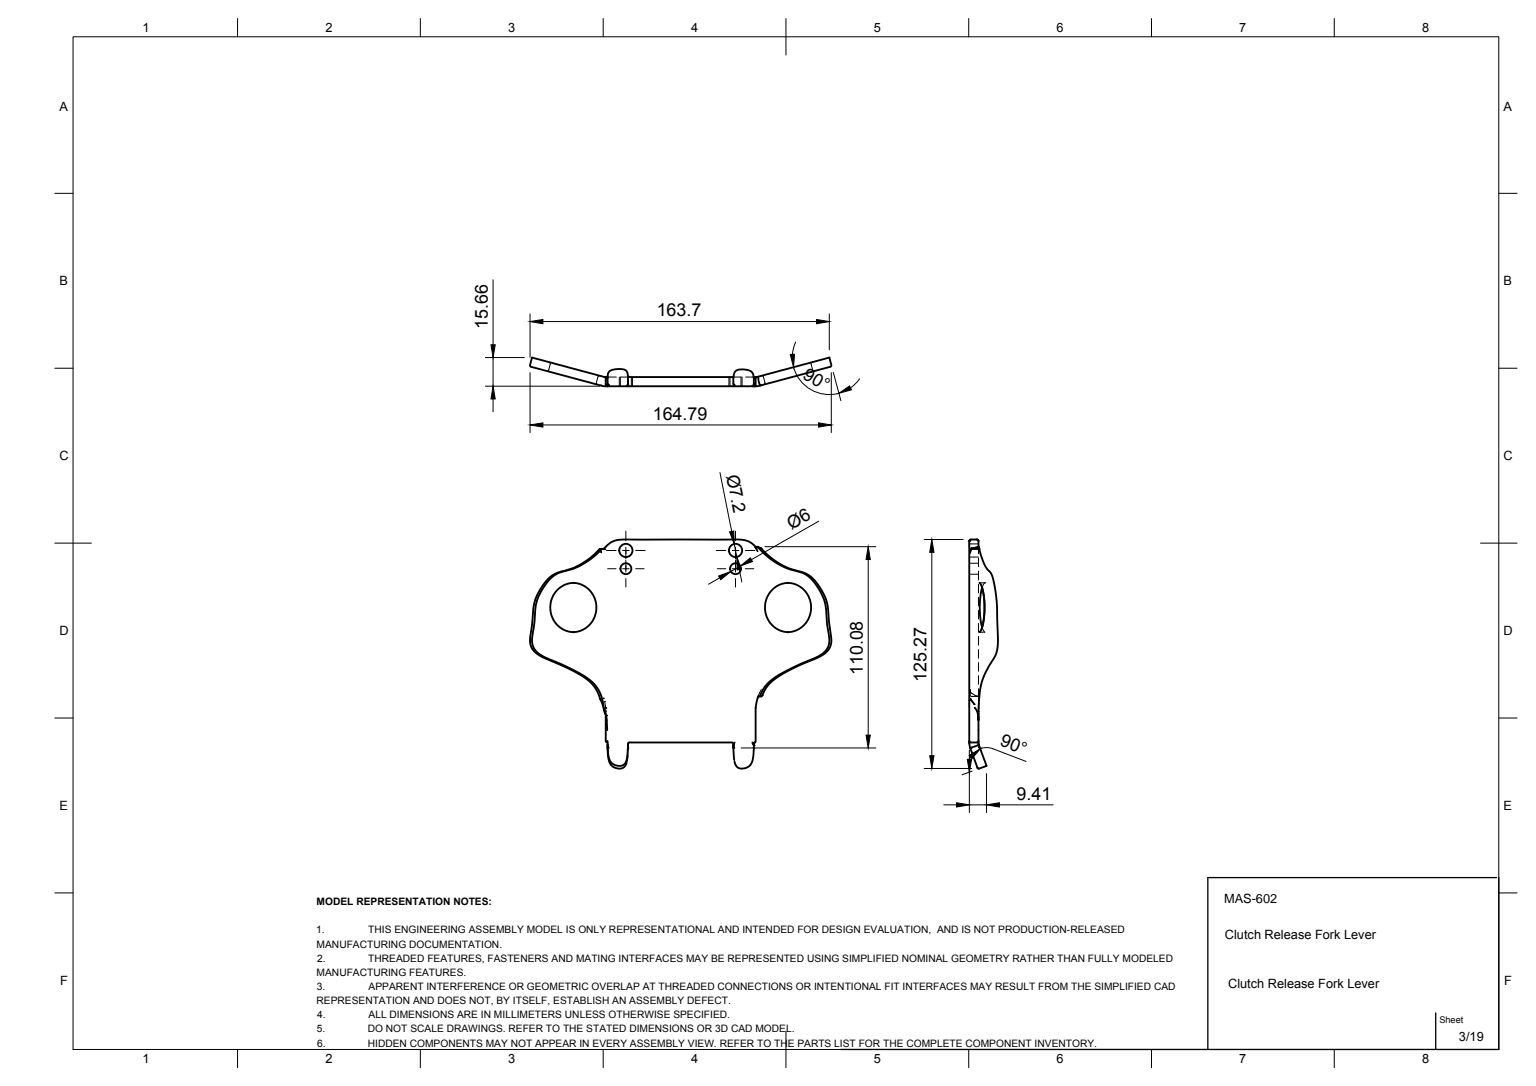
ISO-10303-21;
HEADER;
/* Generated by software containing ST-Developer
 * from STEP Tools, Inc. (www.steptools.com) 
 */

FILE_DESCRIPTION(
/* description */ (''),
/* implementation_level */ '2;1');

FILE_NAME(
/* name */ 'Clutch Release Fork Lever.step',
/* time_stamp */ '2026-10-15T14:42:47-07:00',
/* author */ (''),
/* organization */ (''),
/* preprocessor_version */ 'ST-DEVELOPER v20.2',
/* originating_system */ 'Autodesk Translation Framework v15.15.0.0',
/* authorisation */ '');

FILE_SCHEMA (('AUTOMOTIVE_DESIGN { 1 0 10303 214 3 1 1 }'));
ENDSEC;

DATA;
#10=MECHANICAL_DESIGN_GEOMETRIC_PRESENTATION_REPRESENTATION('',(#234),#85789);
#198=SHAPE_REPRESENTATION_RELATIONSHIP('SRR','None',#85863,#216);
#216=ADVANCED_BREP_SHAPE_REPRESENTATION('',(#252),#85771);
#234=STYLED_ITEM('',(#85962),#252);
#252=MANIFOLD_SOLID_BREP('Body1',#9881);
#270=SPHERICAL_SURFACE('',#10130,0.08);
#271=SPHERICAL_SURFACE('',#10138,0.08);
#272=SPHERICAL_SURFACE('',#10178,0.08);
#273=SPHERICAL_SURFACE('',#10200,0.08);
#274=SPHERICAL_SURFACE('',#10239,0.08);
#275=SPHERICAL_SURFACE('',#10241,0.08);
#276=SPHERICAL_SURFACE('',#10260,0.08);
#277=SPHERICAL_SURFACE('',#10282,0.08);
#278=SPHERICAL_SURFACE('',#10292,0.08);
#280=B_SPLINE_SURFACE_WITH_KNOTS('',3,1,((#13627,#13628),(#13629,#13630),
(#13631,#13632),(#13633,#13634),(#13635,#13636),(#13637,#13638),(#13639,
#13640)),.UNSPECIFIED.,.F.,.F.,.F.,(4,1,1,1,4),(2,2),(0.,0.285714285714286,
0.571428571428571,0.785714285714286,1.),(0.,0.504000000000458),
 .UNSPECIFIED.);
#281=B_SPLINE_SURFACE_WITH_KNOTS('',5,1,((#13700,#13701),(#13702,#13703),
(#13704,#13705),(#13706,#13707),(#13708,#13709),(#13710,#13711),(#13712,
#13713),(#13714,#13715),(#13716,#13717),(#13718,#13719),(#13720,#13721),
(#13722,#13723),(#13724,#13725),(#13726,#13727),(#13728,#13729),(#13730,
#13731),(#13732,#13733),(#13734,#13735),(#13736,#13737),(#13738,#13739),
(#13740,#13741),(#13742,#13743),(#13744,#13745),(#13746,#13747),(#13748,
#13749),(#13750,#13751),(#13752,#13753),(#13754,#13755),(#13756,#13757),
(#13758,#13759),(#13760,#13761),(#13762,#13763),(#13764,#13765),(#13766,
#13767),(#13768,#13769),(#13770,#13771),(#13772,#13773),(#13774,#13775),
(#13776,#13777),(#13778,#13779),(#13780,#13781),(#13782,#13783),(#13784,
#13785),(#13786,#13787),(#13788,#13789),(#13790,#13791),(#13792,#13793),
(#13794,#13795),(#13796,#13797),(#13798,#13799),(#13800,#13801),(#13802,
#13803),(#13804,#13805),(#13806,#13807),(#13808,#13809),(#13810,#13811),
(#13812,#13813),(#13814,#13815),(#13816,#13817),(#13818,#13819),(#13820,
#13821),(#13822,#13823),(#13824,#13825),(#13826,#13827),(#13828,#13829),
(#13830,#13831),(#13832,#13833),(#13834,#13835),(#13836,#13837),(#13838,
#13839),(#13840,#13841),(#13842,#13843),(#13844,#13845),(#13846,#13847),
(#13848,#13849),(#13850,#13851),(#13852,#13853),(#13854,#13855),(#13856,
#13857),(#13858,#13859),(#13860,#13861),(#13862,#13863),(#13864,#13865),
(#13866,#13867),(#13868,#13869),(#13870,#13871),(#13872,#13873),(#13874,
#13875),(#13876,#13877),(#13878,#13879),(#13880,#13881),(#13882,#13883),
(#13884,#13885),(#13886,#13887),(#13888,#13889),(#13890,#13891),(#13892,
#13893),(#13894,#13895),(#13896,#13897),(#13898,#13899),(#13900,#13901),
(#13902,#13903),(#13904,#13905),(#13906,#13907),(#13908,#13909),(#13910,
#13911),(#13912,#13913),(#13914,#13915),(#13916,#13917),(#13918,#13919),
(#13920,#13921),(#13922,#13923),(#13924,#13925),(#13926,#13927),(#13928,
#13929),(#13930,#13931),(#13932,#13933),(#13934,#13935),(#13936,#13937),
(#13938,#13939),(#13940,#13941),(#13942,#13943),(#13944,#13945),(#13946,
#13947),(#13948,#13949),(#13950,#13951),(#13952,#13953),(#13954,#13955),
(#13956,#13957),(#13958,#13959),(#13960,#13961),(#13962,#13963),(#13964,
#13965),(#13966,#13967),(#13968,#13969),(#13970,#13971),(#13972,#13973),
(#13974,#13975),(#13976,#13977),(#13978,#13979),(#13980,#13981),(#13982,
#13983),(#13984,#13985),(#13986,#13987),(#13988,#13989),(#13990,#13991),
(#13992,#13993),(#13994,#13995),(#13996,#13997),(#13998,#13999),(#14000,
#14001),(#14002,#14003),(#14004,#14005),(#14006,#14007),(#14008,#14009),
(#14010,#14011),(#14012,#14013),(#14014,#14015),(#14016,#14017),(#14018,
#14019),(#14020,#14021),(#14022,#14023),(#14024,#14025),(#14026,#14027),
(#14028,#14029),(#14030,#14031),(#14032,#14033),(#14034,#14035),(#14036,
#14037),(#14038,#14039),(#14040,#14041),(#14042,#14043),(#14044,#14045),
(#14046,#14047),(#14048,#14049),(#14050,#14051),(#14052,#14053),(#14054,
#14055),(#14056,#14057),(#14058,#14059),(#14060,#14061),(#14062,#14063),
(#14064,#14065),(#14066,#14067),(#14068,#14069),(#14070,#14071),(#14072,
#14073),(#14074,#14075),(#14076,#14077),(#14078,#14079),(#14080,#14081),
(#14082,#14083),(#14084,#14085),(#14086,#14087),(#14088,#14089),(#14090,
#14091),(#14092,#14093),(#14094,#14095),(#14096,#14097),(#14098,#14099),
(#14100,#14101),(#14102,#14103),(#14104,#14105),(#14106,#14107),(#14108,
#14109),(#14110,#14111),(#14112,#14113),(#14114,#14115),(#14116,#14117),
(#14118,#14119),(#14120,#14121),(#14122,#14123),(#14124,#14125),(#14126,
#14127),(#14128,#14129),(#14130,#14131),(#14132,#14133),(#14134,#14135),
(#14136,#14137),(#14138,#14139),(#14140,#14141),(#14142,#14143),(#14144,
#14145),(#14146,#14147),(#14148,#14149),(#14150,#14151),(#14152,#14153),
(#14154,#14155),(#14156,#14157),(#14158,#14159),(#14160,#14161),(#14162,
#14163),(#14164,#14165),(#14166,#14167),(#14168,#14169),(#14170,#14171),
(#14172,#14173),(#14174,#14175),(#14176,#14177),(#14178,#14179),(#14180,
#14181),(#14182,#14183),(#14184,#14185),(#14186,#14187),(#14188,#14189),
(#14190,#14191),(#14192,#14193),(#14194,#14195),(#14196,#14197),(#14198,
#14199),(#14200,#14201),(#14202,#14203),(#14204,#14205),(#14206,#14207),
(#14208,#14209),(#14210,#14211),(#14212,#14213),(#14214,#14215),(#14216,
#14217),(#14218,#14219)),.UNSPECIFIED.,.T.,.F.,.F.,(6,1,1,1,1,1,1,1,1,1,
1,1,1,1,1,1,1,1,1,1,1,1,1,1,1,1,1,1,1,1,1,1,1,1,1,1,1,1,1,1,1,1,1,1,1,1,
1,1,1,1,1,1,1,1,1,1,1,1,1,1,1,1,1,1,1,1,1,1,1,1,1,1,1,1,1,1,1,1,1,1,5,1,
1,1,1,1,1,1,1,1,1,1,1,1,1,1,1,1,1,1,1,1,1,1,1,1,1,1,1,1,1,1,1,1,1,1,1,1,
1,1,1,1,1,1,1,1,1,1,1,1,1,1,1,1,1,1,1,1,1,1,1,1,1,1,1,1,1,1,1,1,1,1,1,1,
1,1,1,1,1,1,1,1,1,1,1,1,1,1,1,1,1,1,1,1,1,1,1,1,1,1,1,1,1,1,1,1,1,1,1,1,
1,1,1,1,1,1,1,1,1,1,1,1,1,1,1,1,1,1,1,1,1,1,1,1,1,1,1,1,1,1,1,1,1,1,1,1,
1,1,1,1,1,1,1,1,1,1,1,1,1,1,1,1,1,1,1,1,1,1,1,1,1,6),(2,2),(-0.318438690804418,
-0.316,-0.312,-0.308,-0.304,-0.3,-0.296,-0.292,-0.288,-0.284,-0.28,-0.276,
-0.272,-0.268,-0.264,-0.26,-0.256,-0.252,-0.248,-0.244,-0.24,-0.236,-0.232,
-0.228,-0.224,-0.22,-0.216,-0.212,-0.208,-0.204,-0.2,-0.196,-0.192,-0.188,
-0.184,-0.18,-0.176,-0.172,-0.168,-0.164,-0.16,-0.156,-0.152,-0.148,-0.144,
-0.14,-0.136,-0.132,-0.128,-0.124,-0.12,-0.116,-0.112,-0.108,-0.104,-0.1,
-0.0960000000000001,-0.0920000000000001,-0.0880000000000001,-0.084,-0.08,
-0.076,-0.072,-0.068,-0.064,-0.06,-0.056,-0.052,-0.048,-0.044,-0.04,-0.036,
-0.032,-0.028,-0.024,-0.02,-0.016,-0.012,-0.008,-0.004,0.,0.00399999999999923,
0.00799999999999923,0.0119999999999992,0.0159999999999992,0.0199999999999992,
0.0239999999999992,0.0279999999999992,0.0319999999999993,0.0359999999999993,
0.0399999999999993,0.0439999999999993,0.0479999999999993,0.0519999999999993,
0.0559999999999993,0.0599999999999993,0.0639999999999993,0.0679999999999993,
0.0719999999999993,0.0759999999999993,0.0799999999999993,0.0839999999999993,
0.0879999999999993,0.0919999999999993,0.0959999999999993,0.0999999999999993,
0.103999999999999,0.107999999999999,0.111999999999999,0.115999999999999,
0.119999999999999,0.123999999999999,0.127999999999999,0.131999999999999,
0.135999999999999,0.139999999999999,0.143999999999999,0.147999999999999,
0.151999999999999,0.155999999999999,0.159999999999999,0.163999999999999,
0.167999999999999,0.171999999999999,0.175999999999999,0.179999999999999,
0.183999999999999,0.187999999999999,0.191999999999999,0.195999999999999,
0.199999999999999,0.203999999999999,0.207999999999999,0.211999999999999,
0.215999999999999,0.219999999999999,0.223999999999999,0.227999999999999,
0.231999999999999,0.235999999999999,0.239999999999999,0.243999999999999,
0.247999999999999,0.251999999999999,0.255999999999999,0.259999999999999,
0.263999999999999,0.267999999999999,0.271999999999999,0.275999999999999,
0.279999999999999,0.283999999999999,0.287999999999999,0.291999999999999,
0.295999999999999,0.299999999999999,0.303999999999999,0.307999999999999,
0.311999999999999,0.316,0.32,0.324,0.328,0.332,0.336,0.34,0.344,0.348,0.352,
0.356,0.36,0.364,0.368,0.372,0.376,0.38,0.384,0.388,0.392,0.396,0.4,0.404,
0.408,0.412,0.416,0.42,0.424,0.428,0.432,0.436,0.44,0.444,0.448,0.452,0.456,
0.46,0.464,0.468,0.472,0.476,0.48,0.484,0.488,0.492,0.496,0.5,0.504,0.508,
0.512,0.516,0.52,0.524,0.528,0.532,0.536,0.54,0.544,0.548,0.552,0.556,0.56,
0.564,0.568,0.572,0.576,0.58,0.584,0.588,0.592,0.596,0.6,0.604,0.608,0.612,
0.616,0.62,0.624,0.628,0.632,0.636,0.64,0.644,0.648,0.652,0.656,0.66,0.664,
0.668,0.672,0.676,0.68,0.681561309195582),(0.,2.17767906516806),
 .UNSPECIFIED.);
#282=B_SPLINE_SURFACE_WITH_KNOTS('',3,3,((#14275,#14276,#14277,#14278,#14279,
#14280,#14281,#14282,#14283,#14284,#14285,#14286,#14287,#14288,#14289,#14290,
#14291,#14292,#14293,#14294,#14295,#14296,#14297,#14298,#14299,#14300,#14301,
#14302,#14303,#14304,#14305,#14306,#14307,#14308,#14309),(#14310,#14311,
#14312,#14313,#14314,#14315,#14316,#14317,#14318,#14319,#14320,#14321,#14322,
#14323,#14324,#14325,#14326,#14327,#14328,#14329,#14330,#14331,#14332,#14333,
#14334,#14335,#14336,#14337,#14338,#14339,#14340,#14341,#14342,#14343,#14344),
(#14345,#14346,#14347,#14348,#14349,#14350,#14351,#14352,#14353,#14354,
#14355,#14356,#14357,#14358,#14359,#14360,#14361,#14362,#14363,#14364,#14365,
#14366,#14367,#14368,#14369,#14370,#14371,#14372,#14373,#14374,#14375,#14376,
#14377,#14378,#14379),(#14380,#14381,#14382,#14383,#14384,#14385,#14386,
#14387,#14388,#14389,#14390,#14391,#14392,#14393,#14394,#14395,#14396,#14397,
#14398,#14399,#14400,#14401,#14402,#14403,#14404,#14405,#14406,#14407,#14408,
#14409,#14410,#14411,#14412,#14413,#14414),(#14415,#14416,#14417,#14418,
#14419,#14420,#14421,#14422,#14423,#14424,#14425,#14426,#14427,#14428,#14429,
#14430,#14431,#14432,#14433,#14434,#14435,#14436,#14437,#14438,#14439,#14440,
#14441,#14442,#14443,#14444,#14445,#14446,#14447,#14448,#14449)),
 .UNSPECIFIED.,.F.,.F.,.F.,(4,1,4),(4,1,1,1,1,1,1,1,1,1,1,1,1,1,1,1,1,1,
1,1,1,1,1,1,1,1,1,1,1,1,1,1,4),(0.,0.571428571428571,1.),(0.,0.433353360299055,
0.866706720598111,1.30006008089717,1.73341344119622,2.16676680149528,2.49178182171957,
2.60012016179433,3.03347352209339,3.25015020224292,3.46682688239244,4.04463136279118,
4.62243584318992,4.91133808338929,5.20024032358866,5.77804480398741,6.06694704418677,
6.35584928438614,6.64475152458552,6.93365376478489,7.22255600498426,7.36700712508394,
7.51145824518363,7.65590936528331,7.800360485383,8.08926272558237,8.66706720598111,
9.24487168637985,9.82267616677859,10.4004806471773,11.2671873677754,11.7005407280745,
12.1338940883735),.UNSPECIFIED.);
#283=B_SPLINE_SURFACE_WITH_KNOTS('',3,3,((#14451,#14452,#14453,#14454,#14455,
#14456),(#14457,#14458,#14459,#14460,#14461,#14462),(#14463,#14464,#14465,
#14466,#14467,#14468),(#14469,#14470,#14471,#14472,#14473,#14474)),
 .UNSPECIFIED.,.F.,.F.,.F.,(4,4),(4,2,4),(-0.0537574666271907,1.),(-0.15340523472588,
-0.152867184867239,-0.0444303035234761),.UNSPECIFIED.);
#284=B_SPLINE_SURFACE_WITH_KNOTS('',3,3,((#14503,#14504,#14505,#14506),
(#14507,#14508,#14509,#14510),(#14511,#14512,#14513,#14514),(#14515,#14516,
#14517,#14518),(#14519,#14520,#14521,#14522)),.UNSPECIFIED.,.F.,.F.,.F.,
(4,1,4),(4,4),(0.,0.571428571428571,1.),(0.,0.0543233651499556),
 .UNSPECIFIED.);
#285=B_SPLINE_SURFACE_WITH_KNOTS('',3,3,((#14540,#14541,#14542,#14543,#14544,
#14545,#14546,#14547),(#14548,#14549,#14550,#14551,#14552,#14553,#14554,
#14555),(#14556,#14557,#14558,#14559,#14560,#14561,#14562,#14563),(#14564,
#14565,#14566,#14567,#14568,#14569,#14570,#14571),(#14572,#14573,#14574,
#14575,#14576,#14577,#14578,#14579),(#14580,#14581,#14582,#14583,#14584,
#14585,#14586,#14587)),.UNSPECIFIED.,.F.,.F.,.F.,(4,1,1,4),(4,1,1,1,1,4),
(0.,0.285714285714286,0.571428571428571,1.),(0.0937174606900304,0.104785099917186,
0.112163526068624,0.115852739144342,0.117697345682202,0.119541952220061),
 .UNSPECIFIED.);
#286=B_SPLINE_SURFACE_WITH_KNOTS('',3,3,((#14598,#14599,#14600,#14601,#14602,
#14603),(#14604,#14605,#14606,#14607,#14608,#14609),(#14610,#14611,#14612,
#14613,#14614,#14615),(#14616,#14617,#14618,#14619,#14620,#14621),(#14622,
#14623,#14624,#14625,#14626,#14627)),.UNSPECIFIED.,.F.,.F.,.F.,(4,1,4),
(4,1,1,4),(0.362133804475251,0.635505031128715,1.),(1.65498255800438E-15,
0.129082836972258,0.215138061620429,0.3011932862686),.UNSPECIFIED.);
#287=B_SPLINE_SURFACE_WITH_KNOTS('',3,3,((#14636,#14637,#14638,#14639),
(#14640,#14641,#14642,#14643),(#14644,#14645,#14646,#14647),(#14648,#14649,
#14650,#14651),(#14652,#14653,#14654,#14655)),.UNSPECIFIED.,.F.,.F.,.F.,
(4,1,4),(4,4),(-3.21642455285252E-5,0.5,1.),(-3.21642455285252E-5,0.22768259721804),
 .UNSPECIFIED.);
#288=B_SPLINE_SURFACE_WITH_KNOTS('',3,3,((#14667,#14668,#14669,#14670),
(#14671,#14672,#14673,#14674),(#14675,#14676,#14677,#14678),(#14679,#14680,
#14681,#14682),(#14683,#14684,#14685,#14686)),.UNSPECIFIED.,.F.,.F.,.F.,
(4,1,4),(4,4),(0.,0.5,1.),(6.03465648009666E-14,0.0429068684110201),
 .UNSPECIFIED.);
#289=B_SPLINE_SURFACE_WITH_KNOTS('',3,3,((#14693,#14694,#14695,#14696),
(#14697,#14698,#14699,#14700),(#14701,#14702,#14703,#14704),(#14705,#14706,
#14707,#14708),(#14709,#14710,#14711,#14712)),.UNSPECIFIED.,.F.,.F.,.F.,
(4,1,4),(4,4),(0.,0.571428571428571,1.),(0.,0.0979595230969147),
 .UNSPECIFIED.);
#290=B_SPLINE_SURFACE_WITH_KNOTS('',3,3,((#14714,#14715,#14716,#14717),
(#14718,#14719,#14720,#14721),(#14722,#14723,#14724,#14725),(#14726,#14727,
#14728,#14729),(#14730,#14731,#14732,#14733)),.UNSPECIFIED.,.F.,.F.,.F.,
(4,1,4),(4,4),(0.,0.5,1.),(0.101309492239901,0.150948832556605),
 .UNSPECIFIED.);
#291=B_SPLINE_SURFACE_WITH_KNOTS('',3,3,((#14774,#14775,#14776,#14777),
(#14778,#14779,#14780,#14781),(#14782,#14783,#14784,#14785),(#14786,#14787,
#14788,#14789),(#14790,#14791,#14792,#14793)),.UNSPECIFIED.,.F.,.F.,.F.,
(4,1,4),(4,4),(0.362133804475334,0.726628773346571,1.),(0.,0.0965340005117894),
 .UNSPECIFIED.);
#292=B_SPLINE_SURFACE_WITH_KNOTS('',3,3,((#14829,#14830,#14831,#14832),
(#14833,#14834,#14835,#14836),(#14837,#14838,#14839,#14840),(#14841,#14842,
#14843,#14844),(#14845,#14846,#14847,#14848)),.UNSPECIFIED.,.F.,.F.,.F.,
(4,1,4),(4,4),(0.40963181845835,0.704815909229175,1.),(0.,0.224615521635083),
 .UNSPECIFIED.);
#293=B_SPLINE_SURFACE_WITH_KNOTS('',3,3,((#14855,#14856,#14857,#14858),
(#14859,#14860,#14861,#14862),(#14863,#14864,#14865,#14866),(#14867,#14868,
#14869,#14870),(#14871,#14872,#14873,#14874)),.UNSPECIFIED.,.F.,.F.,.F.,
(4,1,4),(4,4),(0.,0.23767239441161,0.47534478882322),(0.0854459382956349,
0.127798241063314),.UNSPECIFIED.);
#294=B_SPLINE_SURFACE_WITH_KNOTS('',3,3,((#14881,#14882,#14883,#14884,#14885,
#14886,#14887),(#14888,#14889,#14890,#14891,#14892,#14893,#14894),(#14895,
#14896,#14897,#14898,#14899,#14900,#14901),(#14902,#14903,#14904,#14905,
#14906,#14907,#14908),(#14909,#14910,#14911,#14912,#14913,#14914,#14915),
(#14916,#14917,#14918,#14919,#14920,#14921,#14922)),.UNSPECIFIED.,.F.,.F.,
 .F.,(4,1,1,4),(4,1,1,1,4),(0.283162399774082,0.590378514156618,0.795189257078309,
1.),(0.,0.0328013253035665,0.065602650607133,0.109337751011888,0.153072851416644),
 .UNSPECIFIED.);
#295=B_SPLINE_SURFACE_WITH_KNOTS('',3,3,((#14931,#14932,#14933,#14934),
(#14935,#14936,#14937,#14938),(#14939,#14940,#14941,#14942),(#14943,#14944,
#14945,#14946),(#14947,#14948,#14949,#14950)),.UNSPECIFIED.,.F.,.F.,.F.,
(4,1,4),(4,4),(0.44925085787876,0.702584769501779,0.955918681124799),(0.,
0.0419417607304844),.UNSPECIFIED.);
#296=B_SPLINE_SURFACE_WITH_KNOTS('',3,3,((#14951,#14952,#14953,#14954),
(#14955,#14956,#14957,#14958),(#14959,#14960,#14961,#14962),(#14963,#14964,
#14965,#14966)),.UNSPECIFIED.,.F.,.F.,.F.,(4,4),(4,4),(0.,0.279727981322212),
(0.,0.17884239607127),.UNSPECIFIED.);
#297=B_SPLINE_SURFACE_WITH_KNOTS('',3,3,((#14973,#14974,#14975,#14976),
(#14977,#14978,#14979,#14980),(#14981,#14982,#14983,#14984),(#14985,#14986,
#14987,#14988)),.UNSPECIFIED.,.F.,.F.,.F.,(4,4),(4,4),(0.547578918945948,
1.),(0.,0.0801298062963358),.UNSPECIFIED.);
#298=B_SPLINE_SURFACE_WITH_KNOTS('',3,3,((#14995,#14996,#14997,#14998,#14999,
#15000,#15001,#15002,#15003,#15004,#15005,#15006,#15007,#15008,#15009,#15010,
#15011,#15012,#15013,#15014,#15015),(#15016,#15017,#15018,#15019,#15020,
#15021,#15022,#15023,#15024,#15025,#15026,#15027,#15028,#15029,#15030,#15031,
#15032,#15033,#15034,#15035,#15036),(#15037,#15038,#15039,#15040,#15041,
#15042,#15043,#15044,#15045,#15046,#15047,#15048,#15049,#15050,#15051,#15052,
#15053,#15054,#15055,#15056,#15057),(#15058,#15059,#15060,#15061,#15062,
#15063,#15064,#15065,#15066,#15067,#15068,#15069,#15070,#15071,#15072,#15073,
#15074,#15075,#15076,#15077,#15078),(#15079,#15080,#15081,#15082,#15083,
#15084,#15085,#15086,#15087,#15088,#15089,#15090,#15091,#15092,#15093,#15094,
#15095,#15096,#15097,#15098,#15099)),.UNSPECIFIED.,.F.,.F.,.F.,(4,1,4),
(4,1,1,1,1,1,1,1,1,1,1,1,1,1,1,1,1,1,4),(0.,0.571428571428571,1.),(0.,0.148302061038192,
0.296604122076384,0.444906183114576,0.593208244152767,0.889812366229151,
1.18641648830553,1.7796247324583,2.37283297661107,4.74566595322214,5.93208244152767,
6.52529068568044,7.11849892983321,7.41510305190959,7.71170717398598,7.86000923502417,
8.00831129606236,8.15661335710055,8.30491541813874),.UNSPECIFIED.);
#299=B_SPLINE_SURFACE_WITH_KNOTS('',5,1,((#15347,#15348),(#15349,#15350),
(#15351,#15352),(#15353,#15354),(#15355,#15356),(#15357,#15358),(#15359,
#15360),(#15361,#15362),(#15363,#15364),(#15365,#15366),(#15367,#15368),
(#15369,#15370),(#15371,#15372),(#15373,#15374),(#15375,#15376),(#15377,
#15378),(#15379,#15380),(#15381,#15382),(#15383,#15384),(#15385,#15386),
(#15387,#15388),(#15389,#15390),(#15391,#15392),(#15393,#15394),(#15395,
#15396),(#15397,#15398),(#15399,#15400),(#15401,#15402),(#15403,#15404),
(#15405,#15406),(#15407,#15408),(#15409,#15410),(#15411,#15412),(#15413,
#15414),(#15415,#15416),(#15417,#15418),(#15419,#15420),(#15421,#15422),
(#15423,#15424),(#15425,#15426),(#15427,#15428)),.UNSPECIFIED.,.F.,.F.,
 .F.,(6,1,1,1,1,1,1,1,1,1,1,1,1,1,1,1,5,1,1,1,1,1,1,1,1,1,1,1,1,1,1,1,6),
(2,2),(-1.06140995878253,-1.06,-1.056,-1.052,-1.048,-1.044,-1.04,-1.036,
-1.032,-1.028,-1.024,-1.02,-1.016,-1.012,-1.008,-1.004,-1.,-0.996000000000001,
-0.992000000000001,-0.988000000000001,-0.984000000000001,-0.980000000000001,
-0.976000000000001,-0.972000000000001,-0.968000000000001,-0.964000000000001,
-0.960000000000001,-0.956000000000001,-0.952000000000001,-0.948000000000001,
-0.944000000000001,-0.940000000000001,-0.938590041217474),(0.,0.6),
 .UNSPECIFIED.);
#300=B_SPLINE_SURFACE_WITH_KNOTS('',5,1,((#15656,#15657),(#15658,#15659),
(#15660,#15661),(#15662,#15663),(#15664,#15665),(#15666,#15667),(#15668,
#15669),(#15670,#15671),(#15672,#15673),(#15674,#15675),(#15676,#15677),
(#15678,#15679),(#15680,#15681),(#15682,#15683),(#15684,#15685),(#15686,
#15687),(#15688,#15689),(#15690,#15691),(#15692,#15693),(#15694,#15695),
(#15696,#15697),(#15698,#15699),(#15700,#15701),(#15702,#15703),(#15704,
#15705),(#15706,#15707),(#15708,#15709),(#15710,#15711),(#15712,#15713),
(#15714,#15715),(#15716,#15717),(#15718,#15719),(#15720,#15721),(#15722,
#15723),(#15724,#15725),(#15726,#15727),(#15728,#15729),(#15730,#15731),
(#15732,#15733),(#15734,#15735),(#15736,#15737),(#15738,#15739),(#15740,
#15741),(#15742,#15743),(#15744,#15745),(#15746,#15747),(#15748,#15749),
(#15750,#15751),(#15752,#15753),(#15754,#15755),(#15756,#15757),(#15758,
#15759),(#15760,#15761),(#15762,#15763),(#15764,#15765),(#15766,#15767),
(#15768,#15769),(#15770,#15771),(#15772,#15773),(#15774,#15775),(#15776,
#15777),(#15778,#15779),(#15780,#15781),(#15782,#15783),(#15784,#15785),
(#15786,#15787),(#15788,#15789),(#15790,#15791),(#15792,#15793),(#15794,
#15795)),.UNSPECIFIED.,.F.,.F.,.F.,(6,1,1,1,1,1,1,1,1,1,1,1,1,1,1,1,1,1,
1,1,1,1,1,1,1,1,1,1,1,1,1,1,1,1,1,1,1,1,1,1,1,1,1,1,1,1,1,1,1,1,1,1,1,1,
1,1,1,1,1,1,1,1,1,1,1,6),(2,2),(-0.318438690804418,-0.316,-0.312,-0.308,
-0.304,-0.3,-0.296,-0.292,-0.288,-0.284,-0.28,-0.276,-0.272,-0.268,-0.264,
-0.26,-0.256,-0.252,-0.248,-0.244,-0.24,-0.236,-0.232,-0.228,-0.224,-0.22,
-0.216,-0.212,-0.208,-0.204,-0.2,-0.196,-0.192,-0.188,-0.184,-0.18,-0.176,
-0.172,-0.168,-0.164,-0.16,-0.156,-0.152,-0.148,-0.144,-0.14,-0.136,-0.132,
-0.128,-0.124,-0.12,-0.116,-0.112,-0.108,-0.104,-0.1,-0.0960000000000001,
-0.0920000000000001,-0.0880000000000001,-0.084,-0.08,-0.076,-0.072,-0.068,
-0.064,-0.0614099587825327),(0.,7.2),.UNSPECIFIED.);
#301=B_SPLINE_SURFACE_WITH_KNOTS('',3,3,((#15802,#15803,#15804,#15805,#15806,
#15807),(#15808,#15809,#15810,#15811,#15812,#15813),(#15814,#15815,#15816,
#15817,#15818,#15819),(#15820,#15821,#15822,#15823,#15824,#15825)),
 .UNSPECIFIED.,.F.,.F.,.F.,(4,4),(4,1,1,4),(-4.4838175058205E-5,1.),(-0.140841580089521,
-0.0804552810939789,-0.0402276405469894,4.34253766641143E-5),
 .UNSPECIFIED.);
#302=B_SPLINE_SURFACE_WITH_KNOTS('',3,3,((#15860,#15861,#15862,#15863),
(#15864,#15865,#15866,#15867),(#15868,#15869,#15870,#15871),(#15872,#15873,
#15874,#15875)),.UNSPECIFIED.,.F.,.F.,.F.,(4,4),(4,4),(0.,1.),(-0.0800719510115295,
0.),.UNSPECIFIED.);
#303=B_SPLINE_SURFACE_WITH_KNOTS('',3,3,((#15884,#15885,#15886,#15887,#15888,
#15889),(#15890,#15891,#15892,#15893,#15894,#15895),(#15896,#15897,#15898,
#15899,#15900,#15901),(#15902,#15903,#15904,#15905,#15906,#15907)),
 .UNSPECIFIED.,.F.,.F.,.F.,(4,4),(4,2,4),(0.,1.),(0.148045073228805,0.168188087897107,
0.168704904027193),.UNSPECIFIED.);
#304=B_SPLINE_SURFACE_WITH_KNOTS('',3,3,((#15911,#15912,#15913,#15914),
(#15915,#15916,#15917,#15918),(#15919,#15920,#15921,#15922),(#15923,#15924,
#15925,#15926)),.UNSPECIFIED.,.F.,.F.,.F.,(4,4),(4,4),(0.,1.),(-0.0911290973321825,
-0.0858168351305703),.UNSPECIFIED.);
#305=B_SPLINE_SURFACE_WITH_KNOTS('',3,3,((#15932,#15933,#15934,#15935),
(#15936,#15937,#15938,#15939),(#15940,#15941,#15942,#15943),(#15944,#15945,
#15946,#15947)),.UNSPECIFIED.,.F.,.F.,.F.,(4,4),(4,4),(0.,1.),(0.00872869968615488,
0.428984955288124),.UNSPECIFIED.);
#306=B_SPLINE_SURFACE_WITH_KNOTS('',3,3,((#15962,#15963,#15964,#15965,#15966,
#15967,#15968,#15969),(#15970,#15971,#15972,#15973,#15974,#15975,#15976,
#15977),(#15978,#15979,#15980,#15981,#15982,#15983,#15984,#15985),(#15986,
#15987,#15988,#15989,#15990,#15991,#15992,#15993),(#15994,#15995,#15996,
#15997,#15998,#15999,#16000,#16001)),.UNSPECIFIED.,.F.,.F.,.F.,(4,1,4),
(4,1,1,1,1,4),(0.,0.5,1.),(-0.288406861392734,-0.268681894462045,-0.248956927531355,
-0.209506993669976,-0.170057059808597,-0.01225732436308),.UNSPECIFIED.);
#307=B_SPLINE_SURFACE_WITH_KNOTS('',5,1,((#16074,#16075),(#16076,#16077),
(#16078,#16079),(#16080,#16081),(#16082,#16083),(#16084,#16085),(#16086,
#16087),(#16088,#16089),(#16090,#16091),(#16092,#16093),(#16094,#16095),
(#16096,#16097),(#16098,#16099),(#16100,#16101),(#16102,#16103),(#16104,
#16105),(#16106,#16107),(#16108,#16109),(#16110,#16111),(#16112,#16113),
(#16114,#16115),(#16116,#16117),(#16118,#16119),(#16120,#16121),(#16122,
#16123),(#16124,#16125),(#16126,#16127),(#16128,#16129),(#16130,#16131),
(#16132,#16133),(#16134,#16135),(#16136,#16137),(#16138,#16139),(#16140,
#16141),(#16142,#16143),(#16144,#16145),(#16146,#16147),(#16148,#16149),
(#16150,#16151),(#16152,#16153),(#16154,#16155),(#16156,#16157),(#16158,
#16159),(#16160,#16161),(#16162,#16163),(#16164,#16165),(#16166,#16167),
(#16168,#16169),(#16170,#16171),(#16172,#16173),(#16174,#16175),(#16176,
#16177),(#16178,#16179),(#16180,#16181),(#16182,#16183),(#16184,#16185),
(#16186,#16187),(#16188,#16189),(#16190,#16191),(#16192,#16193),(#16194,
#16195),(#16196,#16197),(#16198,#16199),(#16200,#16201),(#16202,#16203),
(#16204,#16205),(#16206,#16207),(#16208,#16209),(#16210,#16211),(#16212,
#16213),(#16214,#16215),(#16216,#16217),(#16218,#16219),(#16220,#16221),
(#16222,#16223),(#16224,#16225),(#16226,#16227),(#16228,#16229),(#16230,
#16231),(#16232,#16233),(#16234,#16235),(#16236,#16237),(#16238,#16239),
(#16240,#16241),(#16242,#16243),(#16244,#16245),(#16246,#16247),(#16248,
#16249),(#16250,#16251),(#16252,#16253),(#16254,#16255),(#16256,#16257),
(#16258,#16259),(#16260,#16261),(#16262,#16263),(#16264,#16265),(#16266,
#16267),(#16268,#16269),(#16270,#16271),(#16272,#16273),(#16274,#16275),
(#16276,#16277),(#16278,#16279),(#16280,#16281),(#16282,#16283),(#16284,
#16285),(#16286,#16287),(#16288,#16289),(#16290,#16291),(#16292,#16293),
(#16294,#16295),(#16296,#16297),(#16298,#16299),(#16300,#16301),(#16302,
#16303),(#16304,#16305),(#16306,#16307),(#16308,#16309),(#16310,#16311),
(#16312,#16313),(#16314,#16315),(#16316,#16317),(#16318,#16319),(#16320,
#16321),(#16322,#16323),(#16324,#16325),(#16326,#16327),(#16328,#16329),
(#16330,#16331),(#16332,#16333),(#16334,#16335),(#16336,#16337),(#16338,
#16339),(#16340,#16341),(#16342,#16343),(#16344,#16345),(#16346,#16347),
(#16348,#16349),(#16350,#16351),(#16352,#16353),(#16354,#16355),(#16356,
#16357),(#16358,#16359),(#16360,#16361),(#16362,#16363),(#16364,#16365),
(#16366,#16367),(#16368,#16369),(#16370,#16371),(#16372,#16373),(#16374,
#16375),(#16376,#16377),(#16378,#16379),(#16380,#16381),(#16382,#16383),
(#16384,#16385),(#16386,#16387),(#16388,#16389),(#16390,#16391),(#16392,
#16393),(#16394,#16395),(#16396,#16397),(#16398,#16399),(#16400,#16401),
(#16402,#16403),(#16404,#16405),(#16406,#16407),(#16408,#16409),(#16410,
#16411),(#16412,#16413),(#16414,#16415),(#16416,#16417),(#16418,#16419),
(#16420,#16421),(#16422,#16423),(#16424,#16425),(#16426,#16427),(#16428,
#16429),(#16430,#16431),(#16432,#16433),(#16434,#16435),(#16436,#16437),
(#16438,#16439),(#16440,#16441),(#16442,#16443),(#16444,#16445),(#16446,
#16447),(#16448,#16449),(#16450,#16451),(#16452,#16453),(#16454,#16455),
(#16456,#16457),(#16458,#16459),(#16460,#16461),(#16462,#16463),(#16464,
#16465),(#16466,#16467),(#16468,#16469),(#16470,#16471),(#16472,#16473),
(#16474,#16475),(#16476,#16477),(#16478,#16479),(#16480,#16481),(#16482,
#16483),(#16484,#16485),(#16486,#16487),(#16488,#16489),(#16490,#16491),
(#16492,#16493),(#16494,#16495),(#16496,#16497),(#16498,#16499),(#16500,
#16501),(#16502,#16503),(#16504,#16505),(#16506,#16507),(#16508,#16509),
(#16510,#16511),(#16512,#16513),(#16514,#16515),(#16516,#16517),(#16518,
#16519),(#16520,#16521),(#16522,#16523),(#16524,#16525),(#16526,#16527),
(#16528,#16529),(#16530,#16531),(#16532,#16533),(#16534,#16535),(#16536,
#16537),(#16538,#16539),(#16540,#16541),(#16542,#16543),(#16544,#16545),
(#16546,#16547),(#16548,#16549),(#16550,#16551),(#16552,#16553),(#16554,
#16555),(#16556,#16557),(#16558,#16559),(#16560,#16561),(#16562,#16563),
(#16564,#16565),(#16566,#16567),(#16568,#16569),(#16570,#16571),(#16572,
#16573),(#16574,#16575),(#16576,#16577),(#16578,#16579),(#16580,#16581),
(#16582,#16583),(#16584,#16585),(#16586,#16587),(#16588,#16589),(#16590,
#16591),(#16592,#16593)),.UNSPECIFIED.,.T.,.F.,.F.,(6,1,1,1,1,1,1,1,1,1,
1,1,1,1,1,1,1,1,1,1,1,1,1,1,1,1,1,1,1,1,1,1,1,1,1,1,1,1,1,1,1,1,1,1,1,1,
1,1,1,1,1,1,1,1,1,1,1,1,1,1,1,1,1,1,1,1,1,1,1,1,1,1,1,1,1,1,1,1,1,1,1,1,
1,1,1,1,1,1,1,1,1,1,1,1,1,1,1,1,1,1,1,1,1,1,1,1,1,1,1,1,1,1,1,1,1,1,1,1,
1,1,1,1,1,1,1,1,1,1,1,1,1,1,1,1,1,1,1,1,1,1,1,1,1,1,1,1,1,1,1,1,1,1,1,1,
1,1,1,1,1,1,1,1,1,1,5,1,1,1,1,1,1,1,1,1,1,1,1,1,1,1,1,1,1,1,1,1,1,1,1,1,
1,1,1,1,1,1,1,1,1,1,1,1,1,1,1,1,1,1,1,1,1,1,1,1,1,1,1,1,1,1,1,1,1,1,1,1,
1,1,1,1,1,1,1,1,1,1,1,1,1,1,1,1,1,1,1,1,1,1,1,1,1,6),(2,2),(-0.652913544304935,
-0.652,-0.648,-0.644,-0.64,-0.636,-0.632,-0.628,-0.624,-0.62,-0.616,-0.612,
-0.608,-0.604,-0.6,-0.596,-0.592,-0.588,-0.584,-0.58,-0.576,-0.572,-0.568,
-0.564,-0.56,-0.556,-0.552,-0.548,-0.544,-0.54,-0.536,-0.532,-0.528,-0.524,
-0.52,-0.516,-0.512,-0.508,-0.504,-0.5,-0.496,-0.492,-0.488,-0.484,-0.48,
-0.476,-0.472,-0.468,-0.464,-0.46,-0.456,-0.452,-0.448,-0.444,-0.44,-0.436,
-0.432,-0.428,-0.424,-0.42,-0.416,-0.412,-0.408,-0.404,-0.4,-0.396,-0.392,
-0.388,-0.384,-0.38,-0.376,-0.372,-0.368,-0.364,-0.36,-0.356,-0.352,-0.348,
-0.344,-0.34,-0.336,-0.332,-0.328,-0.324,-0.32,-0.316,-0.312,-0.308,-0.304,
-0.3,-0.296,-0.292,-0.288,-0.284,-0.28,-0.276,-0.272,-0.268,-0.264,-0.26,
-0.256,-0.252,-0.248,-0.244,-0.24,-0.236,-0.232,-0.228,-0.224,-0.22,-0.216,
-0.212,-0.208,-0.204,-0.2,-0.196,-0.192,-0.188,-0.184,-0.18,-0.176,-0.172,
-0.168,-0.164,-0.16,-0.156,-0.152,-0.148,-0.144,-0.14,-0.136,-0.132,-0.128,
-0.124,-0.12,-0.116,-0.112,-0.108,-0.104,-0.1,-0.0960000000000001,-0.0920000000000001,
-0.0880000000000001,-0.084,-0.08,-0.076,-0.072,-0.068,-0.064,-0.06,-0.056,
-0.052,-0.048,-0.044,-0.04,-0.036,-0.032,-0.028,-0.024,-0.02,-0.016,-0.012,
-0.008,-0.004,0.,0.00399999999999923,0.00799999999999923,0.0119999999999992,
0.0159999999999992,0.0199999999999992,0.0239999999999992,0.0279999999999992,
0.0319999999999993,0.0359999999999993,0.0399999999999993,0.0439999999999993,
0.0479999999999993,0.0519999999999993,0.0559999999999993,0.0599999999999993,
0.0639999999999993,0.0679999999999993,0.0719999999999993,0.0759999999999993,
0.0799999999999993,0.0839999999999993,0.0879999999999993,0.0919999999999993,
0.0959999999999993,0.0999999999999993,0.103999999999999,0.107999999999999,
0.111999999999999,0.115999999999999,0.119999999999999,0.123999999999999,
0.127999999999999,0.131999999999999,0.135999999999999,0.139999999999999,
0.143999999999999,0.147999999999999,0.151999999999999,0.155999999999999,
0.159999999999999,0.163999999999999,0.167999999999999,0.171999999999999,
0.175999999999999,0.179999999999999,0.183999999999999,0.187999999999999,
0.191999999999999,0.195999999999999,0.199999999999999,0.203999999999999,
0.207999999999999,0.211999999999999,0.215999999999999,0.219999999999999,
0.223999999999999,0.227999999999999,0.231999999999999,0.235999999999999,
0.239999999999999,0.243999999999999,0.247999999999999,0.251999999999999,
0.255999999999999,0.259999999999999,0.263999999999999,0.267999999999999,
0.271999999999999,0.275999999999999,0.279999999999999,0.283999999999999,
0.287999999999999,0.291999999999999,0.295999999999999,0.299999999999999,
0.303999999999999,0.307999999999999,0.311999999999999,0.316,0.32,0.324,
0.328,0.332,0.336,0.34,0.344,0.347086455695065),(0.,1.0992),
 .UNSPECIFIED.);
#308=B_SPLINE_SURFACE_WITH_KNOTS('',3,3,((#16651,#16652,#16653,#16654,#16655,
#16656,#16657,#16658,#16659,#16660,#16661,#16662,#16663,#16664,#16665,#16666,
#16667,#16668,#16669),(#16670,#16671,#16672,#16673,#16674,#16675,#16676,
#16677,#16678,#16679,#16680,#16681,#16682,#16683,#16684,#16685,#16686,#16687,
#16688),(#16689,#16690,#16691,#16692,#16693,#16694,#16695,#16696,#16697,
#16698,#16699,#16700,#16701,#16702,#16703,#16704,#16705,#16706,#16707),
(#16708,#16709,#16710,#16711,#16712,#16713,#16714,#16715,#16716,#16717,
#16718,#16719,#16720,#16721,#16722,#16723,#16724,#16725,#16726),(#16727,
#16728,#16729,#16730,#16731,#16732,#16733,#16734,#16735,#16736,#16737,#16738,
#16739,#16740,#16741,#16742,#16743,#16744,#16745)),.UNSPECIFIED.,.F.,.F.,
 .F.,(4,1,4),(4,1,1,1,1,1,1,1,1,1,1,1,1,1,1,1,4),(0.,0.571428571428571,
1.),(0.,0.393620506063259,0.787241012126518,0.918447847480938,1.01685297399675,
1.04965468283536,1.11525810051257,1.18086151818978,1.3120683535442,1.44327518889862,
1.57448202425304,1.67288715076885,1.77129227728467,1.96810253031629,2.16491278334792,
2.36172303637955,2.75534354244281),.UNSPECIFIED.);
#309=B_SPLINE_SURFACE_WITH_KNOTS('',3,3,((#16940,#16941,#16942,#16943,#16944),
(#16945,#16946,#16947,#16948,#16949),(#16950,#16951,#16952,#16953,#16954),
(#16955,#16956,#16957,#16958,#16959),(#16960,#16961,#16962,#16963,#16964)),
 .UNSPECIFIED.,.F.,.F.,.F.,(4,1,4),(4,1,4),(0.,0.571428571428571,1.),(-0.166725339205234,
-0.0833626696026172,0.),.UNSPECIFIED.);
#310=B_SPLINE_SURFACE_WITH_KNOTS('',3,3,((#16977,#16978,#16979,#16980),
(#16981,#16982,#16983,#16984),(#16985,#16986,#16987,#16988),(#16989,#16990,
#16991,#16992),(#16993,#16994,#16995,#16996)),.UNSPECIFIED.,.F.,.F.,.F.,
(4,1,4),(4,4),(0.,0.571428571428571,1.),(0.,0.164730944371734),
 .UNSPECIFIED.);
#311=B_SPLINE_SURFACE_WITH_KNOTS('',3,3,((#17011,#17012,#17013,#17014),
(#17015,#17016,#17017,#17018),(#17019,#17020,#17021,#17022),(#17023,#17024,
#17025,#17026),(#17027,#17028,#17029,#17030)),.UNSPECIFIED.,.F.,.F.,.F.,
(4,1,4),(4,4),(0.,0.571428571428571,1.),(0.,0.0505769327849995),
 .UNSPECIFIED.);
#312=B_SPLINE_SURFACE_WITH_KNOTS('',3,3,((#17042,#17043,#17044,#17045),
(#17046,#17047,#17048,#17049),(#17050,#17051,#17052,#17053),(#17054,#17055,
#17056,#17057),(#17058,#17059,#17060,#17061)),.UNSPECIFIED.,.F.,.F.,.F.,
(4,1,4),(4,4),(0.,0.571428571428571,1.),(0.,0.075415368178403),
 .UNSPECIFIED.);
#313=B_SPLINE_SURFACE_WITH_KNOTS('',3,3,((#17070,#17071,#17072,#17073),
(#17074,#17075,#17076,#17077),(#17078,#17079,#17080,#17081),(#17082,#17083,
#17084,#17085),(#17086,#17087,#17088,#17089)),.UNSPECIFIED.,.F.,.F.,.F.,
(4,1,4),(4,4),(0.,0.571428571428571,1.),(0.,0.0172305871960441),
 .UNSPECIFIED.);
#314=B_SPLINE_SURFACE_WITH_KNOTS('',5,1,((#17098,#17099),(#17100,#17101),
(#17102,#17103),(#17104,#17105),(#17106,#17107),(#17108,#17109),(#17110,
#17111),(#17112,#17113),(#17114,#17115),(#17116,#17117),(#17118,#17119),
(#17120,#17121),(#17122,#17123),(#17124,#17125),(#17126,#17127),(#17128,
#17129),(#17130,#17131),(#17132,#17133),(#17134,#17135),(#17136,#17137),
(#17138,#17139),(#17140,#17141),(#17142,#17143),(#17144,#17145)),
 .UNSPECIFIED.,.F.,.F.,.F.,(6,1,1,1,1,1,1,1,1,1,1,1,1,1,1,1,1,1,1,6),(2,
2),(-0.648016352593037,-0.648,-0.644,-0.64,-0.636,-0.632,-0.628,-0.624,
-0.62,-0.616,-0.612,-0.608,-0.604,-0.6,-0.596,-0.592,-0.588,-0.584,-0.58,
-0.578213301303361),(0.,0.600000000000007),.UNSPECIFIED.);
#315=B_SPLINE_SURFACE_WITH_KNOTS('',3,3,((#17175,#17176,#17177,#17178),
(#17179,#17180,#17181,#17182),(#17183,#17184,#17185,#17186),(#17187,#17188,
#17189,#17190)),.UNSPECIFIED.,.F.,.F.,.F.,(4,4),(4,4),(0.,1.),(0.0795665830105256,
0.50017173665434),.UNSPECIFIED.);
#316=B_SPLINE_SURFACE_WITH_KNOTS('',3,3,((#17204,#17205,#17206,#17207),
(#17208,#17209,#17210,#17211),(#17212,#17213,#17214,#17215),(#17216,#17217,
#17218,#17219)),.UNSPECIFIED.,.F.,.F.,.F.,(4,4),(4,4),(0.301693544058951,
1.00002749346625),(0.119480684281991,0.541502145499565),.UNSPECIFIED.);
#317=B_SPLINE_SURFACE_WITH_KNOTS('',5,1,((#17232,#17233),(#17234,#17235),
(#17236,#17237),(#17238,#17239),(#17240,#17241),(#17242,#17243),(#17244,
#17245),(#17246,#17247),(#17248,#17249),(#17250,#17251),(#17252,#17253),
(#17254,#17255),(#17256,#17257),(#17258,#17259),(#17260,#17261),(#17262,
#17263),(#17264,#17265),(#17266,#17267),(#17268,#17269),(#17270,#17271),
(#17272,#17273),(#17274,#17275),(#17276,#17277),(#17278,#17279),(#17280,
#17281),(#17282,#17283),(#17284,#17285),(#17286,#17287),(#17288,#17289),
(#17290,#17291),(#17292,#17293),(#17294,#17295),(#17296,#17297),(#17298,
#17299),(#17300,#17301),(#17302,#17303),(#17304,#17305),(#17306,#17307),
(#17308,#17309),(#17310,#17311),(#17312,#17313),(#17314,#17315),(#17316,
#17317),(#17318,#17319),(#17320,#17321),(#17322,#17323),(#17324,#17325),
(#17326,#17327),(#17328,#17329),(#17330,#17331),(#17332,#17333),(#17334,
#17335),(#17336,#17337),(#17338,#17339),(#17340,#17341),(#17342,#17343),
(#17344,#17345),(#17346,#17347),(#17348,#17349),(#17350,#17351),(#17352,
#17353),(#17354,#17355),(#17356,#17357),(#17358,#17359),(#17360,#17361),
(#17362,#17363),(#17364,#17365),(#17366,#17367),(#17368,#17369),(#17370,
#17371),(#17372,#17373),(#17374,#17375),(#17376,#17377),(#17378,#17379),
(#17380,#17381),(#17382,#17383),(#17384,#17385),(#17386,#17387),(#17388,
#17389),(#17390,#17391),(#17392,#17393),(#17394,#17395),(#17396,#17397),
(#17398,#17399),(#17400,#17401),(#17402,#17403),(#17404,#17405),(#17406,
#17407),(#17408,#17409),(#17410,#17411),(#17412,#17413),(#17414,#17415),
(#17416,#17417),(#17418,#17419),(#17420,#17421),(#17422,#17423),(#17424,
#17425),(#17426,#17427),(#17428,#17429),(#17430,#17431),(#17432,#17433),
(#17434,#17435),(#17436,#17437),(#17438,#17439),(#17440,#17441),(#17442,
#17443),(#17444,#17445),(#17446,#17447),(#17448,#17449),(#17450,#17451),
(#17452,#17453),(#17454,#17455),(#17456,#17457),(#17458,#17459),(#17460,
#17461),(#17462,#17463),(#17464,#17465),(#17466,#17467),(#17468,#17469),
(#17470,#17471),(#17472,#17473),(#17474,#17475),(#17476,#17477),(#17478,
#17479),(#17480,#17481),(#17482,#17483),(#17484,#17485),(#17486,#17487),
(#17488,#17489),(#17490,#17491),(#17492,#17493),(#17494,#17495),(#17496,
#17497),(#17498,#17499),(#17500,#17501),(#17502,#17503),(#17504,#17505),
(#17506,#17507),(#17508,#17509),(#17510,#17511),(#17512,#17513),(#17514,
#17515),(#17516,#17517),(#17518,#17519),(#17520,#17521),(#17522,#17523),
(#17524,#17525),(#17526,#17527),(#17528,#17529),(#17530,#17531),(#17532,
#17533),(#17534,#17535),(#17536,#17537),(#17538,#17539),(#17540,#17541),
(#17542,#17543),(#17544,#17545),(#17546,#17547),(#17548,#17549),(#17550,
#17551),(#17552,#17553),(#17554,#17555),(#17556,#17557),(#17558,#17559),
(#17560,#17561),(#17562,#17563),(#17564,#17565),(#17566,#17567),(#17568,
#17569),(#17570,#17571),(#17572,#17573),(#17574,#17575),(#17576,#17577),
(#17578,#17579),(#17580,#17581),(#17582,#17583),(#17584,#17585),(#17586,
#17587),(#17588,#17589),(#17590,#17591),(#17592,#17593),(#17594,#17595),
(#17596,#17597),(#17598,#17599),(#17600,#17601),(#17602,#17603),(#17604,
#17605),(#17606,#17607),(#17608,#17609),(#17610,#17611),(#17612,#17613),
(#17614,#17615),(#17616,#17617),(#17618,#17619),(#17620,#17621),(#17622,
#17623),(#17624,#17625),(#17626,#17627),(#17628,#17629),(#17630,#17631),
(#17632,#17633),(#17634,#17635),(#17636,#17637),(#17638,#17639),(#17640,
#17641),(#17642,#17643),(#17644,#17645),(#17646,#17647),(#17648,#17649),
(#17650,#17651),(#17652,#17653),(#17654,#17655),(#17656,#17657),(#17658,
#17659),(#17660,#17661),(#17662,#17663),(#17664,#17665),(#17666,#17667),
(#17668,#17669),(#17670,#17671),(#17672,#17673),(#17674,#17675),(#17676,
#17677),(#17678,#17679),(#17680,#17681),(#17682,#17683),(#17684,#17685),
(#17686,#17687),(#17688,#17689),(#17690,#17691),(#17692,#17693),(#17694,
#17695),(#17696,#17697),(#17698,#17699),(#17700,#17701),(#17702,#17703),
(#17704,#17705),(#17706,#17707),(#17708,#17709),(#17710,#17711),(#17712,
#17713),(#17714,#17715),(#17716,#17717),(#17718,#17719),(#17720,#17721),
(#17722,#17723),(#17724,#17725),(#17726,#17727),(#17728,#17729),(#17730,
#17731),(#17732,#17733),(#17734,#17735),(#17736,#17737),(#17738,#17739),
(#17740,#17741),(#17742,#17743),(#17744,#17745),(#17746,#17747),(#17748,
#17749),(#17750,#17751)),.UNSPECIFIED.,.T.,.F.,.F.,(6,1,1,1,1,1,1,1,1,1,
1,1,1,1,1,1,1,1,1,1,1,1,1,1,1,1,1,1,1,1,1,1,1,1,1,1,1,1,1,1,1,1,1,1,1,1,
1,1,1,1,1,1,1,1,1,1,1,1,1,1,1,1,1,1,1,1,1,1,1,1,1,1,1,1,1,1,1,1,1,1,1,1,
1,1,1,1,1,1,1,1,1,1,1,1,1,1,1,1,1,1,1,1,1,1,1,1,1,1,1,1,1,1,1,1,1,1,1,1,
1,1,1,1,1,1,1,1,1,1,1,1,1,1,1,1,1,1,1,1,1,1,1,1,1,1,1,1,1,1,1,1,1,1,1,1,
1,1,1,1,1,1,1,1,1,5,1,1,1,1,1,1,1,1,1,1,1,1,1,1,1,1,1,1,1,1,1,1,1,1,1,1,
1,1,1,1,1,1,1,1,1,1,1,1,1,1,1,1,1,1,1,1,1,1,1,1,1,1,1,1,1,1,1,1,1,1,1,1,
1,1,1,1,1,1,1,1,1,1,1,1,1,1,1,1,1,1,1,1,1,1,1,1,1,6),(2,2),(-0.648016352593037,
-0.648,-0.644,-0.64,-0.636,-0.632,-0.628,-0.624,-0.62,-0.616,-0.612,-0.608,
-0.604,-0.6,-0.596,-0.592,-0.588,-0.584,-0.58,-0.576,-0.572,-0.568,-0.564,
-0.56,-0.556,-0.552,-0.548,-0.544,-0.54,-0.536,-0.532,-0.528,-0.524,-0.52,
-0.516,-0.512,-0.508,-0.504,-0.5,-0.496,-0.492,-0.488,-0.484,-0.48,-0.476,
-0.472,-0.468,-0.464,-0.46,-0.456,-0.452,-0.448,-0.444,-0.44,-0.436,-0.432,
-0.428,-0.424,-0.42,-0.416,-0.412,-0.408,-0.404,-0.4,-0.396,-0.392,-0.388,
-0.384,-0.38,-0.376,-0.372,-0.368,-0.364,-0.36,-0.356,-0.352,-0.348,-0.344,
-0.34,-0.336,-0.332,-0.328,-0.324,-0.32,-0.316,-0.312,-0.308,-0.304,-0.3,
-0.296,-0.292,-0.288,-0.284,-0.28,-0.276,-0.272,-0.268,-0.264,-0.26,-0.256,
-0.252,-0.248,-0.244,-0.24,-0.236,-0.232,-0.228,-0.224,-0.22,-0.216,-0.212,
-0.208,-0.204,-0.2,-0.196,-0.192,-0.188,-0.184,-0.18,-0.176,-0.172,-0.168,
-0.164,-0.16,-0.156,-0.152,-0.148,-0.144,-0.14,-0.136,-0.132,-0.128,-0.124,
-0.12,-0.116,-0.112,-0.108,-0.104,-0.1,-0.0960000000000001,-0.0920000000000001,
-0.0880000000000001,-0.084,-0.08,-0.076,-0.072,-0.068,-0.064,-0.06,-0.056,
-0.052,-0.048,-0.044,-0.04,-0.036,-0.032,-0.028,-0.024,-0.02,-0.016,-0.012,
-0.008,-0.004,0.,0.00399999999999923,0.00799999999999923,0.0119999999999992,
0.0159999999999992,0.0199999999999992,0.0239999999999992,0.0279999999999992,
0.0319999999999993,0.0359999999999993,0.0399999999999993,0.0439999999999993,
0.0479999999999993,0.0519999999999993,0.0559999999999993,0.0599999999999993,
0.0639999999999993,0.0679999999999993,0.0719999999999993,0.0759999999999993,
0.0799999999999993,0.0839999999999993,0.0879999999999993,0.0919999999999993,
0.0959999999999993,0.0999999999999993,0.103999999999999,0.107999999999999,
0.111999999999999,0.115999999999999,0.119999999999999,0.123999999999999,
0.127999999999999,0.131999999999999,0.135999999999999,0.139999999999999,
0.143999999999999,0.147999999999999,0.151999999999999,0.155999999999999,
0.159999999999999,0.163999999999999,0.167999999999999,0.171999999999999,
0.175999999999999,0.179999999999999,0.183999999999999,0.187999999999999,
0.191999999999999,0.195999999999999,0.199999999999999,0.203999999999999,
0.207999999999999,0.211999999999999,0.215999999999999,0.219999999999999,
0.223999999999999,0.227999999999999,0.231999999999999,0.235999999999999,
0.239999999999999,0.243999999999999,0.247999999999999,0.251999999999999,
0.255999999999999,0.259999999999999,0.263999999999999,0.267999999999999,
0.271999999999999,0.275999999999999,0.279999999999999,0.283999999999999,
0.287999999999999,0.291999999999999,0.295999999999999,0.299999999999999,
0.303999999999999,0.307999999999999,0.311999999999999,0.316,0.32,0.324,
0.328,0.332,0.336,0.34,0.344,0.348,0.351983647406963),(0.,0.878547542022766),
 .UNSPECIFIED.);
#318=B_SPLINE_SURFACE_WITH_KNOTS('',3,1,((#17757,#17758),(#17759,#17760),
(#17761,#17762),(#17763,#17764),(#17765,#17766)),.UNSPECIFIED.,.F.,.F.,
 .F.,(4,1,4),(2,2),(0.,0.571428571428571,1.),(0.,0.51269230976995),
 .UNSPECIFIED.);
#319=B_SPLINE_SURFACE_WITH_KNOTS('',5,1,((#17785,#17786),(#17787,#17788),
(#17789,#17790),(#17791,#17792),(#17793,#17794),(#17795,#17796),(#17797,
#17798),(#17799,#17800),(#17801,#17802),(#17803,#17804),(#17805,#17806),
(#17807,#17808),(#17809,#17810),(#17811,#17812),(#17813,#17814),(#17815,
#17816),(#17817,#17818),(#17819,#17820),(#17821,#17822),(#17823,#17824),
(#17825,#17826),(#17827,#17828),(#17829,#17830),(#17831,#17832),(#17833,
#17834),(#17835,#17836),(#17837,#17838),(#17839,#17840),(#17841,#17842),
(#17843,#17844),(#17845,#17846),(#17847,#17848),(#17849,#17850),(#17851,
#17852),(#17853,#17854),(#17855,#17856),(#17857,#17858),(#17859,#17860),
(#17861,#17862),(#17863,#17864),(#17865,#17866),(#17867,#17868),(#17869,
#17870),(#17871,#17872),(#17873,#17874),(#17875,#17876),(#17877,#17878),
(#17879,#17880),(#17881,#17882),(#17883,#17884),(#17885,#17886),(#17887,
#17888),(#17889,#17890),(#17891,#17892),(#17893,#17894),(#17895,#17896),
(#17897,#17898),(#17899,#17900),(#17901,#17902),(#17903,#17904),(#17905,
#17906),(#17907,#17908),(#17909,#17910),(#17911,#17912),(#17913,#17914),
(#17915,#17916),(#17917,#17918),(#17919,#17920),(#17921,#17922),(#17923,
#17924),(#17925,#17926),(#17927,#17928),(#17929,#17930),(#17931,#17932),
(#17933,#17934),(#17935,#17936),(#17937,#17938),(#17939,#17940),(#17941,
#17942),(#17943,#17944),(#17945,#17946),(#17947,#17948),(#17949,#17950),
(#17951,#17952),(#17953,#17954),(#17955,#17956),(#17957,#17958),(#17959,
#17960),(#17961,#17962),(#17963,#17964),(#17965,#17966),(#17967,#17968),
(#17969,#17970),(#17971,#17972),(#17973,#17974),(#17975,#17976),(#17977,
#17978),(#17979,#17980),(#17981,#17982),(#17983,#17984),(#17985,#17986),
(#17987,#17988),(#17989,#17990),(#17991,#17992),(#17993,#17994),(#17995,
#17996),(#17997,#17998),(#17999,#18000),(#18001,#18002),(#18003,#18004),
(#18005,#18006),(#18007,#18008),(#18009,#18010),(#18011,#18012),(#18013,
#18014),(#18015,#18016),(#18017,#18018),(#18019,#18020),(#18021,#18022),
(#18023,#18024),(#18025,#18026),(#18027,#18028),(#18029,#18030),(#18031,
#18032),(#18033,#18034),(#18035,#18036),(#18037,#18038),(#18039,#18040),
(#18041,#18042),(#18043,#18044),(#18045,#18046),(#18047,#18048),(#18049,
#18050),(#18051,#18052),(#18053,#18054),(#18055,#18056),(#18057,#18058),
(#18059,#18060),(#18061,#18062),(#18063,#18064),(#18065,#18066),(#18067,
#18068),(#18069,#18070),(#18071,#18072),(#18073,#18074),(#18075,#18076),
(#18077,#18078),(#18079,#18080),(#18081,#18082),(#18083,#18084),(#18085,
#18086),(#18087,#18088),(#18089,#18090),(#18091,#18092),(#18093,#18094),
(#18095,#18096),(#18097,#18098),(#18099,#18100),(#18101,#18102),(#18103,
#18104),(#18105,#18106),(#18107,#18108),(#18109,#18110),(#18111,#18112),
(#18113,#18114),(#18115,#18116),(#18117,#18118),(#18119,#18120),(#18121,
#18122),(#18123,#18124),(#18125,#18126),(#18127,#18128),(#18129,#18130),
(#18131,#18132),(#18133,#18134),(#18135,#18136),(#18137,#18138),(#18139,
#18140),(#18141,#18142),(#18143,#18144),(#18145,#18146),(#18147,#18148),
(#18149,#18150),(#18151,#18152),(#18153,#18154),(#18155,#18156),(#18157,
#18158),(#18159,#18160),(#18161,#18162),(#18163,#18164),(#18165,#18166),
(#18167,#18168),(#18169,#18170),(#18171,#18172),(#18173,#18174),(#18175,
#18176),(#18177,#18178),(#18179,#18180),(#18181,#18182),(#18183,#18184),
(#18185,#18186),(#18187,#18188),(#18189,#18190),(#18191,#18192),(#18193,
#18194),(#18195,#18196),(#18197,#18198),(#18199,#18200),(#18201,#18202),
(#18203,#18204),(#18205,#18206),(#18207,#18208),(#18209,#18210),(#18211,
#18212),(#18213,#18214),(#18215,#18216),(#18217,#18218),(#18219,#18220),
(#18221,#18222),(#18223,#18224),(#18225,#18226),(#18227,#18228),(#18229,
#18230),(#18231,#18232),(#18233,#18234),(#18235,#18236),(#18237,#18238),
(#18239,#18240),(#18241,#18242),(#18243,#18244),(#18245,#18246),(#18247,
#18248),(#18249,#18250),(#18251,#18252),(#18253,#18254),(#18255,#18256),
(#18257,#18258),(#18259,#18260),(#18261,#18262),(#18263,#18264),(#18265,
#18266),(#18267,#18268),(#18269,#18270),(#18271,#18272),(#18273,#18274),
(#18275,#18276),(#18277,#18278),(#18279,#18280),(#18281,#18282),(#18283,
#18284),(#18285,#18286),(#18287,#18288),(#18289,#18290),(#18291,#18292),
(#18293,#18294),(#18295,#18296),(#18297,#18298),(#18299,#18300),(#18301,
#18302),(#18303,#18304)),.UNSPECIFIED.,.T.,.F.,.F.,(6,1,1,1,1,1,1,1,1,1,
1,1,1,1,1,1,1,1,1,1,1,1,1,1,1,1,1,1,1,1,1,1,1,1,1,1,1,1,1,1,1,1,1,1,1,1,
1,1,1,1,1,1,1,1,1,1,1,1,1,1,1,1,1,1,1,1,1,1,1,1,1,1,1,1,1,1,1,1,1,1,1,5,
1,1,1,1,1,1,1,1,1,1,1,1,1,1,1,1,1,1,1,1,1,1,1,1,1,1,1,1,1,1,1,1,1,1,1,1,
1,1,1,1,1,1,1,1,1,1,1,1,1,1,1,1,1,1,1,1,1,1,1,1,1,1,1,1,1,1,1,1,1,1,1,1,
1,1,1,1,1,1,1,1,1,1,1,1,1,1,1,1,1,1,1,1,1,1,1,1,1,1,1,1,1,1,1,1,1,1,1,1,
1,1,1,1,1,1,1,1,1,1,1,1,1,1,1,1,1,1,1,1,1,1,1,1,1,1,1,1,1,1,1,1,1,1,1,1,
1,1,1,1,1,1,1,1,1,1,1,1,1,1,1,1,1,1,1,1,1,1,1,1,1,6),(2,2),(-0.322416215027029,
-0.32,-0.316,-0.312,-0.308,-0.304,-0.3,-0.296,-0.292,-0.288,-0.284,-0.28,
-0.276,-0.272,-0.268,-0.264,-0.26,-0.256,-0.252,-0.248,-0.244,-0.24,-0.236,
-0.232,-0.228,-0.224,-0.22,-0.216,-0.212,-0.208,-0.204,-0.2,-0.196,-0.192,
-0.188,-0.184,-0.18,-0.176,-0.172,-0.168,-0.164,-0.16,-0.156,-0.152,-0.148,
-0.144,-0.14,-0.136,-0.132,-0.128,-0.124,-0.12,-0.116,-0.112,-0.108,-0.104,
-0.1,-0.0960000000000001,-0.0920000000000001,-0.0880000000000001,-0.084,
-0.08,-0.076,-0.072,-0.068,-0.064,-0.06,-0.056,-0.052,-0.048,-0.044,-0.04,
-0.036,-0.032,-0.028,-0.024,-0.02,-0.016,-0.012,-0.008,-0.004,0.,0.00399999999999923,
0.00799999999999923,0.0119999999999992,0.0159999999999992,0.0199999999999992,
0.0239999999999992,0.0279999999999992,0.0319999999999993,0.0359999999999993,
0.0399999999999993,0.0439999999999993,0.0479999999999993,0.0519999999999993,
0.0559999999999993,0.0599999999999993,0.0639999999999993,0.0679999999999993,
0.0719999999999993,0.0759999999999993,0.0799999999999993,0.0839999999999993,
0.0879999999999993,0.0919999999999993,0.0959999999999993,0.0999999999999993,
0.103999999999999,0.107999999999999,0.111999999999999,0.115999999999999,
0.119999999999999,0.123999999999999,0.127999999999999,0.131999999999999,
0.135999999999999,0.139999999999999,0.143999999999999,0.147999999999999,
0.151999999999999,0.155999999999999,0.159999999999999,0.163999999999999,
0.167999999999999,0.171999999999999,0.175999999999999,0.179999999999999,
0.183999999999999,0.187999999999999,0.191999999999999,0.195999999999999,
0.199999999999999,0.203999999999999,0.207999999999999,0.211999999999999,
0.215999999999999,0.219999999999999,0.223999999999999,0.227999999999999,
0.231999999999999,0.235999999999999,0.239999999999999,0.243999999999999,
0.247999999999999,0.251999999999999,0.255999999999999,0.259999999999999,
0.263999999999999,0.267999999999999,0.271999999999999,0.275999999999999,
0.279999999999999,0.283999999999999,0.287999999999999,0.291999999999999,
0.295999999999999,0.299999999999999,0.303999999999999,0.307999999999999,
0.311999999999999,0.316,0.32,0.324,0.328,0.332,0.336,0.34,0.344,0.348,0.352,
0.356,0.36,0.364,0.368,0.372,0.376,0.38,0.384,0.388,0.392,0.396,0.4,0.404,
0.408,0.412,0.416,0.42,0.424,0.428,0.432,0.436,0.44,0.444,0.448,0.452,0.456,
0.46,0.464,0.468,0.472,0.476,0.48,0.484,0.488,0.492,0.496,0.5,0.504,0.508,
0.512,0.516,0.52,0.524,0.528,0.532,0.536,0.54,0.544,0.548,0.552,0.556,0.56,
0.564,0.568,0.572,0.576,0.58,0.584,0.588,0.592,0.596,0.6,0.604,0.608,0.612,
0.616,0.62,0.624,0.628,0.632,0.636,0.64,0.644,0.648,0.652,0.656,0.66,0.664,
0.668,0.672,0.676,0.677583784972971),(0.,7.2),.UNSPECIFIED.);
#320=B_SPLINE_SURFACE_WITH_KNOTS('',3,3,((#18315,#18316,#18317,#18318),
(#18319,#18320,#18321,#18322),(#18323,#18324,#18325,#18326),(#18327,#18328,
#18329,#18330)),.UNSPECIFIED.,.F.,.F.,.F.,(4,4),(4,4),(0.,1.),(0.214918350132049,
0.48911828449592),.UNSPECIFIED.);
#321=B_SPLINE_SURFACE_WITH_KNOTS('',3,3,((#18350,#18351,#18352,#18353),
(#18354,#18355,#18356,#18357),(#18358,#18359,#18360,#18361),(#18362,#18363,
#18364,#18365)),.UNSPECIFIED.,.F.,.F.,.F.,(4,4),(4,4),(0.,1.),(0.,0.197269104818139),
 .UNSPECIFIED.);
#322=B_SPLINE_SURFACE_WITH_KNOTS('',3,3,((#18377,#18378,#18379,#18380),
(#18381,#18382,#18383,#18384),(#18385,#18386,#18387,#18388),(#18389,#18390,
#18391,#18392)),.UNSPECIFIED.,.F.,.F.,.F.,(4,4),(4,4),(-0.0471135960368116,
1.),(-0.237658380445436,7.56806292790953E-5),.UNSPECIFIED.);
#323=B_SPLINE_SURFACE_WITH_KNOTS('',3,3,((#18408,#18409,#18410,#18411,#18412,
#18413),(#18414,#18415,#18416,#18417,#18418,#18419),(#18420,#18421,#18422,
#18423,#18424,#18425),(#18426,#18427,#18428,#18429,#18430,#18431)),
 .UNSPECIFIED.,.F.,.F.,.F.,(4,4),(4,2,4),(0.,1.),(0.,0.471468502883735,
0.473994966708672),.UNSPECIFIED.);
#324=B_SPLINE_SURFACE_WITH_KNOTS('',3,3,((#18452,#18453,#18454,#18455),
(#18456,#18457,#18458,#18459),(#18460,#18461,#18462,#18463),(#18464,#18465,
#18466,#18467)),.UNSPECIFIED.,.F.,.F.,.F.,(4,4),(4,4),(0.,1.),(1.89854339553983E-15,
0.0666641979607186),.UNSPECIFIED.);
#325=B_SPLINE_SURFACE_WITH_KNOTS('',3,3,((#18476,#18477,#18478,#18479),
(#18480,#18481,#18482,#18483),(#18484,#18485,#18486,#18487),(#18488,#18489,
#18490,#18491)),.UNSPECIFIED.,.F.,.F.,.F.,(4,4),(4,4),(0.186511816400127,
1.),(-1.01772858153936,-0.745004297261558),.UNSPECIFIED.);
#326=B_SPLINE_SURFACE_WITH_KNOTS('',3,3,((#18506,#18507,#18508,#18509),
(#18510,#18511,#18512,#18513),(#18514,#18515,#18516,#18517),(#18518,#18519,
#18520,#18521)),.UNSPECIFIED.,.F.,.F.,.F.,(4,4),(4,4),(0.165314557349038,
1.),(-0.195956842698031,-5.68173586430139E-15),.UNSPECIFIED.);
#327=B_SPLINE_SURFACE_WITH_KNOTS('',3,3,((#18523,#18524,#18525,#18526,#18527,
#18528),(#18529,#18530,#18531,#18532,#18533,#18534),(#18535,#18536,#18537,
#18538,#18539,#18540),(#18541,#18542,#18543,#18544,#18545,#18546)),
 .UNSPECIFIED.,.F.,.F.,.F.,(4,4),(4,2,4),(0.144606210418872,1.),(-0.531787427886525,
-0.530925715886322,0.),.UNSPECIFIED.);
#328=B_SPLINE_SURFACE_WITH_KNOTS('',3,3,((#18547,#18548,#18549,#18550,#18551,
#18552),(#18553,#18554,#18555,#18556,#18557,#18558),(#18559,#18560,#18561,
#18562,#18563,#18564),(#18565,#18566,#18567,#18568,#18569,#18570)),
 .UNSPECIFIED.,.F.,.F.,.F.,(4,4),(4,2,4),(0.,1.02106399261821),(-0.880320663133757,
0.,0.00551932282830541),.UNSPECIFIED.);
#329=B_SPLINE_SURFACE_WITH_KNOTS('',3,3,((#18652,#18653,#18654,#18655),
(#18656,#18657,#18658,#18659),(#18660,#18661,#18662,#18663),(#18664,#18665,
#18666,#18667),(#18668,#18669,#18670,#18671)),.UNSPECIFIED.,.F.,.F.,.F.,
(4,1,4),(4,4),(0.,0.571428571428571,1.00011302068706),(-0.000113020687060352,
0.32384869792086),.UNSPECIFIED.);
#330=B_SPLINE_SURFACE_WITH_KNOTS('',3,3,((#18692,#18693,#18694,#18695),
(#18696,#18697,#18698,#18699),(#18700,#18701,#18702,#18703),(#18704,#18705,
#18706,#18707),(#18708,#18709,#18710,#18711)),.UNSPECIFIED.,.F.,.F.,.F.,
(4,1,4),(4,4),(0.,0.5,1.),(0.,0.105411804182902),.UNSPECIFIED.);
#331=B_SPLINE_SURFACE_WITH_KNOTS('',3,3,((#18722,#18723,#18724,#18725),
(#18726,#18727,#18728,#18729),(#18730,#18731,#18732,#18733),(#18734,#18735,
#18736,#18737),(#18738,#18739,#18740,#18741)),.UNSPECIFIED.,.F.,.F.,.F.,
(4,1,4),(4,4),(0.,0.571428571428571,1.),(0.0597111975742865,0.0778887211231013),
 .UNSPECIFIED.);
#332=B_SPLINE_SURFACE_WITH_KNOTS('',3,3,((#18747,#18748,#18749,#18750,#18751,
#18752,#18753),(#18754,#18755,#18756,#18757,#18758,#18759,#18760),(#18761,
#18762,#18763,#18764,#18765,#18766,#18767),(#18768,#18769,#18770,#18771,
#18772,#18773,#18774),(#18775,#18776,#18777,#18778,#18779,#18780,#18781),
(#18782,#18783,#18784,#18785,#18786,#18787,#18788)),.UNSPECIFIED.,.F.,.F.,
 .F.,(4,1,1,4),(4,1,1,1,4),(0.,0.285714285714286,0.571428571428571,1.),
(-1.84302877518546E-14,0.0336059064221182,0.0672118128442549,0.11201968807377,
0.156827563303286),.UNSPECIFIED.);
#333=B_SPLINE_SURFACE_WITH_KNOTS('',3,3,((#18807,#18808,#18809,#18810,#18811),
(#18812,#18813,#18814,#18815,#18816),(#18817,#18818,#18819,#18820,#18821),
(#18822,#18823,#18824,#18825,#18826),(#18827,#18828,#18829,#18830,#18831)),
 .UNSPECIFIED.,.F.,.F.,.F.,(4,1,4),(4,1,4),(0.,0.571428571428571,1.),(4.07518504807266E-15,
0.0864360398355901,0.172872079671176),.UNSPECIFIED.);
#334=B_SPLINE_SURFACE_WITH_KNOTS('',3,3,((#18845,#18846,#18847,#18848),
(#18849,#18850,#18851,#18852),(#18853,#18854,#18855,#18856),(#18857,#18858,
#18859,#18860),(#18861,#18862,#18863,#18864)),.UNSPECIFIED.,.F.,.F.,.F.,
(4,1,4),(4,4),(0.,0.571428571428571,1.),(0.00704588444375797,0.110567549348147),
 .UNSPECIFIED.);
#335=B_SPLINE_SURFACE_WITH_KNOTS('',3,1,((#18892,#18893),(#18894,#18895),
(#18896,#18897),(#18898,#18899),(#18900,#18901)),.UNSPECIFIED.,.F.,.F.,
 .F.,(4,1,4),(2,2),(0.,0.367757184420533,0.643575072735933),(0.,0.504000000000047),
 .UNSPECIFIED.);
#336=B_SPLINE_SURFACE_WITH_KNOTS('',5,1,((#18910,#18911),(#18912,#18913),
(#18914,#18915),(#18916,#18917),(#18918,#18919),(#18920,#18921),(#18922,
#18923),(#18924,#18925),(#18926,#18927),(#18928,#18929),(#18930,#18931),
(#18932,#18933),(#18934,#18935),(#18936,#18937),(#18938,#18939),(#18940,
#18941),(#18942,#18943),(#18944,#18945),(#18946,#18947),(#18948,#18949),
(#18950,#18951),(#18952,#18953),(#18954,#18955),(#18956,#18957),(#18958,
#18959),(#18960,#18961),(#18962,#18963),(#18964,#18965),(#18966,#18967),
(#18968,#18969),(#18970,#18971),(#18972,#18973),(#18974,#18975),(#18976,
#18977),(#18978,#18979),(#18980,#18981),(#18982,#18983),(#18984,#18985),
(#18986,#18987),(#18988,#18989),(#18990,#18991),(#18992,#18993),(#18994,
#18995),(#18996,#18997),(#18998,#18999),(#19000,#19001),(#19002,#19003),
(#19004,#19005),(#19006,#19007),(#19008,#19009),(#19010,#19011),(#19012,
#19013),(#19014,#19015),(#19016,#19017),(#19018,#19019),(#19020,#19021),
(#19022,#19023),(#19024,#19025),(#19026,#19027),(#19028,#19029),(#19030,
#19031),(#19032,#19033),(#19034,#19035),(#19036,#19037),(#19038,#19039),
(#19040,#19041),(#19042,#19043),(#19044,#19045),(#19046,#19047),(#19048,
#19049),(#19050,#19051),(#19052,#19053),(#19054,#19055),(#19056,#19057),
(#19058,#19059),(#19060,#19061),(#19062,#19063),(#19064,#19065),(#19066,
#19067),(#19068,#19069),(#19070,#19071),(#19072,#19073),(#19074,#19075),
(#19076,#19077),(#19078,#19079),(#19080,#19081),(#19082,#19083),(#19084,
#19085),(#19086,#19087),(#19088,#19089),(#19090,#19091),(#19092,#19093),
(#19094,#19095),(#19096,#19097),(#19098,#19099),(#19100,#19101),(#19102,
#19103),(#19104,#19105),(#19106,#19107),(#19108,#19109),(#19110,#19111),
(#19112,#19113),(#19114,#19115),(#19116,#19117),(#19118,#19119),(#19120,
#19121),(#19122,#19123),(#19124,#19125),(#19126,#19127),(#19128,#19129),
(#19130,#19131),(#19132,#19133),(#19134,#19135),(#19136,#19137),(#19138,
#19139),(#19140,#19141),(#19142,#19143),(#19144,#19145),(#19146,#19147),
(#19148,#19149),(#19150,#19151),(#19152,#19153),(#19154,#19155),(#19156,
#19157),(#19158,#19159),(#19160,#19161),(#19162,#19163),(#19164,#19165),
(#19166,#19167),(#19168,#19169),(#19170,#19171),(#19172,#19173),(#19174,
#19175),(#19176,#19177),(#19178,#19179),(#19180,#19181),(#19182,#19183),
(#19184,#19185),(#19186,#19187),(#19188,#19189),(#19190,#19191),(#19192,
#19193),(#19194,#19195),(#19196,#19197),(#19198,#19199),(#19200,#19201),
(#19202,#19203),(#19204,#19205),(#19206,#19207),(#19208,#19209),(#19210,
#19211),(#19212,#19213),(#19214,#19215),(#19216,#19217),(#19218,#19219),
(#19220,#19221),(#19222,#19223),(#19224,#19225),(#19226,#19227),(#19228,
#19229),(#19230,#19231),(#19232,#19233),(#19234,#19235),(#19236,#19237),
(#19238,#19239),(#19240,#19241),(#19242,#19243),(#19244,#19245),(#19246,
#19247),(#19248,#19249),(#19250,#19251),(#19252,#19253),(#19254,#19255),
(#19256,#19257),(#19258,#19259),(#19260,#19261),(#19262,#19263),(#19264,
#19265),(#19266,#19267),(#19268,#19269),(#19270,#19271),(#19272,#19273),
(#19274,#19275),(#19276,#19277),(#19278,#19279),(#19280,#19281),(#19282,
#19283),(#19284,#19285),(#19286,#19287),(#19288,#19289),(#19290,#19291),
(#19292,#19293),(#19294,#19295),(#19296,#19297),(#19298,#19299),(#19300,
#19301),(#19302,#19303),(#19304,#19305),(#19306,#19307),(#19308,#19309),
(#19310,#19311),(#19312,#19313),(#19314,#19315),(#19316,#19317),(#19318,
#19319),(#19320,#19321),(#19322,#19323),(#19324,#19325),(#19326,#19327),
(#19328,#19329),(#19330,#19331),(#19332,#19333),(#19334,#19335),(#19336,
#19337),(#19338,#19339),(#19340,#19341),(#19342,#19343),(#19344,#19345),
(#19346,#19347),(#19348,#19349),(#19350,#19351),(#19352,#19353),(#19354,
#19355),(#19356,#19357),(#19358,#19359),(#19360,#19361),(#19362,#19363),
(#19364,#19365),(#19366,#19367),(#19368,#19369),(#19370,#19371),(#19372,
#19373),(#19374,#19375),(#19376,#19377),(#19378,#19379),(#19380,#19381),
(#19382,#19383),(#19384,#19385),(#19386,#19387),(#19388,#19389),(#19390,
#19391),(#19392,#19393),(#19394,#19395),(#19396,#19397),(#19398,#19399),
(#19400,#19401),(#19402,#19403),(#19404,#19405),(#19406,#19407),(#19408,
#19409),(#19410,#19411),(#19412,#19413),(#19414,#19415),(#19416,#19417),
(#19418,#19419),(#19420,#19421),(#19422,#19423),(#19424,#19425),(#19426,
#19427),(#19428,#19429)),.UNSPECIFIED.,.T.,.F.,.F.,(6,1,1,1,1,1,1,1,1,1,
1,1,1,1,1,1,1,1,1,1,1,1,1,1,1,1,1,1,1,1,1,1,1,1,1,1,1,1,1,1,1,1,1,1,1,1,
1,1,1,1,1,1,1,1,1,1,1,1,1,1,1,1,1,1,1,1,1,1,1,1,1,1,1,1,1,1,1,1,1,1,1,1,
1,1,1,1,1,1,1,1,1,1,1,1,1,1,1,1,1,1,1,1,1,1,1,1,1,1,1,1,1,1,1,1,1,1,1,1,
1,1,1,1,1,1,1,1,1,1,1,1,1,1,1,1,1,1,1,1,1,1,1,1,1,1,1,1,1,1,1,1,1,1,1,1,
1,1,1,1,1,1,1,1,1,1,1,1,1,1,1,1,1,1,1,1,1,1,1,1,1,1,1,1,1,1,1,1,1,1,1,1,
1,1,1,1,1,1,1,1,1,1,1,1,1,1,1,1,1,1,1,1,1,1,1,1,1,1,1,1,1,1,1,1,1,1,1,1,
1,1,1,1,1,1,1,1,1,5,1,1,1,1,1,1,1,1,1,1,1,1,1,1,1,6),(2,2),(-0.939015270874982,
-0.936000000000001,-0.932000000000001,-0.928000000000001,-0.924000000000001,
-0.920000000000001,-0.916000000000001,-0.912000000000001,-0.908000000000001,
-0.904000000000001,-0.900000000000001,-0.896000000000001,-0.892000000000001,
-0.888000000000001,-0.884000000000001,-0.880000000000001,-0.876000000000001,
-0.872000000000001,-0.868000000000001,-0.864000000000001,-0.860000000000001,
-0.856000000000001,-0.852000000000001,-0.848000000000001,-0.844000000000001,
-0.840000000000001,-0.836000000000001,-0.832000000000001,-0.828000000000001,
-0.824000000000001,-0.820000000000001,-0.816000000000001,-0.812000000000001,
-0.808000000000001,-0.804000000000001,-0.800000000000001,-0.796000000000001,
-0.792000000000001,-0.788000000000001,-0.784000000000001,-0.780000000000001,
-0.776000000000001,-0.772000000000001,-0.768000000000001,-0.764000000000001,
-0.760000000000001,-0.756000000000001,-0.752000000000001,-0.748000000000001,
-0.744000000000001,-0.740000000000001,-0.736000000000001,-0.732000000000001,
-0.728000000000001,-0.724000000000001,-0.720000000000001,-0.716000000000001,
-0.712000000000001,-0.708000000000001,-0.704000000000001,-0.700000000000001,
-0.696000000000001,-0.692000000000001,-0.688000000000001,-0.684,-0.68,-0.676,
-0.672,-0.668,-0.664,-0.66,-0.656,-0.652,-0.648,-0.644,-0.64,-0.636,-0.632,
-0.628,-0.624,-0.62,-0.616,-0.612,-0.608,-0.604,-0.6,-0.596,-0.592,-0.588,
-0.584,-0.58,-0.576,-0.572,-0.568,-0.564,-0.56,-0.556,-0.552,-0.548,-0.544,
-0.54,-0.536,-0.532,-0.528,-0.524,-0.52,-0.516,-0.512,-0.508,-0.504,-0.5,
-0.496,-0.492,-0.488,-0.484,-0.48,-0.476,-0.472,-0.468,-0.464,-0.46,-0.456,
-0.452,-0.448,-0.444,-0.44,-0.436,-0.432,-0.428,-0.424,-0.42,-0.416,-0.412,
-0.408,-0.404,-0.4,-0.396,-0.392,-0.388,-0.384,-0.38,-0.376,-0.372,-0.368,
-0.364,-0.36,-0.356,-0.352,-0.348,-0.344,-0.34,-0.336,-0.332,-0.328,-0.324,
-0.32,-0.316,-0.312,-0.308,-0.304,-0.3,-0.296,-0.292,-0.288,-0.284,-0.28,
-0.276,-0.272,-0.268,-0.264,-0.26,-0.256,-0.252,-0.248,-0.244,-0.24,-0.236,
-0.232,-0.228,-0.224,-0.22,-0.216,-0.212,-0.208,-0.204,-0.2,-0.196,-0.192,
-0.188,-0.184,-0.18,-0.176,-0.172,-0.168,-0.164,-0.16,-0.156,-0.152,-0.148,
-0.144,-0.14,-0.136,-0.132,-0.128,-0.124,-0.12,-0.116,-0.112,-0.108,-0.104,
-0.1,-0.0960000000000001,-0.0920000000000001,-0.0880000000000001,-0.084,
-0.08,-0.076,-0.072,-0.068,-0.064,-0.06,-0.056,-0.052,-0.048,-0.044,-0.04,
-0.036,-0.032,-0.028,-0.024,-0.02,-0.016,-0.012,-0.008,-0.004,0.,0.00399999999999923,
0.00799999999999923,0.0119999999999992,0.0159999999999992,0.0199999999999992,
0.0239999999999992,0.0279999999999992,0.0319999999999993,0.0359999999999993,
0.0399999999999993,0.0439999999999993,0.0479999999999993,0.0519999999999993,
0.0559999999999993,0.0599999999999993,0.0609847291250184),(0.,2.16728151094469),
 .UNSPECIFIED.);
#337=B_SPLINE_SURFACE_WITH_KNOTS('',5,1,((#19434,#19435),(#19436,#19437),
(#19438,#19439),(#19440,#19441),(#19442,#19443),(#19444,#19445),(#19446,
#19447),(#19448,#19449),(#19450,#19451),(#19452,#19453),(#19454,#19455),
(#19456,#19457),(#19458,#19459),(#19460,#19461),(#19462,#19463),(#19464,
#19465),(#19466,#19467),(#19468,#19469),(#19470,#19471),(#19472,#19473),
(#19474,#19475),(#19476,#19477),(#19478,#19479),(#19480,#19481),(#19482,
#19483),(#19484,#19485),(#19486,#19487),(#19488,#19489),(#19490,#19491),
(#19492,#19493),(#19494,#19495),(#19496,#19497),(#19498,#19499),(#19500,
#19501),(#19502,#19503),(#19504,#19505),(#19506,#19507),(#19508,#19509),
(#19510,#19511),(#19512,#19513),(#19514,#19515),(#19516,#19517),(#19518,
#19519),(#19520,#19521),(#19522,#19523),(#19524,#19525),(#19526,#19527),
(#19528,#19529),(#19530,#19531),(#19532,#19533),(#19534,#19535),(#19536,
#19537),(#19538,#19539),(#19540,#19541),(#19542,#19543),(#19544,#19545),
(#19546,#19547),(#19548,#19549),(#19550,#19551),(#19552,#19553),(#19554,
#19555),(#19556,#19557),(#19558,#19559),(#19560,#19561),(#19562,#19563),
(#19564,#19565),(#19566,#19567),(#19568,#19569),(#19570,#19571),(#19572,
#19573),(#19574,#19575),(#19576,#19577),(#19578,#19579),(#19580,#19581),
(#19582,#19583),(#19584,#19585),(#19586,#19587),(#19588,#19589),(#19590,
#19591),(#19592,#19593),(#19594,#19595),(#19596,#19597),(#19598,#19599),
(#19600,#19601),(#19602,#19603),(#19604,#19605),(#19606,#19607),(#19608,
#19609),(#19610,#19611),(#19612,#19613),(#19614,#19615),(#19616,#19617),
(#19618,#19619),(#19620,#19621),(#19622,#19623),(#19624,#19625),(#19626,
#19627),(#19628,#19629),(#19630,#19631),(#19632,#19633),(#19634,#19635),
(#19636,#19637),(#19638,#19639),(#19640,#19641),(#19642,#19643),(#19644,
#19645),(#19646,#19647),(#19648,#19649),(#19650,#19651),(#19652,#19653),
(#19654,#19655),(#19656,#19657),(#19658,#19659),(#19660,#19661),(#19662,
#19663),(#19664,#19665),(#19666,#19667),(#19668,#19669),(#19670,#19671),
(#19672,#19673),(#19674,#19675),(#19676,#19677),(#19678,#19679),(#19680,
#19681),(#19682,#19683),(#19684,#19685),(#19686,#19687),(#19688,#19689),
(#19690,#19691),(#19692,#19693),(#19694,#19695),(#19696,#19697),(#19698,
#19699),(#19700,#19701),(#19702,#19703),(#19704,#19705),(#19706,#19707),
(#19708,#19709),(#19710,#19711),(#19712,#19713),(#19714,#19715),(#19716,
#19717),(#19718,#19719),(#19720,#19721),(#19722,#19723),(#19724,#19725),
(#19726,#19727),(#19728,#19729),(#19730,#19731),(#19732,#19733),(#19734,
#19735),(#19736,#19737),(#19738,#19739),(#19740,#19741),(#19742,#19743),
(#19744,#19745),(#19746,#19747),(#19748,#19749),(#19750,#19751),(#19752,
#19753),(#19754,#19755),(#19756,#19757),(#19758,#19759),(#19760,#19761),
(#19762,#19763),(#19764,#19765),(#19766,#19767),(#19768,#19769),(#19770,
#19771),(#19772,#19773),(#19774,#19775),(#19776,#19777),(#19778,#19779),
(#19780,#19781),(#19782,#19783),(#19784,#19785),(#19786,#19787),(#19788,
#19789),(#19790,#19791),(#19792,#19793),(#19794,#19795),(#19796,#19797),
(#19798,#19799),(#19800,#19801),(#19802,#19803),(#19804,#19805),(#19806,
#19807),(#19808,#19809),(#19810,#19811),(#19812,#19813),(#19814,#19815),
(#19816,#19817),(#19818,#19819),(#19820,#19821),(#19822,#19823),(#19824,
#19825),(#19826,#19827),(#19828,#19829),(#19830,#19831),(#19832,#19833),
(#19834,#19835),(#19836,#19837),(#19838,#19839),(#19840,#19841),(#19842,
#19843),(#19844,#19845),(#19846,#19847),(#19848,#19849),(#19850,#19851),
(#19852,#19853),(#19854,#19855),(#19856,#19857),(#19858,#19859),(#19860,
#19861),(#19862,#19863),(#19864,#19865),(#19866,#19867),(#19868,#19869),
(#19870,#19871),(#19872,#19873),(#19874,#19875),(#19876,#19877),(#19878,
#19879),(#19880,#19881),(#19882,#19883),(#19884,#19885),(#19886,#19887),
(#19888,#19889),(#19890,#19891),(#19892,#19893),(#19894,#19895),(#19896,
#19897),(#19898,#19899),(#19900,#19901),(#19902,#19903),(#19904,#19905),
(#19906,#19907),(#19908,#19909),(#19910,#19911),(#19912,#19913),(#19914,
#19915),(#19916,#19917),(#19918,#19919),(#19920,#19921),(#19922,#19923),
(#19924,#19925),(#19926,#19927),(#19928,#19929),(#19930,#19931),(#19932,
#19933),(#19934,#19935),(#19936,#19937),(#19938,#19939),(#19940,#19941),
(#19942,#19943),(#19944,#19945),(#19946,#19947),(#19948,#19949),(#19950,
#19951),(#19952,#19953)),.UNSPECIFIED.,.T.,.F.,.F.,(6,1,1,1,1,1,1,1,1,1,
1,1,1,1,1,1,1,1,1,1,1,1,1,1,1,1,1,1,1,1,1,1,1,1,1,1,1,1,1,1,1,1,1,1,1,1,
1,1,1,1,1,1,1,1,1,1,1,1,1,1,1,1,1,1,1,1,1,1,1,1,1,1,1,1,1,1,1,1,1,1,1,1,
1,1,1,1,1,1,1,1,1,1,1,1,1,1,1,1,1,1,1,1,1,1,1,1,1,1,1,1,1,1,1,1,1,1,1,1,
1,1,1,1,1,1,1,1,1,1,1,1,1,1,1,1,1,1,1,1,1,1,1,1,1,1,1,1,1,1,1,1,1,1,1,1,
1,1,1,1,1,1,1,1,1,1,1,1,1,1,1,1,1,1,1,1,1,1,1,1,1,1,1,1,1,1,1,1,1,1,1,1,
1,1,1,1,1,1,1,1,1,1,1,1,1,1,1,1,1,1,1,1,1,1,1,1,1,1,1,1,1,1,1,1,1,1,1,1,
1,1,1,1,1,1,1,1,1,5,1,1,1,1,1,1,1,1,1,1,1,1,1,1,1,6),(2,2),(-0.938590041217468,
-0.936000000000001,-0.932000000000001,-0.928000000000001,-0.924000000000001,
-0.920000000000001,-0.916000000000001,-0.912000000000001,-0.908000000000001,
-0.904000000000001,-0.900000000000001,-0.896000000000001,-0.892000000000001,
-0.888000000000001,-0.884000000000001,-0.880000000000001,-0.876000000000001,
-0.872000000000001,-0.868000000000001,-0.864000000000001,-0.860000000000001,
-0.856000000000001,-0.852000000000001,-0.848000000000001,-0.844000000000001,
-0.840000000000001,-0.836000000000001,-0.832000000000001,-0.828000000000001,
-0.824000000000001,-0.820000000000001,-0.816000000000001,-0.812000000000001,
-0.808000000000001,-0.804000000000001,-0.800000000000001,-0.796000000000001,
-0.792000000000001,-0.788000000000001,-0.784000000000001,-0.780000000000001,
-0.776000000000001,-0.772000000000001,-0.768000000000001,-0.764000000000001,
-0.760000000000001,-0.756000000000001,-0.752000000000001,-0.748000000000001,
-0.744000000000001,-0.740000000000001,-0.736000000000001,-0.732000000000001,
-0.728000000000001,-0.724000000000001,-0.720000000000001,-0.716000000000001,
-0.712000000000001,-0.708000000000001,-0.704000000000001,-0.700000000000001,
-0.696000000000001,-0.692000000000001,-0.688000000000001,-0.684,-0.68,-0.676,
-0.672,-0.668,-0.664,-0.66,-0.656,-0.652,-0.648,-0.644,-0.64,-0.636,-0.632,
-0.628,-0.624,-0.62,-0.616,-0.612,-0.608,-0.604,-0.6,-0.596,-0.592,-0.588,
-0.584,-0.58,-0.576,-0.572,-0.568,-0.564,-0.56,-0.556,-0.552,-0.548,-0.544,
-0.54,-0.536,-0.532,-0.528,-0.524,-0.52,-0.516,-0.512,-0.508,-0.504,-0.5,
-0.496,-0.492,-0.488,-0.484,-0.48,-0.476,-0.472,-0.468,-0.464,-0.46,-0.456,
-0.452,-0.448,-0.444,-0.44,-0.436,-0.432,-0.428,-0.424,-0.42,-0.416,-0.412,
-0.408,-0.404,-0.4,-0.396,-0.392,-0.388,-0.384,-0.38,-0.376,-0.372,-0.368,
-0.364,-0.36,-0.356,-0.352,-0.348,-0.344,-0.34,-0.336,-0.332,-0.328,-0.324,
-0.32,-0.316,-0.312,-0.308,-0.304,-0.3,-0.296,-0.292,-0.288,-0.284,-0.28,
-0.276,-0.272,-0.268,-0.264,-0.26,-0.256,-0.252,-0.248,-0.244,-0.24,-0.236,
-0.232,-0.228,-0.224,-0.22,-0.216,-0.212,-0.208,-0.204,-0.2,-0.196,-0.192,
-0.188,-0.184,-0.18,-0.176,-0.172,-0.168,-0.164,-0.16,-0.156,-0.152,-0.148,
-0.144,-0.14,-0.136,-0.132,-0.128,-0.124,-0.12,-0.116,-0.112,-0.108,-0.104,
-0.1,-0.0960000000000001,-0.0920000000000001,-0.0880000000000001,-0.084,
-0.08,-0.076,-0.072,-0.068,-0.064,-0.06,-0.056,-0.052,-0.048,-0.044,-0.04,
-0.036,-0.032,-0.028,-0.024,-0.02,-0.016,-0.012,-0.008,-0.004,0.,0.00399999999999923,
0.00799999999999923,0.0119999999999992,0.0159999999999992,0.0199999999999992,
0.0239999999999992,0.0279999999999992,0.0319999999999993,0.0359999999999993,
0.0399999999999993,0.0439999999999993,0.0479999999999993,0.0519999999999993,
0.0559999999999993,0.0599999999999993,0.0614099587825321),(0.,0.936109769296308),
 .UNSPECIFIED.);
#338=B_SPLINE_SURFACE_WITH_KNOTS('',3,3,((#19994,#19995,#19996,#19997,#19998,
#19999,#20000,#20001,#20002,#20003,#20004,#20005,#20006,#20007,#20008,#20009,
#20010,#20011,#20012,#20013,#20014,#20015,#20016,#20017,#20018,#20019,#20020,
#20021,#20022,#20023,#20024,#20025,#20026,#20027),(#20028,#20029,#20030,
#20031,#20032,#20033,#20034,#20035,#20036,#20037,#20038,#20039,#20040,#20041,
#20042,#20043,#20044,#20045,#20046,#20047,#20048,#20049,#20050,#20051,#20052,
#20053,#20054,#20055,#20056,#20057,#20058,#20059,#20060,#20061),(#20062,
#20063,#20064,#20065,#20066,#20067,#20068,#20069,#20070,#20071,#20072,#20073,
#20074,#20075,#20076,#20077,#20078,#20079,#20080,#20081,#20082,#20083,#20084,
#20085,#20086,#20087,#20088,#20089,#20090,#20091,#20092,#20093,#20094,#20095),
(#20096,#20097,#20098,#20099,#20100,#20101,#20102,#20103,#20104,#20105,
#20106,#20107,#20108,#20109,#20110,#20111,#20112,#20113,#20114,#20115,#20116,
#20117,#20118,#20119,#20120,#20121,#20122,#20123,#20124,#20125,#20126,#20127,
#20128,#20129),(#20130,#20131,#20132,#20133,#20134,#20135,#20136,#20137,
#20138,#20139,#20140,#20141,#20142,#20143,#20144,#20145,#20146,#20147,#20148,
#20149,#20150,#20151,#20152,#20153,#20154,#20155,#20156,#20157,#20158,#20159,
#20160,#20161,#20162,#20163)),.UNSPECIFIED.,.F.,.F.,.F.,(4,1,4),(4,1,1,
1,1,1,1,1,1,1,1,1,1,1,1,1,1,1,1,1,1,1,1,1,1,1,1,1,1,1,1,4),(0.,0.571428571428571,
1.),(0.,0.438300757907035,0.876601515814069,1.3149022737211,1.75320303162814,
2.19150378953517,2.62980454744221,3.50640606325628,4.01775694748115,4.09080707379899,
4.6752080843417,4.96740858961306,5.11350884224874,5.25960909488442,5.55180960015577,
5.84401010542713,6.42841111596984,7.01281212651256,7.30501263178391,7.59721313705527,
8.18161414759798,8.76601515814069,9.05821566341205,9.35041616868341,9.64261667395476,
9.93481717922612,10.5192181897688,10.6287933792456,10.9575189476759,11.3958197055829,
11.8341204634899,12.272421221397),.UNSPECIFIED.);
#339=B_SPLINE_SURFACE_WITH_KNOTS('',3,3,((#20178,#20179,#20180,#20181),
(#20182,#20183,#20184,#20185),(#20186,#20187,#20188,#20189),(#20190,#20191,
#20192,#20193),(#20194,#20195,#20196,#20197)),.UNSPECIFIED.,.F.,.F.,.F.,
(4,1,4),(4,4),(0.,0.571428571428571,1.),(0.,0.164738445253465),
 .UNSPECIFIED.);
#340=B_SPLINE_SURFACE_WITH_KNOTS('',3,3,((#20212,#20213,#20214,#20215),
(#20216,#20217,#20218,#20219),(#20220,#20221,#20222,#20223),(#20224,#20225,
#20226,#20227),(#20228,#20229,#20230,#20231)),.UNSPECIFIED.,.F.,.F.,.F.,
(4,1,4),(4,4),(0.,0.571428571428571,1.),(0.,0.0754181362626584),
 .UNSPECIFIED.);
#341=B_SPLINE_SURFACE_WITH_KNOTS('',3,3,((#20243,#20244,#20245,#20246),
(#20247,#20248,#20249,#20250),(#20251,#20252,#20253,#20254),(#20255,#20256,
#20257,#20258),(#20259,#20260,#20261,#20262)),.UNSPECIFIED.,.F.,.F.,.F.,
(4,1,4),(4,4),(0.,0.571428571428571,1.),(0.,0.0505696713863416),
 .UNSPECIFIED.);
#342=B_SPLINE_SURFACE_WITH_KNOTS('',3,3,((#20274,#20275,#20276,#20277,#20278),
(#20279,#20280,#20281,#20282,#20283),(#20284,#20285,#20286,#20287,#20288),
(#20289,#20290,#20291,#20292,#20293),(#20294,#20295,#20296,#20297,#20298)),
 .UNSPECIFIED.,.F.,.F.,.F.,(4,1,4),(4,1,4),(0.,0.571428571428571,1.),(0.,
0.0837730396707311,0.167546079341462),.UNSPECIFIED.);
#343=B_SPLINE_SURFACE_WITH_KNOTS('',3,3,((#20309,#20310,#20311,#20312,#20313),
(#20314,#20315,#20316,#20317,#20318),(#20319,#20320,#20321,#20322,#20323),
(#20324,#20325,#20326,#20327,#20328),(#20329,#20330,#20331,#20332,#20333)),
 .UNSPECIFIED.,.F.,.F.,.F.,(4,1,4),(4,1,4),(-2.33603068056626E-9,0.571428571428571,
1.00000203313126),(-0.0971295855432269,-0.0737466502954258,-0.0503637127115938),
 .UNSPECIFIED.);
#344=B_SPLINE_SURFACE_WITH_KNOTS('',5,1,((#20382,#20383),(#20384,#20385),
(#20386,#20387),(#20388,#20389),(#20390,#20391),(#20392,#20393),(#20394,
#20395),(#20396,#20397),(#20398,#20399),(#20400,#20401),(#20402,#20403),
(#20404,#20405),(#20406,#20407),(#20408,#20409),(#20410,#20411),(#20412,
#20413),(#20414,#20415),(#20416,#20417),(#20418,#20419),(#20420,#20421),
(#20422,#20423),(#20424,#20425),(#20426,#20427),(#20428,#20429)),
 .UNSPECIFIED.,.F.,.F.,.F.,(6,1,1,1,1,1,1,1,1,1,1,1,1,1,1,1,1,1,1,6),(2,
2),(-0.421786698696643,-0.42,-0.416,-0.412,-0.408,-0.404,-0.4,-0.396,-0.392,
-0.388,-0.384,-0.38,-0.376,-0.372,-0.368,-0.364,-0.36,-0.356,-0.352,-0.351983647406963),
(0.,7.2),.UNSPECIFIED.);
#345=B_SPLINE_SURFACE_WITH_KNOTS('',3,3,((#20446,#20447,#20448,#20449),
(#20450,#20451,#20452,#20453),(#20454,#20455,#20456,#20457),(#20458,#20459,
#20460,#20461)),.UNSPECIFIED.,.F.,.F.,.F.,(4,4),(4,4),(-2.28168025676385E-5,
1.),(-0.0965691449411131,-0.0938109728066715),.UNSPECIFIED.);
#346=B_SPLINE_SURFACE_WITH_KNOTS('',3,3,((#20463,#20464,#20465,#20466,#20467,
#20468,#20469,#20470,#20471,#20472,#20473,#20474,#20475,#20476,#20477,#20478,
#20479,#20480,#20481,#20482),(#20483,#20484,#20485,#20486,#20487,#20488,
#20489,#20490,#20491,#20492,#20493,#20494,#20495,#20496,#20497,#20498,#20499,
#20500,#20501,#20502),(#20503,#20504,#20505,#20506,#20507,#20508,#20509,
#20510,#20511,#20512,#20513,#20514,#20515,#20516,#20517,#20518,#20519,#20520,
#20521,#20522),(#20523,#20524,#20525,#20526,#20527,#20528,#20529,#20530,
#20531,#20532,#20533,#20534,#20535,#20536,#20537,#20538,#20539,#20540,#20541,
#20542),(#20543,#20544,#20545,#20546,#20547,#20548,#20549,#20550,#20551,
#20552,#20553,#20554,#20555,#20556,#20557,#20558,#20559,#20560,#20561,#20562)),
 .UNSPECIFIED.,.F.,.F.,.F.,(4,1,4),(4,1,1,1,1,1,1,1,1,1,1,1,1,1,1,1,1,4),
(0.,0.571428571428571,1.),(0.,0.197097619692083,0.394195239384165,0.689841668922289,
0.78839047876833,0.886939288614372,0.985488098460413,1.08403690830645,1.1825857181525,
1.37968333784458,1.47823214769062,1.57678095753666,1.62605536245968,1.6753297673827,
1.77387857722874,1.97097619692083,2.36517143630499,2.75936667568916),
 .UNSPECIFIED.);
#347=B_SPLINE_SURFACE_WITH_KNOTS('',3,3,((#20785,#20786,#20787,#20788),
(#20789,#20790,#20791,#20792),(#20793,#20794,#20795,#20796),(#20797,#20798,
#20799,#20800),(#20801,#20802,#20803,#20804)),.UNSPECIFIED.,.F.,.F.,.F.,
(4,1,4),(4,4),(0.,0.571428571428571,1.),(0.,0.304037814733278),
 .UNSPECIFIED.);
#348=B_SPLINE_SURFACE_WITH_KNOTS('',3,3,((#20816,#20817,#20818,#20819,#20820,
#20821,#20822,#20823,#20824,#20825,#20826,#20827,#20828,#20829,#20830,#20831,
#20832,#20833,#20834,#20835,#20836),(#20837,#20838,#20839,#20840,#20841,
#20842,#20843,#20844,#20845,#20846,#20847,#20848,#20849,#20850,#20851,#20852,
#20853,#20854,#20855,#20856,#20857),(#20858,#20859,#20860,#20861,#20862,
#20863,#20864,#20865,#20866,#20867,#20868,#20869,#20870,#20871,#20872,#20873,
#20874,#20875,#20876,#20877,#20878),(#20879,#20880,#20881,#20882,#20883,
#20884,#20885,#20886,#20887,#20888,#20889,#20890,#20891,#20892,#20893,#20894,
#20895,#20896,#20897,#20898,#20899),(#20900,#20901,#20902,#20903,#20904,
#20905,#20906,#20907,#20908,#20909,#20910,#20911,#20912,#20913,#20914,#20915,
#20916,#20917,#20918,#20919,#20920)),.UNSPECIFIED.,.F.,.F.,.F.,(4,1,4),
(4,1,1,1,1,1,1,1,1,1,1,1,1,1,1,1,1,1,4),(0.,0.571428571428571,1.),(0.,0.148302061038192,
0.296604122076384,0.444906183114576,0.593208244152768,0.889812366229152,
1.18641648830554,1.7796247324583,2.37283297661107,4.74566595322215,5.93208244152768,
6.52529068568045,7.11849892983322,7.4151030519096,7.71170717398599,7.86000923502418,
8.00831129606237,8.15661335710056,8.30491541813876),.UNSPECIFIED.);
#349=B_SPLINE_SURFACE_WITH_KNOTS('',3,3,((#20946,#20947,#20948,#20949),
(#20950,#20951,#20952,#20953),(#20954,#20955,#20956,#20957),(#20958,#20959,
#20960,#20961),(#20962,#20963,#20964,#20965)),.UNSPECIFIED.,.F.,.F.,.F.,
(4,1,4),(4,4),(0.,0.571428571428571,1.),(0.,0.0801298062965183),
 .UNSPECIFIED.);
#350=B_SPLINE_SURFACE_WITH_KNOTS('',3,3,((#20974,#20975,#20976,#20977),
(#20978,#20979,#20980,#20981),(#20982,#20983,#20984,#20985),(#20986,#20987,
#20988,#20989),(#20990,#20991,#20992,#20993)),.UNSPECIFIED.,.F.,.F.,.F.,
(4,1,4),(4,4),(0.,0.571428571428571,1.),(0.0423193643606908,0.252933252504432),
 .UNSPECIFIED.);
#351=B_SPLINE_SURFACE_WITH_KNOTS('',3,3,((#20995,#20996,#20997,#20998),
(#20999,#21000,#21001,#21002),(#21003,#21004,#21005,#21006),(#21007,#21008,
#21009,#21010),(#21011,#21012,#21013,#21014)),.UNSPECIFIED.,.F.,.F.,.F.,
(4,1,4),(4,4),(0.,0.571428571428571,1.),(2.65444323739948E-13,0.080129806296636),
 .UNSPECIFIED.);
#352=B_SPLINE_SURFACE_WITH_KNOTS('',3,3,((#21199,#21200,#21201,#21202),
(#21203,#21204,#21205,#21206),(#21207,#21208,#21209,#21210),(#21211,#21212,
#21213,#21214),(#21215,#21216,#21217,#21218)),.UNSPECIFIED.,.F.,.F.,.F.,
(4,1,4),(4,4),(0.,0.571428571428571,1.),(0.,0.0200337106211744),
 .UNSPECIFIED.);
#353=B_SPLINE_SURFACE_WITH_KNOTS('',3,3,((#21222,#21223,#21224,#21225),
(#21226,#21227,#21228,#21229),(#21230,#21231,#21232,#21233),(#21234,#21235,
#21236,#21237),(#21238,#21239,#21240,#21241)),.UNSPECIFIED.,.F.,.F.,.F.,
(4,1,4),(4,4),(0.,0.571428571428571,1.),(0.,0.357185215222936),
 .UNSPECIFIED.);
#354=B_SPLINE_SURFACE_WITH_KNOTS('',3,3,((#21248,#21249,#21250,#21251,#21252,
#21253),(#21254,#21255,#21256,#21257,#21258,#21259),(#21260,#21261,#21262,
#21263,#21264,#21265),(#21266,#21267,#21268,#21269,#21270,#21271),(#21272,
#21273,#21274,#21275,#21276,#21277)),.UNSPECIFIED.,.F.,.F.,.F.,(4,1,4),
(4,1,1,4),(0.,0.5,1.),(0.0650388601395548,0.184879728366205,0.264773640517305,
0.344667552668405),.UNSPECIFIED.);
#355=B_SPLINE_SURFACE_WITH_KNOTS('',3,3,((#21288,#21289,#21290,#21291),
(#21292,#21293,#21294,#21295),(#21296,#21297,#21298,#21299),(#21300,#21301,
#21302,#21303),(#21304,#21305,#21306,#21307)),.UNSPECIFIED.,.F.,.F.,.F.,
(4,1,4),(4,4),(0.,0.571428571428571,1.),(0.,0.0647166470509305),
 .UNSPECIFIED.);
#356=B_SPLINE_SURFACE_WITH_KNOTS('',3,3,((#21309,#21310,#21311,#21312),
(#21313,#21314,#21315,#21316),(#21317,#21318,#21319,#21320),(#21321,#21322,
#21323,#21324)),.UNSPECIFIED.,.F.,.F.,.F.,(4,4),(4,4),(0.,1.),(0.,0.0229846076752987),
 .UNSPECIFIED.);
#357=B_SPLINE_SURFACE_WITH_KNOTS('',5,1,((#21330,#21331),(#21332,#21333),
(#21334,#21335),(#21336,#21337),(#21338,#21339),(#21340,#21341),(#21342,
#21343),(#21344,#21345),(#21346,#21347),(#21348,#21349),(#21350,#21351),
(#21352,#21353),(#21354,#21355),(#21356,#21357),(#21358,#21359),(#21360,
#21361),(#21362,#21363),(#21364,#21365),(#21366,#21367),(#21368,#21369),
(#21370,#21371),(#21372,#21373),(#21374,#21375),(#21376,#21377),(#21378,
#21379),(#21380,#21381),(#21382,#21383),(#21384,#21385),(#21386,#21387),
(#21388,#21389),(#21390,#21391),(#21392,#21393),(#21394,#21395),(#21396,
#21397),(#21398,#21399),(#21400,#21401),(#21402,#21403),(#21404,#21405),
(#21406,#21407),(#21408,#21409),(#21410,#21411),(#21412,#21413),(#21414,
#21415),(#21416,#21417),(#21418,#21419),(#21420,#21421),(#21422,#21423),
(#21424,#21425),(#21426,#21427),(#21428,#21429),(#21430,#21431),(#21432,
#21433),(#21434,#21435),(#21436,#21437),(#21438,#21439),(#21440,#21441),
(#21442,#21443),(#21444,#21445),(#21446,#21447),(#21448,#21449),(#21450,
#21451),(#21452,#21453),(#21454,#21455),(#21456,#21457),(#21458,#21459),
(#21460,#21461),(#21462,#21463),(#21464,#21465),(#21466,#21467),(#21468,
#21469),(#21470,#21471),(#21472,#21473),(#21474,#21475),(#21476,#21477),
(#21478,#21479),(#21480,#21481),(#21482,#21483),(#21484,#21485),(#21486,
#21487),(#21488,#21489),(#21490,#21491),(#21492,#21493),(#21494,#21495),
(#21496,#21497),(#21498,#21499),(#21500,#21501),(#21502,#21503),(#21504,
#21505),(#21506,#21507),(#21508,#21509),(#21510,#21511),(#21512,#21513),
(#21514,#21515),(#21516,#21517),(#21518,#21519),(#21520,#21521),(#21522,
#21523),(#21524,#21525),(#21526,#21527),(#21528,#21529),(#21530,#21531),
(#21532,#21533),(#21534,#21535),(#21536,#21537),(#21538,#21539),(#21540,
#21541),(#21542,#21543),(#21544,#21545),(#21546,#21547),(#21548,#21549),
(#21550,#21551),(#21552,#21553),(#21554,#21555),(#21556,#21557),(#21558,
#21559),(#21560,#21561),(#21562,#21563),(#21564,#21565),(#21566,#21567),
(#21568,#21569),(#21570,#21571),(#21572,#21573),(#21574,#21575),(#21576,
#21577),(#21578,#21579),(#21580,#21581),(#21582,#21583),(#21584,#21585),
(#21586,#21587),(#21588,#21589),(#21590,#21591),(#21592,#21593),(#21594,
#21595),(#21596,#21597),(#21598,#21599),(#21600,#21601),(#21602,#21603),
(#21604,#21605),(#21606,#21607),(#21608,#21609),(#21610,#21611),(#21612,
#21613),(#21614,#21615),(#21616,#21617),(#21618,#21619),(#21620,#21621),
(#21622,#21623),(#21624,#21625),(#21626,#21627),(#21628,#21629),(#21630,
#21631),(#21632,#21633),(#21634,#21635),(#21636,#21637),(#21638,#21639),
(#21640,#21641),(#21642,#21643),(#21644,#21645),(#21646,#21647),(#21648,
#21649),(#21650,#21651),(#21652,#21653),(#21654,#21655),(#21656,#21657),
(#21658,#21659),(#21660,#21661),(#21662,#21663),(#21664,#21665),(#21666,
#21667),(#21668,#21669),(#21670,#21671),(#21672,#21673),(#21674,#21675),
(#21676,#21677),(#21678,#21679),(#21680,#21681),(#21682,#21683),(#21684,
#21685),(#21686,#21687),(#21688,#21689),(#21690,#21691),(#21692,#21693),
(#21694,#21695),(#21696,#21697),(#21698,#21699),(#21700,#21701),(#21702,
#21703),(#21704,#21705),(#21706,#21707),(#21708,#21709),(#21710,#21711),
(#21712,#21713),(#21714,#21715),(#21716,#21717),(#21718,#21719),(#21720,
#21721),(#21722,#21723),(#21724,#21725),(#21726,#21727),(#21728,#21729),
(#21730,#21731),(#21732,#21733),(#21734,#21735),(#21736,#21737),(#21738,
#21739),(#21740,#21741),(#21742,#21743),(#21744,#21745),(#21746,#21747),
(#21748,#21749),(#21750,#21751),(#21752,#21753),(#21754,#21755),(#21756,
#21757),(#21758,#21759),(#21760,#21761),(#21762,#21763),(#21764,#21765),
(#21766,#21767),(#21768,#21769),(#21770,#21771),(#21772,#21773),(#21774,
#21775),(#21776,#21777),(#21778,#21779),(#21780,#21781),(#21782,#21783),
(#21784,#21785),(#21786,#21787),(#21788,#21789),(#21790,#21791),(#21792,
#21793),(#21794,#21795),(#21796,#21797),(#21798,#21799),(#21800,#21801),
(#21802,#21803),(#21804,#21805),(#21806,#21807),(#21808,#21809),(#21810,
#21811),(#21812,#21813),(#21814,#21815),(#21816,#21817),(#21818,#21819),
(#21820,#21821),(#21822,#21823),(#21824,#21825),(#21826,#21827),(#21828,
#21829),(#21830,#21831),(#21832,#21833),(#21834,#21835),(#21836,#21837),
(#21838,#21839),(#21840,#21841),(#21842,#21843),(#21844,#21845),(#21846,
#21847),(#21848,#21849)),.UNSPECIFIED.,.T.,.F.,.F.,(6,1,1,1,1,1,1,1,1,1,
1,1,1,1,1,1,1,1,1,1,1,1,1,1,1,1,1,1,1,1,1,1,1,1,1,1,1,1,1,1,1,1,1,1,1,1,
1,1,1,1,1,1,1,1,1,1,1,1,1,1,1,1,1,1,1,1,1,1,1,1,1,1,1,1,1,1,1,1,1,1,1,1,
1,1,1,1,1,1,1,1,1,1,1,1,1,1,1,1,1,1,1,1,1,1,1,1,1,1,1,1,1,1,1,1,1,1,1,1,
1,1,1,1,1,1,1,1,1,1,1,1,1,1,1,1,1,1,1,1,1,1,1,1,1,1,1,1,1,1,1,1,1,1,1,1,
1,1,1,1,1,1,1,1,1,1,1,1,1,1,1,1,1,1,1,1,1,1,1,1,1,1,1,1,1,1,1,1,1,1,1,1,
1,1,1,1,1,1,1,1,1,1,1,1,1,1,1,1,1,1,1,1,1,1,1,1,1,1,1,1,1,1,1,1,1,1,1,1,
1,1,1,1,1,1,1,1,1,5,1,1,1,1,1,1,1,1,1,1,1,1,1,1,1,6),(2,2),(-0.938590041217468,
-0.936000000000001,-0.932000000000001,-0.928000000000001,-0.924000000000001,
-0.920000000000001,-0.916000000000001,-0.912000000000001,-0.908000000000001,
-0.904000000000001,-0.900000000000001,-0.896000000000001,-0.892000000000001,
-0.888000000000001,-0.884000000000001,-0.880000000000001,-0.876000000000001,
-0.872000000000001,-0.868000000000001,-0.864000000000001,-0.860000000000001,
-0.856000000000001,-0.852000000000001,-0.848000000000001,-0.844000000000001,
-0.840000000000001,-0.836000000000001,-0.832000000000001,-0.828000000000001,
-0.824000000000001,-0.820000000000001,-0.816000000000001,-0.812000000000001,
-0.808000000000001,-0.804000000000001,-0.800000000000001,-0.796000000000001,
-0.792000000000001,-0.788000000000001,-0.784000000000001,-0.780000000000001,
-0.776000000000001,-0.772000000000001,-0.768000000000001,-0.764000000000001,
-0.760000000000001,-0.756000000000001,-0.752000000000001,-0.748000000000001,
-0.744000000000001,-0.740000000000001,-0.736000000000001,-0.732000000000001,
-0.728000000000001,-0.724000000000001,-0.720000000000001,-0.716000000000001,
-0.712000000000001,-0.708000000000001,-0.704000000000001,-0.700000000000001,
-0.696000000000001,-0.692000000000001,-0.688000000000001,-0.684,-0.68,-0.676,
-0.672,-0.668,-0.664,-0.66,-0.656,-0.652,-0.648,-0.644,-0.64,-0.636,-0.632,
-0.628,-0.624,-0.62,-0.616,-0.612,-0.608,-0.604,-0.6,-0.596,-0.592,-0.588,
-0.584,-0.58,-0.576,-0.572,-0.568,-0.564,-0.56,-0.556,-0.552,-0.548,-0.544,
-0.54,-0.536,-0.532,-0.528,-0.524,-0.52,-0.516,-0.512,-0.508,-0.504,-0.5,
-0.496,-0.492,-0.488,-0.484,-0.48,-0.476,-0.472,-0.468,-0.464,-0.46,-0.456,
-0.452,-0.448,-0.444,-0.44,-0.436,-0.432,-0.428,-0.424,-0.42,-0.416,-0.412,
-0.408,-0.404,-0.4,-0.396,-0.392,-0.388,-0.384,-0.38,-0.376,-0.372,-0.368,
-0.364,-0.36,-0.356,-0.352,-0.348,-0.344,-0.34,-0.336,-0.332,-0.328,-0.324,
-0.32,-0.316,-0.312,-0.308,-0.304,-0.3,-0.296,-0.292,-0.288,-0.284,-0.28,
-0.276,-0.272,-0.268,-0.264,-0.26,-0.256,-0.252,-0.248,-0.244,-0.24,-0.236,
-0.232,-0.228,-0.224,-0.22,-0.216,-0.212,-0.208,-0.204,-0.2,-0.196,-0.192,
-0.188,-0.184,-0.18,-0.176,-0.172,-0.168,-0.164,-0.16,-0.156,-0.152,-0.148,
-0.144,-0.14,-0.136,-0.132,-0.128,-0.124,-0.12,-0.116,-0.112,-0.108,-0.104,
-0.1,-0.0960000000000001,-0.0920000000000001,-0.0880000000000001,-0.084,
-0.08,-0.076,-0.072,-0.068,-0.064,-0.06,-0.056,-0.052,-0.048,-0.044,-0.04,
-0.036,-0.032,-0.028,-0.024,-0.02,-0.016,-0.012,-0.008,-0.004,0.,0.00399999999999923,
0.00799999999999923,0.0119999999999992,0.0159999999999992,0.0199999999999992,
0.0239999999999992,0.0279999999999992,0.0319999999999993,0.0359999999999993,
0.0399999999999993,0.0439999999999993,0.0479999999999993,0.0519999999999993,
0.0559999999999993,0.0599999999999993,0.0614099587825321),(0.,0.8496),
 .UNSPECIFIED.);
#358=B_SPLINE_SURFACE_WITH_KNOTS('',3,3,((#21860,#21861,#21862,#21863,#21864),
(#21865,#21866,#21867,#21868,#21869),(#21870,#21871,#21872,#21873,#21874),
(#21875,#21876,#21877,#21878,#21879),(#21880,#21881,#21882,#21883,#21884),
(#21885,#21886,#21887,#21888,#21889)),.UNSPECIFIED.,.F.,.F.,.F.,(4,1,1,
4),(4,1,4),(-6.44657208043772E-5,0.285714285714286,0.571428571428571,1.),
(0.0475827460273853,0.473360639981091,1.04097854429163),.UNSPECIFIED.);
#359=B_SPLINE_SURFACE_WITH_KNOTS('',3,3,((#21920,#21921,#21922,#21923,#21924,
#21925),(#21926,#21927,#21928,#21929,#21930,#21931),(#21932,#21933,#21934,
#21935,#21936,#21937),(#21938,#21939,#21940,#21941,#21942,#21943),(#21944,
#21945,#21946,#21947,#21948,#21949),(#21950,#21951,#21952,#21953,#21954,
#21955)),.UNSPECIFIED.,.F.,.F.,.F.,(4,1,1,4),(4,1,1,4),(0.331395853675239,
0.617940487814422,0.808970243907211,1.),(-0.0266531801543891,0.336302079828547,
0.698984668949978,1.24300855263212),.UNSPECIFIED.);
#360=B_SPLINE_SURFACE_WITH_KNOTS('',3,3,((#21956,#21957,#21958,#21959),
(#21960,#21961,#21962,#21963),(#21964,#21965,#21966,#21967),(#21968,#21969,
#21970,#21971),(#21972,#21973,#21974,#21975)),.UNSPECIFIED.,.F.,.F.,.F.,
(4,1,4),(4,4),(0.,0.571428571428571,1.),(0.19533758964745,0.254963272600067),
 .UNSPECIFIED.);
#361=B_SPLINE_SURFACE_WITH_KNOTS('',3,3,((#21983,#21984,#21985,#21986),
(#21987,#21988,#21989,#21990),(#21991,#21992,#21993,#21994),(#21995,#21996,
#21997,#21998),(#21999,#22000,#22001,#22002)),.UNSPECIFIED.,.F.,.F.,.F.,
(4,1,4),(4,4),(0.,0.571428571428571,1.),(2.63411853293822E-13,0.0801298062968181),
 .UNSPECIFIED.);
#362=B_SPLINE_SURFACE_WITH_KNOTS('',3,1,((#22009,#22010),(#22011,#22012),
(#22013,#22014),(#22015,#22016),(#22017,#22018)),.UNSPECIFIED.,.F.,.F.,
 .F.,(4,1,4),(2,2),(0.,0.5,1.),(0.,0.6),.UNSPECIFIED.);
#363=B_SPLINE_SURFACE_WITH_KNOTS('',3,3,((#22052,#22053,#22054,#22055,#22056),
(#22057,#22058,#22059,#22060,#22061),(#22062,#22063,#22064,#22065,#22066),
(#22067,#22068,#22069,#22070,#22071),(#22072,#22073,#22074,#22075,#22076),
(#22077,#22078,#22079,#22080,#22081)),.UNSPECIFIED.,.F.,.F.,.F.,(4,1,1,
4),(4,1,4),(-1.51321272498462E-5,0.285714285714286,0.571428571428571,1.),
(-6.52754885944507E-7,0.0874114081347553,0.17493857403387),
 .UNSPECIFIED.);
#364=B_SPLINE_SURFACE_WITH_KNOTS('',3,1,((#22105,#22106),(#22107,#22108),
(#22109,#22110),(#22111,#22112),(#22113,#22114)),.UNSPECIFIED.,.F.,.F.,
 .F.,(4,1,4),(2,2),(0.239075842950699,0.619537921475349,1.),(0.,0.410906527432635),
 .UNSPECIFIED.);
#365=B_SPLINE_SURFACE_WITH_KNOTS('',3,3,((#22118,#22119,#22120,#22121,#22122,
#22123),(#22124,#22125,#22126,#22127,#22128,#22129),(#22130,#22131,#22132,
#22133,#22134,#22135),(#22136,#22137,#22138,#22139,#22140,#22141),(#22142,
#22143,#22144,#22145,#22146,#22147)),.UNSPECIFIED.,.F.,.F.,.F.,(4,1,4),
(4,1,1,4),(0.,0.571428571428571,1.),(0.,0.107642143366443,0.179403572277406,
0.251165001188368),.UNSPECIFIED.);
#366=B_SPLINE_SURFACE_WITH_KNOTS('',3,3,((#22154,#22155,#22156,#22157),
(#22158,#22159,#22160,#22161),(#22162,#22163,#22164,#22165),(#22166,#22167,
#22168,#22169),(#22170,#22171,#22172,#22173)),.UNSPECIFIED.,.F.,.F.,.F.,
(4,1,4),(4,4),(0.,0.571428571428571,1.),(0.00243784671109485,0.137031673359032),
 .UNSPECIFIED.);
#367=B_SPLINE_SURFACE_WITH_KNOTS('',3,3,((#22182,#22183,#22184,#22185),
(#22186,#22187,#22188,#22189),(#22190,#22191,#22192,#22193),(#22194,#22195,
#22196,#22197),(#22198,#22199,#22200,#22201)),.UNSPECIFIED.,.F.,.F.,.F.,
(4,1,4),(4,4),(0.,0.571428571428571,1.),(0.,0.033167786256901),
 .UNSPECIFIED.);
#368=B_SPLINE_SURFACE_WITH_KNOTS('',3,3,((#22207,#22208,#22209,#22210,#22211,
#22212,#22213,#22214,#22215,#22216,#22217,#22218,#22219,#22220,#22221,#22222,
#22223,#22224,#22225,#22226),(#22227,#22228,#22229,#22230,#22231,#22232,
#22233,#22234,#22235,#22236,#22237,#22238,#22239,#22240,#22241,#22242,#22243,
#22244,#22245,#22246),(#22247,#22248,#22249,#22250,#22251,#22252,#22253,
#22254,#22255,#22256,#22257,#22258,#22259,#22260,#22261,#22262,#22263,#22264,
#22265,#22266),(#22267,#22268,#22269,#22270,#22271,#22272,#22273,#22274,
#22275,#22276,#22277,#22278,#22279,#22280,#22281,#22282,#22283,#22284,#22285,
#22286),(#22287,#22288,#22289,#22290,#22291,#22292,#22293,#22294,#22295,
#22296,#22297,#22298,#22299,#22300,#22301,#22302,#22303,#22304,#22305,#22306)),
 .UNSPECIFIED.,.F.,.F.,.F.,(4,1,4),(4,1,1,1,1,1,1,1,1,1,1,1,1,1,1,1,1,4),
(0.,0.571428571428571,1.),(0.00458897054204579,0.398834822329043,0.79308067411604,
0.990203600009539,1.02305742099179,1.05591124197404,1.12161888393854,1.18732652590304,
1.31874180983204,1.45015709376104,1.58157237769003,1.68013384063678,1.77869530358353,
1.97581822947703,2.07437969242378,2.17294115537053,2.37006408126403,2.76430993305103),
 .UNSPECIFIED.);
#369=B_SPLINE_SURFACE_WITH_KNOTS('',3,3,((#22503,#22504,#22505,#22506),
(#22507,#22508,#22509,#22510),(#22511,#22512,#22513,#22514),(#22515,#22516,
#22517,#22518)),.UNSPECIFIED.,.F.,.F.,.F.,(4,4),(4,4),(0.461946105359466,
1.),(-0.919615460485724,-0.751979757135207),.UNSPECIFIED.);
#370=B_SPLINE_SURFACE_WITH_KNOTS('',3,3,((#22527,#22528,#22529,#22530),
(#22531,#22532,#22533,#22534),(#22535,#22536,#22537,#22538),(#22539,#22540,
#22541,#22542),(#22543,#22544,#22545,#22546)),.UNSPECIFIED.,.F.,.F.,.F.,
(4,1,4),(4,4),(0.,0.571428571428571,1.),(0.0177382428884037,0.0280297096615123),
 .UNSPECIFIED.);
#371=B_SPLINE_SURFACE_WITH_KNOTS('',3,3,((#22549,#22550,#22551,#22552),
(#22553,#22554,#22555,#22556),(#22557,#22558,#22559,#22560),(#22561,#22562,
#22563,#22564)),.UNSPECIFIED.,.F.,.F.,.F.,(4,4),(4,4),(0.,1.),(0.0797065098565302,
0.419743206478425),.UNSPECIFIED.);
#372=B_SPLINE_SURFACE_WITH_KNOTS('',5,1,((#22575,#22576),(#22577,#22578),
(#22579,#22580),(#22581,#22582),(#22583,#22584),(#22585,#22586),(#22587,
#22588),(#22589,#22590),(#22591,#22592),(#22593,#22594),(#22595,#22596),
(#22597,#22598),(#22599,#22600),(#22601,#22602),(#22603,#22604),(#22605,
#22606),(#22607,#22608),(#22609,#22610),(#22611,#22612),(#22613,#22614),
(#22615,#22616),(#22617,#22618),(#22619,#22620),(#22621,#22622)),
 .UNSPECIFIED.,.F.,.F.,.F.,(6,1,1,1,1,1,1,1,1,1,1,1,1,1,1,1,1,1,1,6),(2,
2),(-0.421786698696643,-0.42,-0.416,-0.412,-0.408,-0.404,-0.4,-0.396,-0.392,
-0.388,-0.384,-0.38,-0.376,-0.372,-0.368,-0.364,-0.36,-0.356,-0.352,-0.351983647406963),
(0.,0.600000000000009),.UNSPECIFIED.);
#373=B_SPLINE_SURFACE_WITH_KNOTS('',3,3,((#22624,#22625,#22626,#22627),
(#22628,#22629,#22630,#22631),(#22632,#22633,#22634,#22635),(#22636,#22637,
#22638,#22639)),.UNSPECIFIED.,.F.,.F.,.F.,(4,4),(4,4),(0.,1.),(0.0253342885542915,
0.430969252801444),.UNSPECIFIED.);
#374=B_SPLINE_SURFACE_WITH_KNOTS('',3,1,((#22640,#22641),(#22642,#22643),
(#22644,#22645),(#22646,#22647),(#22648,#22649)),.UNSPECIFIED.,.F.,.F.,
 .F.,(4,1,4),(2,2),(0.,0.571428571428571,1.),(0.,0.504),.UNSPECIFIED.);
#375=B_SPLINE_SURFACE_WITH_KNOTS('',3,3,((#22651,#22652,#22653,#22654),
(#22655,#22656,#22657,#22658),(#22659,#22660,#22661,#22662),(#22663,#22664,
#22665,#22666),(#22667,#22668,#22669,#22670)),.UNSPECIFIED.,.F.,.F.,.F.,
(4,1,4),(4,4),(-0.000167747802972519,0.571428571428571,1.00016650641139),
(0.,0.17490202709838),.UNSPECIFIED.);
#376=B_SPLINE_SURFACE_WITH_KNOTS('',3,3,((#22677,#22678,#22679,#22680),
(#22681,#22682,#22683,#22684),(#22685,#22686,#22687,#22688),(#22689,#22690,
#22691,#22692),(#22693,#22694,#22695,#22696)),.UNSPECIFIED.,.F.,.F.,.F.,
(4,1,4),(4,4),(0.,0.571428571428571,1.),(0.,0.0459140586584383),
 .UNSPECIFIED.);
#377=B_SPLINE_SURFACE_WITH_KNOTS('',3,3,((#22703,#22704,#22705,#22706),
(#22707,#22708,#22709,#22710),(#22711,#22712,#22713,#22714),(#22715,#22716,
#22717,#22718),(#22719,#22720,#22721,#22722)),.UNSPECIFIED.,.F.,.F.,.F.,
(4,1,4),(4,4),(0.,0.571428571428571,1.),(0.0248279171959177,0.040552544467034),
 .UNSPECIFIED.);
#378=B_SPLINE_SURFACE_WITH_KNOTS('',3,3,((#22726,#22727,#22728,#22729),
(#22730,#22731,#22732,#22733),(#22734,#22735,#22736,#22737),(#22738,#22739,
#22740,#22741)),.UNSPECIFIED.,.F.,.F.,.F.,(4,4),(4,4),(0.287554629624749,
1.),(0.120808499840007,0.462316210796172),.UNSPECIFIED.);
#379=B_SPLINE_SURFACE_WITH_KNOTS('',5,1,((#22746,#22747),(#22748,#22749),
(#22750,#22751),(#22752,#22753),(#22754,#22755),(#22756,#22757),(#22758,
#22759),(#22760,#22761),(#22762,#22763),(#22764,#22765),(#22766,#22767),
(#22768,#22769),(#22770,#22771),(#22772,#22773),(#22774,#22775),(#22776,
#22777),(#22778,#22779),(#22780,#22781),(#22782,#22783),(#22784,#22785),
(#22786,#22787),(#22788,#22789),(#22790,#22791),(#22792,#22793)),
 .UNSPECIFIED.,.F.,.F.,.F.,(6,1,1,1,1,1,1,1,1,1,1,1,1,1,1,1,1,1,1,6),(2,
2),(-0.421786698696643,-0.42,-0.416,-0.412,-0.408,-0.404,-0.4,-0.396,-0.392,
-0.388,-0.384,-0.38,-0.376,-0.372,-0.368,-0.364,-0.36,-0.356,-0.352,-0.351983647406963),
(0.,7.2),.UNSPECIFIED.);
#380=B_SPLINE_SURFACE_WITH_KNOTS('',5,1,((#22799,#22800),(#22801,#22802),
(#22803,#22804),(#22805,#22806),(#22807,#22808),(#22809,#22810),(#22811,
#22812),(#22813,#22814),(#22815,#22816),(#22817,#22818),(#22819,#22820),
(#22821,#22822),(#22823,#22824),(#22825,#22826),(#22827,#22828),(#22829,
#22830),(#22831,#22832),(#22833,#22834),(#22835,#22836),(#22837,#22838),
(#22839,#22840),(#22841,#22842),(#22843,#22844),(#22845,#22846),(#22847,
#22848),(#22849,#22850),(#22851,#22852),(#22853,#22854),(#22855,#22856),
(#22857,#22858),(#22859,#22860),(#22861,#22862),(#22863,#22864),(#22865,
#22866),(#22867,#22868),(#22869,#22870),(#22871,#22872),(#22873,#22874),
(#22875,#22876),(#22877,#22878),(#22879,#22880),(#22881,#22882),(#22883,
#22884),(#22885,#22886),(#22887,#22888),(#22889,#22890),(#22891,#22892),
(#22893,#22894),(#22895,#22896),(#22897,#22898),(#22899,#22900),(#22901,
#22902),(#22903,#22904),(#22905,#22906),(#22907,#22908),(#22909,#22910),
(#22911,#22912),(#22913,#22914),(#22915,#22916),(#22917,#22918),(#22919,
#22920),(#22921,#22922),(#22923,#22924),(#22925,#22926),(#22927,#22928),
(#22929,#22930),(#22931,#22932),(#22933,#22934),(#22935,#22936),(#22937,
#22938),(#22939,#22940),(#22941,#22942),(#22943,#22944),(#22945,#22946),
(#22947,#22948),(#22949,#22950),(#22951,#22952),(#22953,#22954),(#22955,
#22956),(#22957,#22958),(#22959,#22960),(#22961,#22962),(#22963,#22964),
(#22965,#22966),(#22967,#22968),(#22969,#22970),(#22971,#22972),(#22973,
#22974),(#22975,#22976),(#22977,#22978),(#22979,#22980),(#22981,#22982),
(#22983,#22984),(#22985,#22986),(#22987,#22988),(#22989,#22990),(#22991,
#22992),(#22993,#22994),(#22995,#22996),(#22997,#22998),(#22999,#23000),
(#23001,#23002),(#23003,#23004),(#23005,#23006),(#23007,#23008),(#23009,
#23010),(#23011,#23012),(#23013,#23014),(#23015,#23016),(#23017,#23018),
(#23019,#23020),(#23021,#23022),(#23023,#23024),(#23025,#23026),(#23027,
#23028),(#23029,#23030),(#23031,#23032),(#23033,#23034),(#23035,#23036),
(#23037,#23038),(#23039,#23040),(#23041,#23042),(#23043,#23044),(#23045,
#23046),(#23047,#23048),(#23049,#23050),(#23051,#23052),(#23053,#23054),
(#23055,#23056),(#23057,#23058),(#23059,#23060),(#23061,#23062),(#23063,
#23064),(#23065,#23066),(#23067,#23068),(#23069,#23070),(#23071,#23072),
(#23073,#23074),(#23075,#23076),(#23077,#23078),(#23079,#23080),(#23081,
#23082),(#23083,#23084),(#23085,#23086),(#23087,#23088),(#23089,#23090),
(#23091,#23092),(#23093,#23094),(#23095,#23096),(#23097,#23098),(#23099,
#23100),(#23101,#23102),(#23103,#23104),(#23105,#23106),(#23107,#23108),
(#23109,#23110),(#23111,#23112),(#23113,#23114),(#23115,#23116),(#23117,
#23118),(#23119,#23120),(#23121,#23122),(#23123,#23124),(#23125,#23126),
(#23127,#23128),(#23129,#23130),(#23131,#23132),(#23133,#23134),(#23135,
#23136),(#23137,#23138),(#23139,#23140),(#23141,#23142),(#23143,#23144),
(#23145,#23146),(#23147,#23148),(#23149,#23150),(#23151,#23152),(#23153,
#23154),(#23155,#23156),(#23157,#23158),(#23159,#23160),(#23161,#23162),
(#23163,#23164),(#23165,#23166),(#23167,#23168),(#23169,#23170),(#23171,
#23172),(#23173,#23174),(#23175,#23176),(#23177,#23178),(#23179,#23180),
(#23181,#23182),(#23183,#23184),(#23185,#23186),(#23187,#23188),(#23189,
#23190),(#23191,#23192),(#23193,#23194),(#23195,#23196),(#23197,#23198),
(#23199,#23200),(#23201,#23202),(#23203,#23204),(#23205,#23206),(#23207,
#23208),(#23209,#23210),(#23211,#23212),(#23213,#23214),(#23215,#23216),
(#23217,#23218),(#23219,#23220),(#23221,#23222),(#23223,#23224),(#23225,
#23226),(#23227,#23228),(#23229,#23230),(#23231,#23232),(#23233,#23234),
(#23235,#23236),(#23237,#23238),(#23239,#23240),(#23241,#23242),(#23243,
#23244),(#23245,#23246),(#23247,#23248),(#23249,#23250),(#23251,#23252),
(#23253,#23254),(#23255,#23256),(#23257,#23258),(#23259,#23260),(#23261,
#23262),(#23263,#23264),(#23265,#23266),(#23267,#23268),(#23269,#23270),
(#23271,#23272),(#23273,#23274),(#23275,#23276),(#23277,#23278),(#23279,
#23280),(#23281,#23282),(#23283,#23284),(#23285,#23286),(#23287,#23288),
(#23289,#23290),(#23291,#23292),(#23293,#23294),(#23295,#23296),(#23297,
#23298),(#23299,#23300),(#23301,#23302),(#23303,#23304),(#23305,#23306),
(#23307,#23308),(#23309,#23310),(#23311,#23312),(#23313,#23314),(#23315,
#23316),(#23317,#23318)),.UNSPECIFIED.,.T.,.F.,.F.,(6,1,1,1,1,1,1,1,1,1,
1,1,1,1,1,1,1,1,1,1,1,1,1,1,1,1,1,1,1,1,1,1,1,1,1,1,1,1,1,1,1,1,1,1,1,1,
1,1,1,1,1,1,1,1,1,1,1,1,1,1,1,1,1,1,1,1,1,1,1,1,1,1,1,1,1,1,1,1,1,1,1,1,
1,1,1,1,1,1,1,1,1,1,1,1,1,1,1,1,1,1,1,1,1,1,1,1,1,1,1,1,1,1,1,1,1,1,1,1,
1,1,1,1,1,1,1,1,1,1,1,1,1,1,1,1,1,1,1,1,1,1,1,1,1,1,1,1,1,1,1,1,1,1,1,1,
1,1,1,1,1,1,1,1,1,1,1,1,1,1,1,1,1,1,1,1,1,1,1,1,1,1,1,1,1,1,1,1,1,1,1,1,
1,1,1,1,1,1,1,1,1,1,1,1,1,1,1,1,1,1,1,1,1,1,1,1,1,1,1,1,1,1,1,1,1,1,1,1,
1,1,1,1,1,1,1,1,1,5,1,1,1,1,1,1,1,1,1,1,1,1,1,1,1,6),(2,2),(-0.939015270874982,
-0.936000000000001,-0.932000000000001,-0.928000000000001,-0.924000000000001,
-0.920000000000001,-0.916000000000001,-0.912000000000001,-0.908000000000001,
-0.904000000000001,-0.900000000000001,-0.896000000000001,-0.892000000000001,
-0.888000000000001,-0.884000000000001,-0.880000000000001,-0.876000000000001,
-0.872000000000001,-0.868000000000001,-0.864000000000001,-0.860000000000001,
-0.856000000000001,-0.852000000000001,-0.848000000000001,-0.844000000000001,
-0.840000000000001,-0.836000000000001,-0.832000000000001,-0.828000000000001,
-0.824000000000001,-0.820000000000001,-0.816000000000001,-0.812000000000001,
-0.808000000000001,-0.804000000000001,-0.800000000000001,-0.796000000000001,
-0.792000000000001,-0.788000000000001,-0.784000000000001,-0.780000000000001,
-0.776000000000001,-0.772000000000001,-0.768000000000001,-0.764000000000001,
-0.760000000000001,-0.756000000000001,-0.752000000000001,-0.748000000000001,
-0.744000000000001,-0.740000000000001,-0.736000000000001,-0.732000000000001,
-0.728000000000001,-0.724000000000001,-0.720000000000001,-0.716000000000001,
-0.712000000000001,-0.708000000000001,-0.704000000000001,-0.700000000000001,
-0.696000000000001,-0.692000000000001,-0.688000000000001,-0.684,-0.68,-0.676,
-0.672,-0.668,-0.664,-0.66,-0.656,-0.652,-0.648,-0.644,-0.64,-0.636,-0.632,
-0.628,-0.624,-0.62,-0.616,-0.612,-0.608,-0.604,-0.6,-0.596,-0.592,-0.588,
-0.584,-0.58,-0.576,-0.572,-0.568,-0.564,-0.56,-0.556,-0.552,-0.548,-0.544,
-0.54,-0.536,-0.532,-0.528,-0.524,-0.52,-0.516,-0.512,-0.508,-0.504,-0.5,
-0.496,-0.492,-0.488,-0.484,-0.48,-0.476,-0.472,-0.468,-0.464,-0.46,-0.456,
-0.452,-0.448,-0.444,-0.44,-0.436,-0.432,-0.428,-0.424,-0.42,-0.416,-0.412,
-0.408,-0.404,-0.4,-0.396,-0.392,-0.388,-0.384,-0.38,-0.376,-0.372,-0.368,
-0.364,-0.36,-0.356,-0.352,-0.348,-0.344,-0.34,-0.336,-0.332,-0.328,-0.324,
-0.32,-0.316,-0.312,-0.308,-0.304,-0.3,-0.296,-0.292,-0.288,-0.284,-0.28,
-0.276,-0.272,-0.268,-0.264,-0.26,-0.256,-0.252,-0.248,-0.244,-0.24,-0.236,
-0.232,-0.228,-0.224,-0.22,-0.216,-0.212,-0.208,-0.204,-0.2,-0.196,-0.192,
-0.188,-0.184,-0.18,-0.176,-0.172,-0.168,-0.164,-0.16,-0.156,-0.152,-0.148,
-0.144,-0.14,-0.136,-0.132,-0.128,-0.124,-0.12,-0.116,-0.112,-0.108,-0.104,
-0.1,-0.0960000000000001,-0.0920000000000001,-0.0880000000000001,-0.084,
-0.08,-0.076,-0.072,-0.068,-0.064,-0.06,-0.056,-0.052,-0.048,-0.044,-0.04,
-0.036,-0.032,-0.028,-0.024,-0.02,-0.016,-0.012,-0.008,-0.004,0.,0.00399999999999923,
0.00799999999999923,0.0119999999999992,0.0159999999999992,0.0199999999999992,
0.0239999999999992,0.0279999999999992,0.0319999999999993,0.0359999999999993,
0.0399999999999993,0.0439999999999993,0.0479999999999993,0.0519999999999993,
0.0559999999999993,0.0599999999999993,0.0609847291250184),(0.,2.16728151094469),
 .UNSPECIFIED.);
#386=FACE_BOUND('',#2906,.T.);
#387=FACE_BOUND('',#2909,.T.);
#388=FACE_BOUND('',#2913,.T.);
#389=FACE_BOUND('',#2916,.T.);
#390=FACE_BOUND('',#3005,.T.);
#391=FACE_BOUND('',#3006,.T.);
#392=FACE_BOUND('',#3007,.T.);
#393=FACE_BOUND('',#3008,.T.);
#394=FACE_BOUND('',#3018,.T.);
#395=FACE_BOUND('',#3019,.T.);
#396=FACE_BOUND('',#3020,.T.);
#397=FACE_BOUND('',#3021,.T.);
#475=ELLIPSE('',#10109,0.179163796285099,0.132134456811432);
#476=ELLIPSE('',#10160,0.0711578408474482,0.0609612663807345);
#477=ELLIPSE('',#10161,0.643183425815913,0.414173412397355);
#478=ELLIPSE('',#10163,0.0804815181446777,0.0720771207638654);
#479=ELLIPSE('',#10165,0.062158381280911,0.0435390307992324);
#480=ELLIPSE('',#10177,0.0691697767700365,0.0595893379399011);
#481=ELLIPSE('',#10204,0.111726638420037,0.0803736621029293);
#482=ELLIPSE('',#10214,0.0704571051122974,0.0497299141222001);
#483=ELLIPSE('',#10227,0.417631904706076,0.321033921213905);
#484=ELLIPSE('',#10257,0.224701868798773,0.0973759172030223);
#485=ELLIPSE('',#10259,0.14551373866235,0.0747733658362826);
#486=ELLIPSE('',#10277,0.11254060849194,0.108742931573845);
#487=ELLIPSE('',#10285,0.0694099985395438,0.0599094462298757);
#488=ELLIPSE('',#10286,0.138556662637378,0.119815564117158);
#489=ELLIPSE('',#10291,0.0693000182697834,0.0597453527106058);
#490=B_SPLINE_CURVE_WITH_KNOTS('',3,(#13238,#13239,#13240,#13241),
 .UNSPECIFIED.,.F.,.F.,(4,4),(0.394864882524291,0.484810313459459),
 .UNSPECIFIED.);
#491=B_SPLINE_CURVE_WITH_KNOTS('',3,(#13248,#13249,#13250,#13251,#13252,
#13253,#13254,#13255,#13256,#13257,#13258,#13259,#13260,#13261,#13262,#13263,
#13264,#13265,#13266,#13267,#13268,#13269,#13270,#13271,#13272,#13273,#13274,
#13275,#13276,#13277,#13278,#13279,#13280,#13281),.UNSPECIFIED.,.F.,.F.,
(4,1,1,1,1,1,1,1,1,1,1,1,1,1,1,1,1,1,1,1,1,1,1,1,1,1,1,1,1,1,1,4),(-12.272421221397,
-11.8341204634899,-11.3958197055829,-10.9575189476759,-10.6287933792456,
-10.5192181897688,-9.93481717922612,-9.64261667395476,-9.35041616868341,
-9.05821566341205,-8.76601515814069,-8.18161414759798,-7.59721313705527,
-7.30501263178391,-7.01281212651256,-6.42841111596984,-5.84401010542713,
-5.55180960015577,-5.25960909488442,-5.11350884224874,-4.96740858961306,
-4.6752080843417,-4.09080707379899,-4.01775694748115,-3.50640606325628,
-2.62980454744221,-2.19150378953517,-1.75320303162814,-1.3149022737211,
-0.876601515814069,-0.438300757907035,0.),.UNSPECIFIED.);
#492=B_SPLINE_CURVE_WITH_KNOTS('',3,(#13289,#13290,#13291,#13292),
 .UNSPECIFIED.,.F.,.F.,(4,4),(-1.01772858153936,-0.900201355715508),
 .UNSPECIFIED.);
#493=B_SPLINE_CURVE_WITH_KNOTS('',3,(#13294,#13295,#13296,#13297),
 .UNSPECIFIED.,.F.,.F.,(4,4),(-0.195956842698031,-5.68173586430139E-15),
 .UNSPECIFIED.);
#494=B_SPLINE_CURVE_WITH_KNOTS('',3,(#13299,#13300,#13301,#13302,#13303,
#13304),.UNSPECIFIED.,.F.,.F.,(4,2,4),(-0.531787427886525,-0.530925715886322,
0.),.UNSPECIFIED.);
#495=B_SPLINE_CURVE_WITH_KNOTS('',3,(#13308,#13309,#13310,#13311,#13312,
#13313),.UNSPECIFIED.,.F.,.F.,(4,2,4),(0.,0.0240503814822642,0.0482649912255638),
 .UNSPECIFIED.);
#496=B_SPLINE_CURVE_WITH_KNOTS('',3,(#13315,#13316,#13317,#13318,#13319),
 .UNSPECIFIED.,.F.,.F.,(4,1,4),(0.,0.0699088059566157,0.0984547839530403),
 .UNSPECIFIED.);
#497=B_SPLINE_CURVE_WITH_KNOTS('',5,(#13321,#13322,#13323,#13324,#13325,
#13326,#13327,#13328,#13329,#13330,#13331,#13332,#13333,#13334,#13335,#13336,
#13337,#13338,#13339,#13340,#13341,#13342,#13343,#13344,#13345,#13346,#13347,
#13348,#13349,#13350,#13351,#13352,#13353,#13354,#13355,#13356,#13357,#13358,
#13359,#13360,#13361,#13362,#13363,#13364,#13365,#13366,#13367,#13368,#13369,
#13370,#13371,#13372,#13373,#13374,#13375,#13376,#13377,#13378,#13379,#13380,
#13381,#13382,#13383,#13384,#13385,#13386,#13387,#13388,#13389),
 .UNSPECIFIED.,.F.,.F.,(6,1,1,1,1,1,1,1,1,1,1,1,1,1,1,1,1,1,1,1,1,1,1,1,
1,1,1,1,1,1,1,1,1,1,1,1,1,1,1,1,1,1,1,1,1,1,1,1,1,1,1,1,1,1,1,1,1,1,1,1,
1,1,1,1,6),(-0.934439937517936,-0.932000000000001,-0.928000000000001,-0.924000000000001,
-0.920000000000001,-0.916000000000001,-0.912000000000001,-0.908000000000001,
-0.904000000000001,-0.900000000000001,-0.896000000000001,-0.892000000000001,
-0.888000000000001,-0.884000000000001,-0.880000000000001,-0.876000000000001,
-0.872000000000001,-0.868000000000001,-0.864000000000001,-0.860000000000001,
-0.856000000000001,-0.852000000000001,-0.848000000000001,-0.844000000000001,
-0.840000000000001,-0.836000000000001,-0.832000000000001,-0.828000000000001,
-0.824000000000001,-0.820000000000001,-0.816000000000001,-0.812000000000001,
-0.808000000000001,-0.804000000000001,-0.800000000000001,-0.796000000000001,
-0.792000000000001,-0.788000000000001,-0.784000000000001,-0.780000000000001,
-0.776000000000001,-0.772000000000001,-0.768000000000001,-0.764000000000001,
-0.760000000000001,-0.756000000000001,-0.752000000000001,-0.748000000000001,
-0.744000000000001,-0.740000000000001,-0.736000000000001,-0.732000000000001,
-0.728000000000001,-0.724000000000001,-0.720000000000001,-0.716000000000001,
-0.712000000000001,-0.708000000000001,-0.704000000000001,-0.700000000000001,
-0.696000000000001,-0.692000000000001,-0.688000000000001,-0.684,-0.681561309195619),
 .UNSPECIFIED.);
#498=B_SPLINE_CURVE_WITH_KNOTS('',5,(#13391,#13392,#13393,#13394,#13395,
#13396,#13397),.UNSPECIFIED.,.F.,.F.,(6,1,6),(-0.681561309195566,-0.68,
-0.679861520205026),.UNSPECIFIED.);
#499=B_SPLINE_CURVE_WITH_KNOTS('',3,(#13398,#13399,#13400,#13401,#13402,
#13403),.UNSPECIFIED.,.F.,.F.,(4,2,4),(-0.260568044992996,-0.115264054870948,
0.),.UNSPECIFIED.);
#500=B_SPLINE_CURVE_WITH_KNOTS('',3,(#13423,#13424,#13425,#13426,#13427,
#13428,#13429),.UNSPECIFIED.,.F.,.F.,(4,3,4),(0.584503639029328,0.623122512964242,
0.74773332064937),.UNSPECIFIED.);
#501=B_SPLINE_CURVE_WITH_KNOTS('',3,(#13433,#13434,#13435,#13436),
 .UNSPECIFIED.,.F.,.F.,(4,4),(-0.0543233651499556,0.),.UNSPECIFIED.);
#502=B_SPLINE_CURVE_WITH_KNOTS('',3,(#13437,#13438,#13439,#13440,#13441,
#13442,#13443,#13444,#13445,#13446,#13447,#13448,#13449,#13450,#13451,#13452,
#13453,#13454,#13455,#13456,#13457,#13458,#13459,#13460,#13461,#13462,#13463,
#13464,#13465,#13466,#13467,#13468,#13469,#13470,#13471),.UNSPECIFIED.,
 .F.,.F.,(4,1,1,1,1,1,1,1,1,1,1,1,1,1,1,1,1,1,1,1,1,1,1,1,1,1,1,1,1,1,1,
1,4),(-12.1338940883735,-11.7005407280745,-11.2671873677754,-10.4004806471773,
-9.82267616677859,-9.24487168637985,-8.66706720598111,-8.08926272558237,
-7.800360485383,-7.65590936528331,-7.51145824518363,-7.36700712508394,-7.22255600498426,
-6.93365376478489,-6.64475152458552,-6.35584928438614,-6.06694704418677,
-5.77804480398741,-5.20024032358866,-4.91133808338929,-4.62243584318992,
-4.04463136279118,-3.46682688239244,-3.25015020224292,-3.03347352209339,
-2.60012016179433,-2.49178182171957,-2.16676680149528,-1.73341344119622,
-1.30006008089717,-0.866706720598111,-0.433353360299055,0.),
 .UNSPECIFIED.);
#503=B_SPLINE_CURVE_WITH_KNOTS('',3,(#13479,#13480,#13481,#13482,#13483,
#13484,#13485),.UNSPECIFIED.,.F.,.F.,(4,3,4),(0.489041562207919,0.588820757539051,
0.610492150702822),.UNSPECIFIED.);
#504=B_SPLINE_CURVE_WITH_KNOTS('',3,(#13487,#13488,#13489,#13490,#13491,
#13492),.UNSPECIFIED.,.F.,.F.,(4,1,1,4),(0.,0.0638374291107252,0.12767485822145,
0.141538528407714),.UNSPECIFIED.);
#505=B_SPLINE_CURVE_WITH_KNOTS('',5,(#13494,#13495,#13496,#13497,#13498,
#13499,#13500,#13501,#13502,#13503,#13504,#13505,#13506,#13507,#13508,#13509,
#13510,#13511,#13512,#13513,#13514,#13515,#13516,#13517,#13518,#13519,#13520,
#13521,#13522,#13523,#13524,#13525,#13526,#13527,#13528,#13529,#13530,#13531,
#13532,#13533,#13534,#13535,#13536,#13537,#13538,#13539,#13540,#13541,#13542,
#13543,#13544,#13545,#13546,#13547,#13548,#13549,#13550,#13551,#13552,#13553,
#13554,#13555,#13556,#13557,#13558,#13559,#13560),.UNSPECIFIED.,.F.,.F.,
(6,1,1,1,1,1,1,1,1,1,1,1,1,1,1,1,1,1,1,1,1,1,1,1,1,1,1,1,1,1,1,1,1,1,1,
1,1,1,1,1,1,1,1,1,1,1,1,1,1,1,1,1,1,1,1,1,1,1,1,1,1,1,6),(-0.304944691462234,
-0.304,-0.3,-0.296,-0.292,-0.288,-0.284,-0.28,-0.276,-0.272,-0.268,-0.264,
-0.26,-0.256,-0.252,-0.248,-0.244,-0.24,-0.236,-0.232,-0.228,-0.224,-0.22,
-0.216,-0.212,-0.208,-0.204,-0.2,-0.196,-0.192,-0.188,-0.184,-0.18,-0.176,
-0.172,-0.168,-0.164,-0.16,-0.156,-0.152,-0.148,-0.144,-0.14,-0.136,-0.132,
-0.128,-0.124,-0.12,-0.116,-0.112,-0.108,-0.104,-0.1,-0.0960000000000001,
-0.0920000000000001,-0.0880000000000001,-0.084,-0.08,-0.076,-0.072,-0.068,
-0.064,-0.0619278530721094),.UNSPECIFIED.);
#506=B_SPLINE_CURVE_WITH_KNOTS('',3,(#13562,#13563,#13564,#13565,#13566,
#13567),.UNSPECIFIED.,.F.,.F.,(4,2,4),(-0.0398334813165403,-0.0199277813067177,
-9.94871254822449E-10),.UNSPECIFIED.);
#507=B_SPLINE_CURVE_WITH_KNOTS('',3,(#13569,#13570,#13571,#13572,#13573,
#13574),.UNSPECIFIED.,.F.,.F.,(4,2,4),(2.70147232916989E-5,0.0170939199782327,
0.035271687213346),.UNSPECIFIED.);
#508=B_SPLINE_CURVE_WITH_KNOTS('',3,(#13576,#13577,#13578,#13579,#13580,
#13581,#13582,#13583,#13584,#13585,#13586,#13587,#13588,#13589,#13590,#13591,
#13592,#13593,#13594,#13595),.UNSPECIFIED.,.F.,.F.,(4,2,2,2,2,2,2,2,2,4),
(1.63651820619147E-6,0.010862670932703,0.0337514199363196,0.0421677436560315,
0.0461502331381883,0.0493656606269703,0.0531827874377784,0.0608034042333055,
0.0815457243745407,0.0967454812796038),.UNSPECIFIED.);
#509=B_SPLINE_CURVE_WITH_KNOTS('',3,(#13597,#13598,#13599,#13600,#13601,
#13602),.UNSPECIFIED.,.F.,.F.,(4,2,4),(8.18815340054483E-6,0.00711074921072509,
0.0142181038164433),.UNSPECIFIED.);
#510=B_SPLINE_CURVE_WITH_KNOTS('',3,(#13604,#13605,#13606,#13607,#13608,
#13609),.UNSPECIFIED.,.F.,.F.,(4,2,4),(1.21976025657623E-6,0.00359236891011489,
0.00724827734012079),.UNSPECIFIED.);
#511=B_SPLINE_CURVE_WITH_KNOTS('',3,(#13611,#13612,#13613,#13614,#13615,
#13616),.UNSPECIFIED.,.F.,.F.,(4,2,4),(1.24265944092431E-5,0.0394422622090392,
0.0830428857918921),.UNSPECIFIED.);
#512=B_SPLINE_CURVE_WITH_KNOTS('',3,(#13618,#13619,#13620,#13621,#13622,
#13623,#13624,#13625),.UNSPECIFIED.,.F.,.F.,(4,2,2,4),(-0.000597804895778801,
0.,0.0849714808180455,0.169669487930669),.UNSPECIFIED.);
#513=B_SPLINE_CURVE_WITH_KNOTS('',3,(#13642,#13643,#13644,#13645,#13646,
#13647,#13648,#13649,#13650,#13651,#13652,#13653,#13654,#13655,#13656,#13657,
#13658,#13659,#13660),.UNSPECIFIED.,.F.,.F.,(4,3,3,3,3,3,4),(0.,0.057820470339356,
0.0749307800866031,0.0860134923791381,0.116509264080236,0.148377898752131,
0.154536834355727),.UNSPECIFIED.);
#514=B_SPLINE_CURVE_WITH_KNOTS('',3,(#13668,#13669,#13670,#13671,#13672,
#13673,#13674,#13675,#13676,#13677,#13678,#13679,#13680,#13681,#13682,#13683,
#13684,#13685,#13686,#13687,#13688,#13689,#13690,#13691,#13692,#13693,#13694,
#13695),.UNSPECIFIED.,.F.,.F.,(4,3,3,3,3,3,3,3,3,4),(-0.221165784147146,
-0.203605965934998,-0.1863734624514,-0.168207576681715,-0.143931298953183,
-0.100603143960458,-0.064904744585576,-0.048733613964838,-0.0209494131580949,
-9.99999236175762E-7),.UNSPECIFIED.);
#515=B_SPLINE_CURVE_WITH_KNOTS('',3,(#14221,#14222,#14223,#14224,#14225,
#14226,#14227,#14228,#14229,#14230,#14231,#14232,#14233,#14234,#14235,#14236,
#14237,#14238,#14239,#14240,#14241,#14242,#14243,#14244,#14245,#14246,#14247,
#14248,#14249,#14250,#14251,#14252,#14253,#14254,#14255),.UNSPECIFIED.,
 .F.,.F.,(4,1,1,1,1,1,1,1,1,1,1,1,1,1,1,1,1,1,1,1,1,1,1,1,1,1,1,1,1,1,1,
1,4),(0.,0.433353360299055,0.866706720598111,1.30006008089717,1.73341344119622,
2.16676680149528,2.49178182171957,2.60012016179433,3.03347352209339,3.25015020224292,
3.46682688239244,4.04463136279118,4.62243584318992,4.91133808338929,5.20024032358866,
5.77804480398741,6.06694704418677,6.35584928438614,6.64475152458552,6.93365376478489,
7.22255600498426,7.36700712508394,7.51145824518363,7.65590936528331,7.800360485383,
8.08926272558237,8.66706720598111,9.24487168637985,9.82267616677859,10.4004806471773,
11.2671873677754,11.7005407280745,12.1338940883735),.UNSPECIFIED.);
#516=B_SPLINE_CURVE_WITH_KNOTS('',3,(#14257,#14258,#14259,#14260,#14261,
#14262,#14263,#14264),.UNSPECIFIED.,.F.,.F.,(4,1,1,1,1,4),(-0.119541952220061,
-0.117697345682202,-0.115852739144342,-0.112163526068624,-0.104785099917186,
-0.0937174606900304),.UNSPECIFIED.);
#517=B_SPLINE_CURVE_WITH_KNOTS('',3,(#14268,#14269,#14270,#14271),
 .UNSPECIFIED.,.F.,.F.,(4,4),(-0.227650451044217,0.),.UNSPECIFIED.);
#518=B_SPLINE_CURVE_WITH_KNOTS('',3,(#14478,#14479,#14480,#14481,#14482,
#14483),.UNSPECIFIED.,.F.,.F.,(4,2,4),(0.0543371154509674,0.152867184867239,
0.15340523472588),.UNSPECIFIED.);
#519=B_SPLINE_CURVE_WITH_KNOTS('',3,(#14484,#14485,#14486,#14487,#14488,
#14489,#14490,#14491,#14492,#14493,#14494,#14495,#14496,#14497,#14498,#14499,
#14500,#14501,#14502),.UNSPECIFIED.,.F.,.F.,(4,3,3,3,3,3,4),(-0.15340523472588,
-0.152867184867239,-0.121542670578485,-0.0960576486891604,-0.0776465306498218,
-0.0660266035836145,-0.05433711858811),.UNSPECIFIED.);
#520=B_SPLINE_CURVE_WITH_KNOTS('',3,(#14525,#14526,#14527,#14528,#14529,
#14530,#14531,#14532,#14533,#14534,#14535,#14536,#14537),.UNSPECIFIED.,
 .F.,.F.,(4,3,3,3,4),(0.,0.0223793464434253,0.0433077332578928,0.0522216264092524,
0.0543233530776371),.UNSPECIFIED.);
#521=B_SPLINE_CURVE_WITH_KNOTS('',3,(#14589,#14590,#14591,#14592,#14593,
#14594,#14595,#14596),.UNSPECIFIED.,.F.,.F.,(4,1,1,1,1,4),(0.0937174606900304,
0.104785099917186,0.112163526068624,0.115852739144342,0.117697345682202,
0.119541952220061),.UNSPECIFIED.);
#522=B_SPLINE_CURVE_WITH_KNOTS('',3,(#14629,#14630,#14631,#14632,#14633,
#14634),.UNSPECIFIED.,.F.,.F.,(4,1,1,4),(1.65498255800438E-15,0.129082836972258,
0.215138061620429,0.301190240731281),.UNSPECIFIED.);
#523=B_SPLINE_CURVE_WITH_KNOTS('',3,(#14660,#14661,#14662,#14663,#14664,
#14665,#14666),.UNSPECIFIED.,.F.,.F.,(4,3,4),(0.,0.150132901020185,0.227650451044083),
 .UNSPECIFIED.);
#524=B_SPLINE_CURVE_WITH_KNOTS('',3,(#14689,#14690,#14691,#14692),
 .UNSPECIFIED.,.F.,.F.,(4,4),(6.03465648009666E-14,0.0429068684110201),
 .UNSPECIFIED.);
#525=B_SPLINE_CURVE_WITH_KNOTS('',3,(#14734,#14735,#14736,#14737,#14738,
#14739,#14740,#14741,#14742,#14743,#14744,#14745,#14746,#14747,#14748,#14749,
#14750,#14751,#14752,#14753,#14754,#14755,#14756,#14757,#14758,#14759,#14760,
#14761,#14762,#14763,#14764,#14765,#14766,#14767,#14768,#14769,#14770,#14771,
#14772,#14773),.UNSPECIFIED.,.F.,.F.,(4,3,3,3,3,3,3,3,3,3,3,3,3,4),(-0.000426969481637764,
-5.70290342727375E-17,0.0136974853077621,0.0169318002365105,0.0215321188993139,
0.030659423657535,0.0358425712401134,0.0361428073033054,0.0487839324257399,
0.0601713945215638,0.0711682787397989,0.071687262555713,0.075441369769445,
0.0785208370583627),.UNSPECIFIED.);
#526=B_SPLINE_CURVE_WITH_KNOTS('',3,(#14799,#14800,#14801,#14802,#14803,
#14804,#14805,#14806,#14807,#14808,#14809,#14810,#14811,#14812,#14813,#14814,
#14815,#14816,#14817,#14818,#14819,#14820),.UNSPECIFIED.,.F.,.F.,(4,3,3,
3,3,3,3,4),(9.99999753309056E-7,0.212329740918838,0.392771135232247,0.447248810346286,
0.622477441204398,0.70601051205627,0.853321790119657,0.891484214299584),
 .UNSPECIFIED.);
#527=B_SPLINE_CURVE_WITH_KNOTS('',3,(#14825,#14826,#14827,#14828),
 .UNSPECIFIED.,.F.,.F.,(4,4),(0.0423193643606908,0.252933252504432),
 .UNSPECIFIED.);
#528=B_SPLINE_CURVE_WITH_KNOTS('',3,(#14850,#14851,#14852,#14853),
 .UNSPECIFIED.,.F.,.F.,(4,4),(0.,0.224615521635083),.UNSPECIFIED.);
#529=B_SPLINE_CURVE_WITH_KNOTS('',3,(#14876,#14877,#14878,#14879),
 .UNSPECIFIED.,.F.,.F.,(4,4),(-0.127798241063314,-0.0854459382956349),
 .UNSPECIFIED.);
#530=B_SPLINE_CURVE_WITH_KNOTS('',3,(#14923,#14924,#14925,#14926,#14927,
#14928,#14929),.UNSPECIFIED.,.F.,.F.,(4,1,1,1,4),(0.,0.0328013253035665,
0.065602650607133,0.109337751011888,0.137794282289288),.UNSPECIFIED.);
#531=B_SPLINE_CURVE_WITH_KNOTS('',3,(#14969,#14970,#14971,#14972),
 .UNSPECIFIED.,.F.,.F.,(4,4),(0.,0.17884239607127),.UNSPECIFIED.);
#532=B_SPLINE_CURVE_WITH_KNOTS('',3,(#14991,#14992,#14993,#14994),
 .UNSPECIFIED.,.F.,.F.,(4,4),(-0.0801298062963358,0.),.UNSPECIFIED.);
#533=B_SPLINE_CURVE_WITH_KNOTS('',3,(#15101,#15102,#15103,#15104,#15105,
#15106,#15107,#15108,#15109,#15110,#15111,#15112,#15113,#15114,#15115,#15116,
#15117,#15118,#15119,#15120,#15121,#15122,#15123,#15124,#15125,#15126,#15127,
#15128,#15129,#15130,#15131,#15132,#15133,#15134,#15135,#15136,#15137,#15138,
#15139,#15140,#15141,#15142,#15143,#15144,#15145,#15146,#15147,#15148,#15149,
#15150,#15151,#15152,#15153,#15154,#15155,#15156,#15157,#15158,#15159,#15160,
#15161,#15162,#15163,#15164,#15165,#15166,#15167,#15168,#15169,#15170,#15171,
#15172,#15173,#15174,#15175,#15176,#15177,#15178,#15179,#15180,#15181,#15182,
#15183,#15184,#15185,#15186,#15187,#15188,#15189,#15190,#15191,#15192,#15193,
#15194,#15195,#15196,#15197,#15198,#15199,#15200,#15201,#15202,#15203,#15204,
#15205,#15206,#15207,#15208,#15209,#15210,#15211,#15212,#15213,#15214,#15215,
#15216,#15217,#15218,#15219,#15220,#15221,#15222,#15223,#15224,#15225,#15226,
#15227,#15228,#15229,#15230,#15231,#15232,#15233,#15234,#15235,#15236,#15237,
#15238,#15239,#15240,#15241,#15242,#15243,#15244,#15245,#15246,#15247,#15248,
#15249,#15250,#15251,#15252,#15253,#15254,#15255,#15256,#15257,#15258,#15259,
#15260,#15261,#15262,#15263,#15264,#15265,#15266,#15267,#15268,#15269,#15270,
#15271,#15272,#15273,#15274,#15275,#15276,#15277,#15278,#15279,#15280,#15281,
#15282,#15283,#15284,#15285,#15286,#15287,#15288,#15289,#15290,#15291,#15292,
#15293,#15294,#15295,#15296,#15297,#15298,#15299,#15300,#15301,#15302,#15303,
#15304,#15305,#15306,#15307,#15308,#15309,#15310,#15311,#15312,#15313,#15314,
#15315,#15316,#15317,#15318,#15319,#15320,#15321,#15322,#15323),
 .UNSPECIFIED.,.F.,.F.,(4,3,3,3,3,3,3,3,3,3,3,3,3,3,3,3,3,3,3,3,3,3,3,3,
3,3,3,3,3,3,3,3,3,3,3,3,3,3,3,3,3,3,3,3,3,3,3,3,3,3,3,3,3,3,3,3,3,3,3,3,
3,3,3,3,3,3,3,3,3,3,3,3,3,3,4),(0.0143556209070032,0.0918173375013859,0.137368681256099,
0.164850487143807,0.236118654939979,0.29915612965247,0.361701124093769,
0.423757485765995,0.463705909920997,0.516706771668045,0.570541124923225,
0.604256389891492,0.685039858234251,0.766114259399882,0.848927080753196,
0.893877183497122,0.978785410078009,1.06778327179008,1.16126984103901,1.21538171189569,
1.333822502657,1.45799045338518,1.58635211001713,1.69368579518043,1.76887432285106,
1.82502584109974,1.99446359366836,2.1682652962319,2.34746509975619,2.40944331829074,
2.63945041210237,2.87599055478919,3.12224465593178,3.38274453001889,3.66483085961975,
4.00177577901762,4.34319730999942,4.59080469175813,4.73545737518022,4.788086707876,
5.04860488829482,5.29050385726843,5.52038017836126,5.74206280076628,5.90224108935206,
6.08765479241645,6.25857458098853,6.42517545732593,6.52288884673658,6.57920791189009,
6.70933184189355,6.83569015966474,6.95707192851147,7.05644314801653,7.12291710476878,
7.21605540565365,7.30472824136214,7.38580967032176,7.44201203358028,7.52405452487865,
7.60444481353644,7.68453791087736,7.71803570888323,7.77141664614894,7.82397351603657,
7.87085605861451,7.92952553290749,7.9764492685614,8.00862146467435,8.0699558254521,
8.12869572362376,8.15667568402911,8.21796501853068,8.28865197779449,8.30491541813874),
 .UNSPECIFIED.);
#534=B_SPLINE_CURVE_WITH_KNOTS('',3,(#15326,#15327,#15328,#15329,#15330,
#15331,#15332,#15333,#15334,#15335,#15336,#15337,#15338,#15339,#15340,#15341,
#15342,#15343,#15344,#15345,#15346),.UNSPECIFIED.,.F.,.F.,(4,1,1,1,1,1,
1,1,1,1,1,1,1,1,1,1,1,1,4),(-8.30491541813874,-8.15661335710055,-8.00831129606236,
-7.86000923502417,-7.71170717398598,-7.41510305190959,-7.11849892983321,
-6.52529068568044,-5.93208244152767,-4.74566595322214,-2.37283297661107,
-1.7796247324583,-1.18641648830553,-0.889812366229151,-0.593208244152767,
-0.444906183114576,-0.296604122076384,-0.148302061038192,0.),
 .UNSPECIFIED.);
#535=B_SPLINE_CURVE_WITH_KNOTS('',3,(#15432,#15433,#15434,#15435,#15436,
#15437,#15438,#15439,#15440,#15441,#15442,#15443,#15444,#15445,#15446,#15447,
#15448,#15449,#15450,#15451,#15452,#15453,#15454,#15455,#15456,#15457,#15458,
#15459,#15460,#15461,#15462,#15463,#15464,#15465,#15466,#15467,#15468,#15469,
#15470,#15471,#15472,#15473,#15474,#15475,#15476,#15477,#15478,#15479,#15480,
#15481,#15482,#15483,#15484,#15485,#15486,#15487,#15488,#15489,#15490,#15491,
#15492,#15493,#15494,#15495,#15496,#15497,#15498,#15499,#15500,#15501,#15502,
#15503,#15504,#15505,#15506,#15507,#15508,#15509,#15510,#15511,#15512,#15513,
#15514,#15515,#15516,#15517,#15518,#15519,#15520,#15521,#15522,#15523,#15524,
#15525,#15526,#15527,#15528,#15529,#15530,#15531,#15532,#15533,#15534,#15535,
#15536,#15537,#15538,#15539,#15540,#15541,#15542,#15543,#15544,#15545,#15546,
#15547,#15548,#15549,#15550,#15551,#15552,#15553,#15554,#15555,#15556,#15557,
#15558,#15559,#15560,#15561,#15562,#15563,#15564,#15565,#15566,#15567,#15568,
#15569,#15570,#15571,#15572,#15573,#15574,#15575,#15576,#15577,#15578,#15579,
#15580,#15581,#15582,#15583,#15584,#15585,#15586,#15587,#15588,#15589,#15590,
#15591,#15592,#15593,#15594,#15595,#15596,#15597,#15598,#15599,#15600,#15601,
#15602,#15603,#15604,#15605,#15606,#15607,#15608,#15609,#15610,#15611,#15612,
#15613,#15614,#15615,#15616,#15617,#15618,#15619,#15620,#15621,#15622,#15623,
#15624,#15625,#15626,#15627,#15628,#15629,#15630,#15631,#15632,#15633,#15634,
#15635,#15636,#15637,#15638,#15639,#15640,#15641,#15642,#15643,#15644,#15645,
#15646,#15647,#15648,#15649,#15650,#15651,#15652,#15653,#15654),
 .UNSPECIFIED.,.F.,.F.,(4,3,3,3,3,3,3,3,3,3,3,3,3,3,3,3,3,3,3,3,3,3,3,3,
3,3,3,3,3,3,3,3,3,3,3,3,3,3,3,3,3,3,3,3,3,3,3,3,3,3,3,3,3,3,3,3,3,3,3,3,
3,3,3,3,3,3,3,3,3,3,3,3,3,3,4),(0.,0.0796002531402428,0.143860527866794,
0.179459274819612,0.242939400939292,0.289836237203638,0.325717441475301,
0.388054925667984,0.442922087934823,0.495706533831402,0.549137052626795,
0.589808904685002,0.633776280374242,0.714472650605738,0.796031244337957,
0.863874470471167,0.933235621193325,1.02001599391656,1.11110468536068,1.19249198525964,
1.30962863517608,1.43279082776966,1.56039482576159,1.69164843617825,1.76643789090045,
1.82645895882964,1.99593365718847,2.16977738887537,2.34903131982582,2.41009920440689,
2.64012149822895,2.87668451600587,3.12297220656693,3.38352156197452,3.66568523716309,
4.00272734179774,4.34406360830132,4.59161684641616,4.73716379055164,4.78741151509335,
5.04798742679384,5.28992117381758,5.51982022830723,5.74151786718094,5.9017302141158,
6.08789567836694,6.25881116250794,6.42540866186584,6.52355479195162,6.57973305697088,
6.70984225463914,6.83618333626226,6.95754104745397,7.05650826390725,7.12298174141615,
7.21611710010299,7.30478715182435,7.38589019760746,7.44197485199613,7.52401831132503,
7.6044090168049,7.68450183493196,7.71800683849413,7.77138849884627,7.82394576594535,
7.87083250800939,7.92950086544489,7.97642768453163,8.00860889412839,8.06994218027327,
8.12868548973964,8.15666640215728,8.21795386255756,8.28863888262294,8.30491541813876),
 .UNSPECIFIED.);
#536=B_SPLINE_CURVE_WITH_KNOTS('',3,(#15798,#15799,#15800,#15801),
 .UNSPECIFIED.,.F.,.F.,(4,4),(2.65444323739948E-13,0.080129806296636),
 .UNSPECIFIED.);
#537=B_SPLINE_CURVE_WITH_KNOTS('',3,(#15830,#15831,#15832,#15833,#15834,
#15835),.UNSPECIFIED.,.F.,.F.,(4,1,1,4),(-0.140796741914463,-0.0804552810939789,
-0.0402276405469894,0.),.UNSPECIFIED.);
#538=B_SPLINE_CURVE_WITH_KNOTS('',3,(#15838,#15839,#15840,#15841,#15842,
#15843,#15844,#15845,#15846,#15847,#15848,#15849,#15850,#15851,#15852,#15853,
#15854,#15855,#15856,#15857,#15858,#15859),.UNSPECIFIED.,.F.,.F.,(4,3,3,
3,3,3,3,4),(-0.116549789703214,-0.104681178539138,-0.0961709462162922,-0.0773146819780265,
-0.0757921027293709,-0.0712796665105129,-0.0536565317120064,-0.0452352637954112),
 .UNSPECIFIED.);
#539=B_SPLINE_CURVE_WITH_KNOTS('',3,(#15879,#15880,#15881,#15882),
 .UNSPECIFIED.,.F.,.F.,(4,4),(-0.0800719510115295,0.),.UNSPECIFIED.);
#540=B_SPLINE_CURVE_WITH_KNOTS('',3,(#15950,#15951,#15952,#15953,#15954,
#15955,#15956),.UNSPECIFIED.,.F.,.F.,(4,3,4),(0.,0.0137497525298979,0.0275089565102414),
 .UNSPECIFIED.);
#541=B_SPLINE_CURVE_WITH_KNOTS('',3,(#15957,#15958,#15959,#15960),
 .UNSPECIFIED.,.F.,.F.,(4,4),(0.00882828078135349,0.428984955288124),
 .UNSPECIFIED.);
#542=B_SPLINE_CURVE_WITH_KNOTS('',3,(#16003,#16004,#16005,#16006,#16007,
#16008,#16009,#16010),.UNSPECIFIED.,.F.,.F.,(4,1,1,1,1,4),(0.0418199835477882,
0.170057059808597,0.209506993669976,0.248956927531355,0.268681894462045,
0.288323933546714),.UNSPECIFIED.);
#543=B_SPLINE_CURVE_WITH_KNOTS('',3,(#16013,#16014,#16015,#16016,#16017,
#16018,#16019,#16020,#16021,#16022,#16023,#16024,#16025,#16026,#16027,#16028,
#16029,#16030,#16031,#16032,#16033,#16034,#16035,#16036,#16037,#16038,#16039,
#16040,#16041,#16042,#16043,#16044,#16045,#16046,#16047,#16048,#16049,#16050,
#16051,#16052,#16053,#16054,#16055,#16056,#16057,#16058,#16059,#16060,#16061,
#16062,#16063,#16064,#16065,#16066,#16067,#16068,#16069,#16070,#16071,#16072,
#16073),.UNSPECIFIED.,.F.,.F.,(4,3,3,3,3,3,3,3,3,3,3,3,3,3,3,3,3,3,3,3,
4),(-0.0442526796497479,-0.0442281707822011,-0.0442036619146543,-0.0441546441795607,
-0.0440566087093734,-0.0438605377689989,-0.0431195460395093,-0.0422129105337495,
-0.0415351353283317,-0.0398096658242585,-0.0373324461243466,-0.0332891307954845,
-0.0254070365801755,-0.0151992737645416,-0.00246712194872464,0.00377091893863574,
0.0240422992970927,0.064119853096241,0.133396539450971,0.205795596167866,
0.226989045266928),.UNSPECIFIED.);
#544=B_SPLINE_CURVE_WITH_KNOTS('',3,(#16595,#16596,#16597,#16598,#16599,
#16600,#16601),.UNSPECIFIED.,.F.,.F.,(4,3,4),(0.0271515251943673,0.0836066639604027,
0.140061802726436),.UNSPECIFIED.);
#545=B_SPLINE_CURVE_WITH_KNOTS('',5,(#16603,#16604,#16605,#16606,#16607,
#16608),.UNSPECIFIED.,.F.,.F.,(6,6),(0.648016352593037,0.649373679600467),
 .UNSPECIFIED.);
#546=B_SPLINE_CURVE_WITH_KNOTS('',3,(#16610,#16611,#16612,#16613,#16614,
#16615,#16616,#16617,#16618,#16619,#16620,#16621,#16622,#16623),
 .UNSPECIFIED.,.F.,.F.,(4,2,2,2,2,2,4),(-0.300128297810014,-0.297956747127101,
-0.285522099406917,-0.254881013502635,-0.225735659999153,-0.194244463145828,
-0.1740900876335),.UNSPECIFIED.);
#547=B_SPLINE_CURVE_WITH_KNOTS('',3,(#16627,#16628,#16629,#16630,#16631,
#16632,#16633,#16634,#16635,#16636,#16637,#16638,#16639,#16640,#16641,#16642),
 .UNSPECIFIED.,.F.,.F.,(4,2,2,2,2,2,2,4),(-0.334017896162169,-0.307673650184263,
-0.27974268303834,-0.254256084112274,-0.232306890768372,-0.212897818769103,
-0.209691850469659,-0.208062418892068),.UNSPECIFIED.);
#548=B_SPLINE_CURVE_WITH_KNOTS('',5,(#16644,#16645,#16646,#16647,#16648,
#16649),.UNSPECIFIED.,.F.,.F.,(6,6),(-0.649373679600467,-0.648016352593037),
 .UNSPECIFIED.);
#549=B_SPLINE_CURVE_WITH_KNOTS('',3,(#16747,#16748,#16749,#16750,#16751,
#16752,#16753,#16754,#16755,#16756,#16757,#16758,#16759,#16760,#16761,#16762,
#16763,#16764,#16765),.UNSPECIFIED.,.F.,.F.,(4,1,1,1,1,1,1,1,1,1,1,1,1,
1,1,1,4),(-2.75290571088706,-2.36172303637955,-2.16491278334792,-1.96810253031629,
-1.77129227728466,-1.67288715076885,-1.57448202425304,-1.44327518889862,
-1.3120683535442,-1.18086151818978,-1.11525810051257,-1.04965468283536,
-1.01685297399675,-0.918447847480937,-0.787241012126518,-0.393620506063259,
0.),.UNSPECIFIED.);
#550=B_SPLINE_CURVE_WITH_KNOTS('',3,(#16768,#16769,#16770,#16771,#16772,
#16773,#16774,#16775,#16776,#16777,#16778,#16779,#16780,#16781,#16782,#16783,
#16784,#16785,#16786,#16787,#16788,#16789,#16790,#16791,#16792,#16793,#16794,
#16795,#16796,#16797,#16798,#16799,#16800,#16801,#16802,#16803,#16804,#16805,
#16806,#16807,#16808,#16809,#16810,#16811,#16812,#16813,#16814,#16815,#16816,
#16817,#16818,#16819,#16820,#16821,#16822,#16823,#16824,#16825,#16826,#16827,
#16828,#16829,#16830,#16831,#16832,#16833,#16834,#16835,#16836,#16837,#16838,
#16839,#16840,#16841,#16842,#16843,#16844,#16845,#16846,#16847,#16848,#16849,
#16850,#16851,#16852,#16853,#16854,#16855,#16856,#16857,#16858,#16859,#16860,
#16861,#16862,#16863,#16864,#16865,#16866,#16867,#16868,#16869,#16870,#16871,
#16872,#16873,#16874,#16875,#16876,#16877,#16878,#16879,#16880,#16881,#16882,
#16883,#16884,#16885,#16886,#16887,#16888,#16889,#16890,#16891,#16892,#16893,
#16894,#16895,#16896,#16897,#16898,#16899,#16900,#16901,#16902,#16903,#16904,
#16905,#16906,#16907,#16908,#16909,#16910,#16911,#16912,#16913,#16914,#16915,
#16916,#16917,#16918,#16919,#16920,#16921,#16922,#16923,#16924,#16925,#16926,
#16927,#16928,#16929,#16930,#16931,#16932,#16933,#16934,#16935,#16936,#16937,
#16938,#16939),.UNSPECIFIED.,.F.,.F.,(4,3,3,3,3,3,3,3,3,3,3,3,3,3,3,3,3,
3,3,3,3,3,3,3,3,3,3,3,3,3,3,3,3,3,3,3,3,3,3,3,3,3,3,3,3,3,3,3,3,3,3,3,3,
3,3,3,3,4),(0.,0.124369445529287,0.240030100192546,0.341233173022898,0.386674939404266,
0.411251254648982,0.491051683172279,0.563259965633032,0.630860010468553,
0.694792605008278,0.755770367876227,0.786749499491396,0.817139299607178,
0.861736210910445,0.904274509743171,0.933198720069145,0.967921430487703,
1.00176688673899,1.03365991619405,1.04965468283536,1.07830325879074,1.1039428236405,
1.123230742087,1.14569030213385,1.16906027640734,1.18086151818978,1.21528836919337,
1.25037899156894,1.28678619044467,1.30975642476343,1.3319781812234,1.37090028685257,
1.41175418522684,1.44539431955843,1.4917123985274,1.53781361798719,1.57586142812643,
1.62639986626241,1.66167935614305,1.68488494942284,1.71866494451513,1.75106115070037,
1.77418615895868,1.83844826443971,1.89630279494469,1.94999284166332,1.99684076151575,
2.05216246141503,2.10981892955224,2.1576446865864,2.20199668451076,2.28010760411423,
2.35258768188503,2.41850715945014,2.51795162746106,2.62227620558227,2.73424605476883,
2.75534354244281),.UNSPECIFIED.);
#551=B_SPLINE_CURVE_WITH_KNOTS('',3,(#16972,#16973,#16974,#16975,#16976),
 .UNSPECIFIED.,.F.,.F.,(4,1,4),(0.,0.0833626696026172,0.166725339205234),
 .UNSPECIFIED.);
#552=B_SPLINE_CURVE_WITH_KNOTS('',3,(#17001,#17002,#17003,#17004),
 .UNSPECIFIED.,.F.,.F.,(4,4),(-0.164730944371734,0.),.UNSPECIFIED.);
#553=B_SPLINE_CURVE_WITH_KNOTS('',3,(#17007,#17008,#17009,#17010),
 .UNSPECIFIED.,.F.,.F.,(4,4),(0.,0.164730944371734),.UNSPECIFIED.);
#554=B_SPLINE_CURVE_WITH_KNOTS('',3,(#17034,#17035,#17036,#17037),
 .UNSPECIFIED.,.F.,.F.,(4,4),(-0.0505768769923026,0.),.UNSPECIFIED.);
#555=B_SPLINE_CURVE_WITH_KNOTS('',3,(#17038,#17039,#17040,#17041),
 .UNSPECIFIED.,.F.,.F.,(4,4),(0.,0.0505769320975467),.UNSPECIFIED.);
#556=B_SPLINE_CURVE_WITH_KNOTS('',3,(#17062,#17063,#17064,#17065),
 .UNSPECIFIED.,.F.,.F.,(4,4),(-0.075415368178403,0.),.UNSPECIFIED.);
#557=B_SPLINE_CURVE_WITH_KNOTS('',3,(#17066,#17067,#17068,#17069),
 .UNSPECIFIED.,.F.,.F.,(4,4),(0.,0.075415368178403),.UNSPECIFIED.);
#558=B_SPLINE_CURVE_WITH_KNOTS('',3,(#17147,#17148,#17149,#17150),
 .UNSPECIFIED.,.F.,.F.,(4,4),(-0.499612937204198,-0.0795665830105256),
 .UNSPECIFIED.);
#559=B_SPLINE_CURVE_WITH_KNOTS('',5,(#17151,#17152,#17153,#17154,#17155,
#17156,#17157,#17158,#17159,#17160,#17161,#17162,#17163,#17164,#17165,#17166,
#17167,#17168,#17169,#17170,#17171,#17172,#17173,#17174),.UNSPECIFIED.,
 .F.,.F.,(6,1,1,1,1,1,1,1,1,1,1,1,1,1,1,1,1,1,1,6),(-0.648016352593037,
-0.648,-0.644,-0.64,-0.636,-0.632,-0.628,-0.624,-0.62,-0.616,-0.612,-0.608,
-0.604,-0.6,-0.596,-0.592,-0.588,-0.584,-0.58,-0.578475706653789),
 .UNSPECIFIED.);
#560=B_SPLINE_CURVE_WITH_KNOTS('',3,(#17192,#17193,#17194,#17195),
 .UNSPECIFIED.,.F.,.F.,(4,4),(0.0795665875934902,0.50017173665434),
 .UNSPECIFIED.);
#561=B_SPLINE_CURVE_WITH_KNOTS('',3,(#17198,#17199,#17200,#17201,#17202,
#17203),.UNSPECIFIED.,.F.,.F.,(4,2,4),(-0.0146609285082182,-0.00733041182656413,
0.),.UNSPECIFIED.);
#562=B_SPLINE_CURVE_WITH_KNOTS('',3,(#17221,#17222,#17223,#17224),
 .UNSPECIFIED.,.F.,.F.,(4,4),(0.120092046373885,0.541502145499565),
 .UNSPECIFIED.);
#563=B_SPLINE_CURVE_WITH_KNOTS('',3,(#17225,#17226,#17227,#17228,#17229,
#17230,#17231),.UNSPECIFIED.,.F.,.F.,(4,3,4),(0.,0.0172799395456661,0.0241280202161043),
 .UNSPECIFIED.);
#564=B_SPLINE_CURVE_WITH_KNOTS('',3,(#17769,#17770,#17771,#17772,#17773,
#17774,#17775,#17776,#17777,#17778),.UNSPECIFIED.,.F.,.F.,(4,2,2,2,4),(-0.100432637091733,
-0.0783128365433848,-0.0562142474116246,-0.0304582357928518,0.),
 .UNSPECIFIED.);
#565=B_SPLINE_CURVE_WITH_KNOTS('',3,(#18305,#18306,#18307,#18308),
 .UNSPECIFIED.,.F.,.F.,(4,4),(0.302038178795817,0.512484404778385),
 .UNSPECIFIED.);
#566=B_SPLINE_CURVE_WITH_KNOTS('',3,(#18309,#18310,#18311,#18312,#18313,
#18314),.UNSPECIFIED.,.F.,.F.,(4,2,4),(-0.531120307157959,-0.238218417429911,
-9.99999644757388E-7),.UNSPECIFIED.);
#567=B_SPLINE_CURVE_WITH_KNOTS('',3,(#18335,#18336,#18337,#18338),
 .UNSPECIFIED.,.F.,.F.,(4,4),(0.214918350132049,0.48911828449592),
 .UNSPECIFIED.);
#568=B_SPLINE_CURVE_WITH_KNOTS('',3,(#18342,#18343,#18344,#18345),
 .UNSPECIFIED.,.F.,.F.,(4,4),(-0.48911828449592,-0.216907151819261),
 .UNSPECIFIED.);
#569=B_SPLINE_CURVE_WITH_KNOTS('',3,(#18346,#18347,#18348,#18349),
 .UNSPECIFIED.,.F.,.F.,(4,4),(-0.00307307886366898,0.),.UNSPECIFIED.);
#570=B_SPLINE_CURVE_WITH_KNOTS('',3,(#18369,#18370,#18371,#18372),
 .UNSPECIFIED.,.F.,.F.,(4,4),(-0.197269104818139,0.),.UNSPECIFIED.);
#571=B_SPLINE_CURVE_WITH_KNOTS('',3,(#18373,#18374,#18375,#18376),
 .UNSPECIFIED.,.F.,.F.,(4,4),(0.,0.197269104818139),.UNSPECIFIED.);
#572=B_SPLINE_CURVE_WITH_KNOTS('',3,(#18394,#18395,#18396,#18397,#18398,
#18399,#18400,#18401,#18402,#18403),.UNSPECIFIED.,.F.,.F.,(4,3,3,4),(-0.221056240648656,
-0.141998498310432,-0.0700174415183823,-7.01203975429252E-6),
 .UNSPECIFIED.);
#573=B_SPLINE_CURVE_WITH_KNOTS('',3,(#18404,#18405,#18406,#18407),
 .UNSPECIFIED.,.F.,.F.,(4,4),(-6.0267045889705E-5,0.216046193075007),
 .UNSPECIFIED.);
#574=B_SPLINE_CURVE_WITH_KNOTS('',3,(#18433,#18434,#18435,#18436,#18437,
#18438),.UNSPECIFIED.,.F.,.F.,(4,2,4),(0.,0.471468502883735,0.473994966708672),
 .UNSPECIFIED.);
#575=B_SPLINE_CURVE_WITH_KNOTS('',3,(#18440,#18441,#18442,#18443,#18444,
#18445),.UNSPECIFIED.,.F.,.F.,(4,2,4),(-0.473994966708672,-0.471468502883735,
-0.468943296379571),.UNSPECIFIED.);
#576=B_SPLINE_CURVE_WITH_KNOTS('',3,(#18447,#18448,#18449,#18450),
 .UNSPECIFIED.,.F.,.F.,(4,4),(-0.468943296379571,0.),.UNSPECIFIED.);
#577=B_SPLINE_CURVE_WITH_KNOTS('',3,(#18468,#18469,#18470,#18471),
 .UNSPECIFIED.,.F.,.F.,(4,4),(-0.0666641938434966,-1.89854339553983E-15),
 .UNSPECIFIED.);
#578=B_SPLINE_CURVE_WITH_KNOTS('',3,(#18472,#18473,#18474,#18475),
 .UNSPECIFIED.,.F.,.F.,(4,4),(1.89854339553983E-15,0.0666641979607186),
 .UNSPECIFIED.);
#579=B_SPLINE_CURVE_WITH_KNOTS('',3,(#18493,#18494,#18495,#18496,#18497,
#18498),.UNSPECIFIED.,.F.,.F.,(4,2,4),(-0.124627466599506,-0.0741353398935927,
-0.00200197401216558),.UNSPECIFIED.);
#580=B_SPLINE_CURVE_WITH_KNOTS('',3,(#18500,#18501,#18502,#18503,#18504,
#18505),.UNSPECIFIED.,.F.,.F.,(4,2,4),(0.,0.0142795390469111,0.0283526878042237),
 .UNSPECIFIED.);
#581=B_SPLINE_CURVE_WITH_KNOTS('',3,(#18572,#18573,#18574,#18575,#18576,
#18577,#18578,#18579,#18580,#18581,#18582,#18583,#18584,#18585,#18586,#18587,
#18588,#18589,#18590,#18591,#18592,#18593,#18594,#18595,#18596),
 .UNSPECIFIED.,.F.,.F.,(4,3,3,3,3,3,3,3,4),(-0.328233327143732,-0.31988827792317,
-0.309570168667151,-0.283899379158957,-0.217011923344775,-0.143922571576324,
-0.117316316451159,-0.0546021126575079,-0.0454417463122694),
 .UNSPECIFIED.);
#582=B_SPLINE_CURVE_WITH_KNOTS('',3,(#18598,#18599,#18600,#18601,#18602,
#18603),.UNSPECIFIED.,.F.,.F.,(4,2,4),(-0.0454927189511385,-0.0227385236174852,
0.),.UNSPECIFIED.);
#583=B_SPLINE_CURVE_WITH_KNOTS('',3,(#18605,#18606,#18607,#18608,#18609,
#18610,#18611,#18612,#18613,#18614,#18615,#18616,#18617,#18618,#18619,#18620,
#18621,#18622,#18623),.UNSPECIFIED.,.F.,.F.,(4,3,3,3,3,3,4),(-0.859256670515544,
-0.689904013970006,-0.517379897379589,-0.342422169251531,-0.159325101934034,
0.,0.00551932282830541),.UNSPECIFIED.);
#584=B_SPLINE_CURVE_WITH_KNOTS('',3,(#18624,#18625,#18626,#18627,#18628,
#18629,#18630,#18631,#18632,#18633,#18634,#18635,#18636,#18637,#18638,#18639,
#18640,#18641,#18642,#18643,#18644,#18645,#18646,#18647,#18648,#18649,#18650,
#18651),.UNSPECIFIED.,.F.,.F.,(4,3,3,3,3,3,3,3,3,4),(0.494993241232899,
0.496085380942586,0.497177520652273,0.49806747763899,0.499361800071647,
0.503730358910395,0.512467476587892,0.612356912997924,0.702921203547389,
0.782344701900257),.UNSPECIFIED.);
#585=B_SPLINE_CURVE_WITH_KNOTS('',3,(#18676,#18677,#18678,#18679),
 .UNSPECIFIED.,.F.,.F.,(4,4),(-0.3237356772338,0.),.UNSPECIFIED.);
#586=B_SPLINE_CURVE_WITH_KNOTS('',3,(#18682,#18683,#18684,#18685,#18686,
#18687,#18688,#18689,#18690,#18691),.UNSPECIFIED.,.F.,.F.,(4,3,3,4),(0.,
0.140915294581484,0.27533410968208,0.3237356772338),.UNSPECIFIED.);
#587=B_SPLINE_CURVE_WITH_KNOTS('',3,(#18712,#18713,#18714,#18715),
 .UNSPECIFIED.,.F.,.F.,(4,4),(-0.105411802493843,-2.2267163093265E-6),
 .UNSPECIFIED.);
#588=B_SPLINE_CURVE_WITH_KNOTS('',3,(#18718,#18719,#18720,#18721),
 .UNSPECIFIED.,.F.,.F.,(4,4),(0.,0.105411804182902),.UNSPECIFIED.);
#589=B_SPLINE_CURVE_WITH_KNOTS('',3,(#18790,#18791,#18792,#18793,#18794,
#18795,#18796,#18797,#18798,#18799),.UNSPECIFIED.,.F.,.F.,(4,2,2,2,4),(-0.092999678223845,
-0.054767181661459,-0.027983845416742,-8.71951452430242E-8,0.000452064458421415),
 .UNSPECIFIED.);
#590=B_SPLINE_CURVE_WITH_KNOTS('',3,(#18800,#18801,#18802,#18803,#18804,
#18805,#18806),.UNSPECIFIED.,.F.,.F.,(4,1,1,1,4),(9.50220145082506E-8,0.0336059064221182,
0.0672118128442549,0.11201968807377,0.156827563303286),.UNSPECIFIED.);
#591=B_SPLINE_CURVE_WITH_KNOTS('',3,(#18835,#18836,#18837,#18838,#18839),
 .UNSPECIFIED.,.F.,.F.,(4,1,4),(-0.172872079671176,-0.0864360398355901,
-4.07518504807266E-15),.UNSPECIFIED.);
#592=B_SPLINE_CURVE_WITH_KNOTS('',3,(#18840,#18841,#18842,#18843,#18844),
 .UNSPECIFIED.,.F.,.F.,(4,1,4),(4.10788875408049E-5,0.0864360398355901,
0.172872079671176),.UNSPECIFIED.);
#593=B_SPLINE_CURVE_WITH_KNOTS('',3,(#18867,#18868,#18869,#18870,#18871,
#18872,#18873,#18874,#18875,#18876),.UNSPECIFIED.,.F.,.F.,(4,3,3,4),(-0.082403918867489,
-0.0430009988442003,-0.0288947220991941,-3.17406135744279E-5),
 .UNSPECIFIED.);
#594=B_SPLINE_CURVE_WITH_KNOTS('',3,(#18877,#18878,#18879,#18880),
 .UNSPECIFIED.,.F.,.F.,(4,4),(0.00704588444375797,0.110567549348147),
 .UNSPECIFIED.);
#595=B_SPLINE_CURVE_WITH_KNOTS('',3,(#18882,#18883,#18884,#18885),
 .UNSPECIFIED.,.F.,.F.,(4,4),(-0.110567549348147,-0.0322193451720294),
 .UNSPECIFIED.);
#596=B_SPLINE_CURVE_WITH_KNOTS('',3,(#18886,#18887,#18888,#18889,#18890,
#18891),.UNSPECIFIED.,.F.,.F.,(4,2,4),(3.38858789424881E-5,0.0291642218697387,
0.058248786360198),.UNSPECIFIED.);
#597=B_SPLINE_CURVE_WITH_KNOTS('',3,(#19430,#19431,#19432,#19433),
 .UNSPECIFIED.,.F.,.F.,(4,4),(0.365433236291192,0.388387607255886),
 .UNSPECIFIED.);
#598=B_SPLINE_CURVE_WITH_KNOTS('',3,(#19955,#19956,#19957,#19958,#19959,
#19960,#19961,#19962,#19963,#19964,#19965,#19966,#19967,#19968,#19969,#19970,
#19971,#19972,#19973,#19974,#19975,#19976,#19977,#19978,#19979,#19980,#19981,
#19982,#19983,#19984,#19985,#19986,#19987,#19988),.UNSPECIFIED.,.F.,.F.,
(4,1,1,1,1,1,1,1,1,1,1,1,1,1,1,1,1,1,1,1,1,1,1,1,1,1,1,1,1,1,1,4),(0.,0.438300757907035,
0.876601515814069,1.3149022737211,1.75320303162814,2.19150378953517,2.62980454744221,
3.50640606325628,4.01775694748115,4.09080707379899,4.6752080843417,4.96740858961306,
5.11350884224874,5.25960909488442,5.55180960015577,5.84401010542713,6.42841111596984,
7.01281212651256,7.30501263178391,7.59721313705527,8.18161414759798,8.76601515814069,
9.05821566341205,9.35041616868341,9.64261667395476,9.93481717922612,10.5192181897688,
10.6287933792456,10.9575189476759,11.3958197055829,11.8341204634899,12.272421221397),
 .UNSPECIFIED.);
#599=B_SPLINE_CURVE_WITH_KNOTS('',3,(#19989,#19990,#19991,#19992,#19993),
 .UNSPECIFIED.,.F.,.F.,(4,1,4),(-0.792076380669774,-0.473360640006854,-0.0476472117508909),
 .UNSPECIFIED.);
#600=B_SPLINE_CURVE_WITH_KNOTS('',3,(#20166,#20167,#20168,#20169,#20170,
#20171),.UNSPECIFIED.,.F.,.F.,(4,2,4),(-0.0417560322026806,-0.0208857221654478,
0.),.UNSPECIFIED.);
#601=B_SPLINE_CURVE_WITH_KNOTS('',3,(#20202,#20203,#20204,#20205),
 .UNSPECIFIED.,.F.,.F.,(4,4),(-0.164738445253465,0.),.UNSPECIFIED.);
#602=B_SPLINE_CURVE_WITH_KNOTS('',3,(#20208,#20209,#20210,#20211),
 .UNSPECIFIED.,.F.,.F.,(4,4),(0.,0.164738445253465),.UNSPECIFIED.);
#603=B_SPLINE_CURVE_WITH_KNOTS('',3,(#20233,#20234,#20235,#20236),
 .UNSPECIFIED.,.F.,.F.,(4,4),(-0.0754181362626584,0.),.UNSPECIFIED.);
#604=B_SPLINE_CURVE_WITH_KNOTS('',3,(#20239,#20240,#20241,#20242),
 .UNSPECIFIED.,.F.,.F.,(4,4),(0.,0.0754181362626584),.UNSPECIFIED.);
#605=B_SPLINE_CURVE_WITH_KNOTS('',3,(#20266,#20267,#20268,#20269),
 .UNSPECIFIED.,.F.,.F.,(4,4),(-0.0505696713863416,0.),.UNSPECIFIED.);
#606=B_SPLINE_CURVE_WITH_KNOTS('',3,(#20270,#20271,#20272,#20273),
 .UNSPECIFIED.,.F.,.F.,(4,4),(0.,0.0505696713863416),.UNSPECIFIED.);
#607=B_SPLINE_CURVE_WITH_KNOTS('',3,(#20299,#20300,#20301,#20302,#20303),
 .UNSPECIFIED.,.F.,.F.,(4,1,4),(-0.167546057491724,-0.0837730396707311,
0.),.UNSPECIFIED.);
#608=B_SPLINE_CURVE_WITH_KNOTS('',3,(#20304,#20305,#20306,#20307,#20308),
 .UNSPECIFIED.,.F.,.F.,(4,1,4),(0.,0.0837730396707311,0.167546079341462),
 .UNSPECIFIED.);
#609=B_SPLINE_CURVE_WITH_KNOTS('',3,(#20336,#20337,#20338,#20339,#20340,
#20341,#20342,#20343,#20344,#20345,#20346,#20347,#20348,#20349,#20350,#20351,
#20352,#20353,#20354,#20355,#20356,#20357,#20358,#20359,#20360,#20361,#20362,
#20363,#20364,#20365,#20366,#20367,#20368,#20369,#20370,#20371,#20372,#20373,
#20374,#20375),.UNSPECIFIED.,.F.,.F.,(4,2,2,2,2,2,2,2,2,2,2,2,2,2,2,2,2,
2,2,4),(-0.143338394766602,-0.143331321978003,-0.143321921751135,-0.143310773562853,
-0.143294817451188,-0.143273441019733,-0.143239462197249,-0.143157800746622,
-0.142979467545553,-0.14264046123677,-0.141964852019619,-0.140613536202353,
-0.137910059169606,-0.132499723273395,-0.121667756807207,-0.0999966720102727,
-0.0636768389896232,-0.0323614893999653,-0.0161529766319166,0.),
 .UNSPECIFIED.);
#610=B_SPLINE_CURVE_WITH_KNOTS('',3,(#20376,#20377,#20378,#20379,#20380),
 .UNSPECIFIED.,.F.,.F.,(4,1,4),(-0.0971295855432269,-0.0737466502954258,
-0.0503637150476246),.UNSPECIFIED.);
#611=B_SPLINE_CURVE_WITH_KNOTS('',3,(#20433,#20434,#20435,#20436),
 .UNSPECIFIED.,.F.,.F.,(4,4),(0.0253342885542915,0.430969252801444),
 .UNSPECIFIED.);
#612=B_SPLINE_CURVE_WITH_KNOTS('',5,(#20438,#20439,#20440,#20441,#20442,
#20443,#20444),.UNSPECIFIED.,.F.,.F.,(6,1,6),(-0.420429130898424,-0.42,
-0.419832797309863),.UNSPECIFIED.);
#613=B_SPLINE_CURVE_WITH_KNOTS('',3,(#20564,#20565,#20566,#20567,#20568,
#20569,#20570,#20571,#20572,#20573,#20574,#20575,#20576,#20577,#20578,#20579,
#20580,#20581,#20582,#20583),.UNSPECIFIED.,.F.,.F.,(4,1,1,1,1,1,1,1,1,1,
1,1,1,1,1,1,1,4),(-2.73841348611599,-2.36517143630499,-1.97097619692083,
-1.77387857722874,-1.6753297673827,-1.62605536245968,-1.57678095753666,
-1.47823214769062,-1.37968333784458,-1.1825857181525,-1.08403690830645,
-0.985488098460413,-0.886939288614372,-0.78839047876833,-0.689841668922289,
-0.394195239384165,-0.197097619692083,0.),.UNSPECIFIED.);
#614=B_SPLINE_CURVE_WITH_KNOTS('',3,(#20586,#20587,#20588,#20589,#20590,
#20591,#20592,#20593,#20594,#20595,#20596,#20597,#20598,#20599,#20600,#20601,
#20602,#20603,#20604,#20605,#20606,#20607,#20608,#20609,#20610,#20611,#20612,
#20613,#20614,#20615,#20616,#20617,#20618,#20619,#20620,#20621,#20622,#20623,
#20624,#20625,#20626,#20627,#20628,#20629,#20630,#20631,#20632,#20633,#20634,
#20635,#20636,#20637,#20638,#20639,#20640,#20641,#20642,#20643,#20644,#20645,
#20646,#20647,#20648,#20649,#20650,#20651,#20652,#20653,#20654,#20655,#20656,
#20657,#20658,#20659,#20660,#20661,#20662,#20663,#20664,#20665,#20666,#20667,
#20668,#20669,#20670,#20671,#20672,#20673,#20674,#20675,#20676,#20677,#20678,
#20679,#20680,#20681,#20682,#20683,#20684,#20685,#20686,#20687,#20688,#20689,
#20690,#20691,#20692,#20693,#20694,#20695,#20696,#20697,#20698,#20699,#20700,
#20701,#20702,#20703,#20704,#20705,#20706,#20707,#20708,#20709,#20710,#20711,
#20712,#20713,#20714,#20715,#20716,#20717,#20718,#20719,#20720,#20721,#20722,
#20723,#20724,#20725,#20726,#20727,#20728,#20729,#20730,#20731,#20732,#20733,
#20734,#20735,#20736,#20737,#20738,#20739,#20740,#20741,#20742,#20743,#20744,
#20745,#20746,#20747,#20748,#20749,#20750,#20751,#20752,#20753,#20754,#20755,
#20756,#20757),.UNSPECIFIED.,.F.,.F.,(4,3,3,3,3,3,3,3,3,3,3,3,3,3,3,3,3,
3,3,3,3,3,3,3,3,3,3,3,3,3,3,3,3,3,3,3,3,3,3,3,3,3,3,3,3,3,3,3,3,3,3,3,3,
3,3,3,3,4),(0.,0.11697816486161,0.199552805824971,0.29207922439174,0.379904425280162,
0.414491531816278,0.487768880062305,0.558756311175645,0.627525385066692,
0.674261606492045,0.716485480031171,0.771587302682763,0.818558905154333,
0.86735829475901,0.896793608968199,0.946203496056523,0.978061410992569,
1.00230666564603,1.0367677818061,1.06943217583647,1.09199787333064,1.14810717859007,
1.17935190443171,1.20496993722993,1.24928688584476,1.29365824383217,1.3394616323277,
1.37582359152284,1.40705262279406,1.44237449278729,1.47192259312313,1.49540819182661,
1.54265747358181,1.56746644655096,1.58208267476035,1.6042054561175,1.62520599234938,
1.65028459177019,1.67022579977173,1.69055676674289,1.72445360136606,1.75960930850324,
1.78944132262637,1.82876432801193,1.86987036112636,1.913227937659,1.95926954326023,
2.00171332991122,2.06665546647158,2.13507849354725,2.20786196528303,2.28965040690062,
2.34836494049919,2.38778597604317,2.49002389242042,2.59973840902036,2.72326481917138,
2.75936667568916),.UNSPECIFIED.);
#615=B_SPLINE_CURVE_WITH_KNOTS('',3,(#20766,#20767,#20768,#20769,#20770,
#20771,#20772,#20773,#20774,#20775),.UNSPECIFIED.,.F.,.F.,(4,2,2,2,4),(-0.000388876996940957,
4.56612658924702E-11,0.0575621541740994,0.0822985038873295,0.0906504752664335),
 .UNSPECIFIED.);
#616=B_SPLINE_CURVE_WITH_KNOTS('',3,(#20777,#20778,#20779,#20780),
 .UNSPECIFIED.,.F.,.F.,(4,4),(0.,0.173814018518568),.UNSPECIFIED.);
#617=B_SPLINE_CURVE_WITH_KNOTS('',3,(#20781,#20782,#20783,#20784),
 .UNSPECIFIED.,.F.,.F.,(4,4),(-0.0459140586584383,0.),.UNSPECIFIED.);
#618=B_SPLINE_CURVE_WITH_KNOTS('',3,(#20806,#20807,#20808,#20809),
 .UNSPECIFIED.,.F.,.F.,(4,4),(-0.107690415926182,0.),.UNSPECIFIED.);
#619=B_SPLINE_CURVE_WITH_KNOTS('',3,(#20812,#20813,#20814,#20815),
 .UNSPECIFIED.,.F.,.F.,(4,4),(0.,0.304037814733278),.UNSPECIFIED.);
#620=B_SPLINE_CURVE_WITH_KNOTS('',3,(#20924,#20925,#20926,#20927,#20928,
#20929,#20930,#20931,#20932,#20933,#20934,#20935,#20936,#20937,#20938,#20939,
#20940,#20941,#20942,#20943,#20944),.UNSPECIFIED.,.F.,.F.,(4,1,1,1,1,1,
1,1,1,1,1,1,1,1,1,1,1,1,4),(-8.30491541813876,-8.15661335710056,-8.00831129606237,
-7.86000923502418,-7.71170717398599,-7.4151030519096,-7.11849892983322,
-6.52529068568045,-5.93208244152768,-4.74566595322215,-2.37283297661107,
-1.7796247324583,-1.18641648830554,-0.889812366229152,-0.593208244152768,
-0.444906183114576,-0.296604122076384,-0.148302061038192,0.),
 .UNSPECIFIED.);
#621=B_SPLINE_CURVE_WITH_KNOTS('',3,(#20966,#20967,#20968,#20969),
 .UNSPECIFIED.,.F.,.F.,(4,4),(-0.0801298062965183,0.),.UNSPECIFIED.);
#622=B_SPLINE_CURVE_WITH_KNOTS('',3,(#20970,#20971,#20972,#20973),
 .UNSPECIFIED.,.F.,.F.,(4,4),(0.,0.0801298062965183),.UNSPECIFIED.);
#623=B_SPLINE_CURVE_WITH_KNOTS('',3,(#21015,#21016,#21017,#21018),
 .UNSPECIFIED.,.F.,.F.,(4,4),(-0.080129806296636,-2.65444323739948E-13),
 .UNSPECIFIED.);
#624=B_SPLINE_CURVE_WITH_KNOTS('',3,(#21022,#21023,#21024,#21025,#21026,
#21027),.UNSPECIFIED.,.F.,.F.,(4,1,1,4),(-0.344667552668405,-0.264773640517305,
-0.184879728366205,-0.0650388601395548),.UNSPECIFIED.);
#625=B_SPLINE_CURVE_WITH_KNOTS('',3,(#21036,#21037,#21038,#21039),
 .UNSPECIFIED.,.F.,.F.,(4,4),(-0.357185215222936,0.),.UNSPECIFIED.);
#626=B_SPLINE_CURVE_WITH_KNOTS('',3,(#21044,#21045,#21046,#21047,#21048),
 .UNSPECIFIED.,.F.,.F.,(4,1,4),(0.0124441963939058,0.048258887840249,0.0965121156546766),
 .UNSPECIFIED.);
#627=B_SPLINE_CURVE_WITH_KNOTS('',3,(#21087,#21088,#21089,#21090,#21091,
#21092,#21093,#21094),.UNSPECIFIED.,.F.,.F.,(4,2,2,4),(0.000388650349350716,
0.116108579564429,0.168099156279993,0.196635243830291),.UNSPECIFIED.);
#628=B_SPLINE_CURVE_WITH_KNOTS('',3,(#21098,#21099,#21100,#21101,#21102,
#21103,#21104,#21105,#21106,#21107,#21108,#21109,#21110,#21111),
 .UNSPECIFIED.,.F.,.F.,(4,2,2,2,2,2,4),(0.000179524113000012,0.0103957521563598,
0.0961675209313773,0.135083973905907,0.163219630081561,0.178069326504183,
0.19211441705983),.UNSPECIFIED.);
#629=B_SPLINE_CURVE_WITH_KNOTS('',3,(#21115,#21116,#21117,#21118),
 .UNSPECIFIED.,.F.,.F.,(4,4),(-0.921184518536775,-0.83453843347903),
 .UNSPECIFIED.);
#630=B_SPLINE_CURVE_WITH_KNOTS('',3,(#21120,#21121,#21122,#21123,#21124,
#21125),.UNSPECIFIED.,.F.,.F.,(4,2,4),(-0.150027473993582,-0.0719000872483259,
-1.60162876488653E-5),.UNSPECIFIED.);
#631=B_SPLINE_CURVE_WITH_KNOTS('',3,(#21127,#21128,#21129,#21130,#21131,
#21132,#21133,#21134),.UNSPECIFIED.,.F.,.F.,(4,2,2,4),(-0.159862307608192,
-0.0802383050665597,0.,0.000515045900834663),.UNSPECIFIED.);
#632=B_SPLINE_CURVE_WITH_KNOTS('',3,(#21138,#21139,#21140,#21141,#21142,
#21143,#21144,#21145),.UNSPECIFIED.,.F.,.F.,(4,2,2,4),(0.000127650722345724,
0.0504964849387841,0.100554030953333,0.101083886401504),.UNSPECIFIED.);
#633=B_SPLINE_CURVE_WITH_KNOTS('',3,(#21147,#21148,#21149,#21150,#21151,
#21152,#21153,#21154,#21155,#21156,#21157,#21158,#21159,#21160),
 .UNSPECIFIED.,.F.,.F.,(4,2,2,2,2,2,4),(0.,0.0370101874890961,0.0864161496254977,
0.117374893296465,0.141975914212591,0.160694465086184,0.18074188497048),
 .UNSPECIFIED.);
#634=B_SPLINE_CURVE_WITH_KNOTS('',3,(#21164,#21165,#21166,#21167,#21168),
 .UNSPECIFIED.,.F.,.F.,(4,1,4),(0.,0.0482654156519333,0.0840891532006709),
 .UNSPECIFIED.);
#635=B_SPLINE_CURVE_WITH_KNOTS('',3,(#21172,#21173,#21174,#21175),
 .UNSPECIFIED.,.F.,.F.,(4,4),(-0.0801298062968181,-2.63411853293822E-13),
 .UNSPECIFIED.);
#636=B_SPLINE_CURVE_WITH_KNOTS('',3,(#21180,#21181,#21182,#21183,#21184),
 .UNSPECIFIED.,.F.,.F.,(4,1,4),(-0.121804337225533,-0.0522018588109426,
0.),.UNSPECIFIED.);
#637=B_SPLINE_CURVE_WITH_KNOTS('',3,(#21185,#21186,#21187,#21188,#21189,
#21190),.UNSPECIFIED.,.F.,.F.,(4,2,4),(-0.0372063908700252,-0.0185630077537129,
0.),.UNSPECIFIED.);
#638=B_SPLINE_CURVE_WITH_KNOTS('',3,(#21244,#21245,#21246,#21247),
 .UNSPECIFIED.,.F.,.F.,(4,4),(0.,0.35717455535325),.UNSPECIFIED.);
#639=B_SPLINE_CURVE_WITH_KNOTS('',3,(#21281,#21282,#21283,#21284,#21285,
#21286),.UNSPECIFIED.,.F.,.F.,(4,1,1,4),(0.0650388601395548,0.184879728366205,
0.264773640517305,0.344667552668405),.UNSPECIFIED.);
#640=B_SPLINE_CURVE_WITH_KNOTS('',3,(#21852,#21853,#21854,#21855,#21856),
 .UNSPECIFIED.,.F.,.F.,(4,1,4),(0.122333686396133,0.336302079828547,0.52623217118239),
 .UNSPECIFIED.);
#641=B_SPLINE_CURVE_WITH_KNOTS('',3,(#21891,#21892,#21893,#21894,#21895,
#21896,#21897,#21898,#21899,#21900,#21901,#21902,#21903,#21904,#21905,#21906,
#21907,#21908,#21909,#21910,#21911,#21912,#21913,#21914,#21915),
 .UNSPECIFIED.,.F.,.F.,(4,3,3,3,3,3,3,3,4),(0.0476472117481897,0.176707628536091,
0.309197145860186,0.421180594715224,0.473360639981091,0.629106032564461,
0.80736131459052,0.81926637292792,1.03517553998266),.UNSPECIFIED.);
#642=B_SPLINE_CURVE_WITH_KNOTS('',3,(#21916,#21917,#21918,#21919),
 .UNSPECIFIED.,.F.,.F.,(4,4),(1.03517572369524,1.04062713634001),
 .UNSPECIFIED.);
#643=B_SPLINE_CURVE_WITH_KNOTS('',3,(#21979,#21980,#21981,#21982),
 .UNSPECIFIED.,.F.,.F.,(4,4),(-0.254963272600067,-0.19533758964745),
 .UNSPECIFIED.);
#644=B_SPLINE_CURVE_WITH_KNOTS('',3,(#22003,#22004,#22005,#22006),
 .UNSPECIFIED.,.F.,.F.,(4,4),(2.63411853293822E-13,0.0801298062968181),
 .UNSPECIFIED.);
#645=B_SPLINE_CURVE_WITH_KNOTS('',3,(#22021,#22022,#22023,#22024,#22025,
#22026),.UNSPECIFIED.,.F.,.F.,(4,2,4),(-0.0739729607057787,0.,0.00065196825529525),
 .UNSPECIFIED.);
#646=B_SPLINE_CURVE_WITH_KNOTS('',3,(#22030,#22031,#22032,#22033,#22034,
#22035,#22036,#22037,#22038,#22039,#22040,#22041,#22042),.UNSPECIFIED.,
 .F.,.F.,(4,3,3,3,4),(-0.0741141580594659,-0.0733119809727613,-0.0421649270605065,
-0.0161079664769414,-3.24706403037789E-5),.UNSPECIFIED.);
#647=B_SPLINE_CURVE_WITH_KNOTS('',1,(#22043,#22044),.UNSPECIFIED.,.F.,.F.,
(2,2),(-0.0103667322106565,0.),.UNSPECIFIED.);
#648=B_SPLINE_CURVE_WITH_KNOTS('',3,(#22046,#22047,#22048,#22049,#22050,
#22051),.UNSPECIFIED.,.F.,.F.,(4,2,4),(-0.000271009268404639,-0.000152937970284206,
-1.02670240187253E-5),.UNSPECIFIED.);
#649=B_SPLINE_CURVE_WITH_KNOTS('',3,(#22084,#22085,#22086,#22087,#22088,
#22089,#22090,#22091,#22092,#22093,#22094,#22095,#22096,#22097,#22098,#22099),
 .UNSPECIFIED.,.F.,.F.,(4,3,3,3,3,4),(-0.170468208410896,-0.121851917489685,
-0.109877931374803,-0.0874114081347553,-0.0402533150305619,0.),
 .UNSPECIFIED.);
#650=B_SPLINE_CURVE_WITH_KNOTS('',3,(#22148,#22149,#22150,#22151,#22152,
#22153),.UNSPECIFIED.,.F.,.F.,(4,1,1,4),(-0.251165001188368,-0.179403572277406,
-0.107642143366443,0.),.UNSPECIFIED.);
#651=B_SPLINE_CURVE_WITH_KNOTS('',3,(#22175,#22176,#22177,#22178),
 .UNSPECIFIED.,.F.,.F.,(4,4),(0.00243784671109485,0.137031673359032),
 .UNSPECIFIED.);
#652=B_SPLINE_CURVE_WITH_KNOTS('',3,(#22308,#22309,#22310,#22311),
 .UNSPECIFIED.,.F.,.F.,(4,4),(0.,0.0029947073568665),.UNSPECIFIED.);
#653=B_SPLINE_CURVE_WITH_KNOTS('',3,(#22313,#22314,#22315,#22316,#22317,
#22318,#22319,#22320,#22321,#22322,#22323,#22324,#22325,#22326,#22327,#22328,
#22329,#22330,#22331,#22332,#22333,#22334,#22335,#22336,#22337,#22338,#22339,
#22340,#22341,#22342,#22343,#22344,#22345,#22346,#22347,#22348,#22349,#22350,
#22351,#22352,#22353,#22354,#22355,#22356,#22357,#22358,#22359,#22360,#22361,
#22362,#22363,#22364,#22365,#22366,#22367,#22368,#22369,#22370,#22371,#22372,
#22373,#22374,#22375,#22376,#22377,#22378,#22379,#22380,#22381,#22382,#22383,
#22384,#22385,#22386,#22387,#22388,#22389,#22390,#22391,#22392,#22393,#22394,
#22395,#22396,#22397,#22398,#22399,#22400,#22401,#22402,#22403,#22404,#22405,
#22406,#22407,#22408,#22409,#22410,#22411,#22412,#22413,#22414,#22415,#22416,
#22417,#22418,#22419,#22420,#22421,#22422,#22423,#22424,#22425,#22426,#22427,
#22428,#22429,#22430,#22431,#22432,#22433,#22434,#22435,#22436,#22437,#22438,
#22439,#22440,#22441,#22442,#22443,#22444,#22445,#22446,#22447,#22448,#22449,
#22450,#22451,#22452,#22453,#22454,#22455,#22456,#22457,#22458,#22459,#22460,
#22461,#22462,#22463,#22464,#22465,#22466,#22467,#22468,#22469,#22470,#22471,
#22472,#22473,#22474,#22475,#22476,#22477,#22478),.UNSPECIFIED.,.F.,.F.,
(4,3,3,3,3,3,3,3,3,3,3,3,3,3,3,3,3,3,3,3,3,3,3,3,3,3,3,3,3,3,3,3,3,3,3,
3,3,3,3,3,3,3,3,3,3,3,3,3,3,3,3,3,3,3,3,4),(0.150051581338353,0.256863936659208,
0.335221624046453,0.385884192471485,0.415095529930595,0.496109926387356,
0.569942607877855,0.638650952641705,0.705077795779496,0.769428800069232,
0.804505228482622,0.849643463003826,0.892080534823519,0.932340746449873,
0.971002669683063,0.990292699500749,1.02414419558244,1.05133428523039,1.07725069503007,
1.10382298151386,1.12328365106401,1.14494121098181,1.1667241512046,1.18428652869351,
1.20604733438692,1.24354147974281,1.28115827676027,1.31547262018988,1.33594212716517,
1.37354010313882,1.4132592349251,1.44718380388559,1.48803315339709,1.53384225960426,
1.57229437439947,1.60642722308793,1.66117380917141,1.68727241905653,1.72119555000744,
1.75379287447755,1.77871300744534,1.8485007475128,1.91500567133357,1.96808718769091,
2.00382424755494,2.05135460289845,2.08266994362526,2.15070750358199,2.21528666185066,
2.28827074173757,2.35567498677221,2.40419094803851,2.50311616375164,2.60679823955146,
2.71856348129842,2.76430993305103),.UNSPECIFIED.);
#654=B_SPLINE_CURVE_WITH_KNOTS('',3,(#22482,#22483,#22484,#22485,#22486,
#22487,#22488,#22489,#22490,#22491,#22492,#22493,#22494,#22495,#22496,#22497,
#22498,#22499,#22500,#22501),.UNSPECIFIED.,.F.,.F.,(4,1,1,1,1,1,1,1,1,1,
1,1,1,1,1,1,1,4),(-2.76430993305103,-2.37006408126403,-2.17294115537053,
-2.07437969242378,-1.97581822947703,-1.77869530358353,-1.68013384063678,
-1.58157237769003,-1.45015709376104,-1.31874180983204,-1.18732652590304,
-1.12161888393854,-1.05591124197404,-1.02305742099179,-0.990203600009539,
-0.79308067411604,-0.398834822329043,-0.00458897054204579),
 .UNSPECIFIED.);
#655=B_SPLINE_CURVE_WITH_KNOTS('',3,(#22519,#22520,#22521,#22522),
 .UNSPECIFIED.,.F.,.F.,(4,4),(0.7519797577463,0.919615460485724),
 .UNSPECIFIED.);
#656=B_SPLINE_CURVE_WITH_KNOTS('',3,(#22565,#22566,#22567,#22568),
 .UNSPECIFIED.,.F.,.F.,(4,4),(-0.419743206478425,-0.0797065098565302),
 .UNSPECIFIED.);
#657=B_SPLINE_CURVE_WITH_KNOTS('',3,(#22571,#22572,#22573,#22574),
 .UNSPECIFIED.,.F.,.F.,(4,4),(0.0797065098565302,0.419743206478425),
 .UNSPECIFIED.);
#658=B_SPLINE_CURVE_WITH_KNOTS('',3,(#22672,#22673,#22674,#22675),
 .UNSPECIFIED.,.F.,.F.,(4,4),(-0.166269642083837,0.),.UNSPECIFIED.);
#659=B_SPLINE_CURVE_WITH_KNOTS('',3,(#22699,#22700,#22701,#22702),
 .UNSPECIFIED.,.F.,.F.,(4,4),(0.,0.0459140586584383),.UNSPECIFIED.);
#660=B_SPLINE_CURVE_WITH_KNOTS('',3,(#22742,#22743,#22744,#22745),
 .UNSPECIFIED.,.F.,.F.,(4,4),(0.121211854500864,0.461940930144229),
 .UNSPECIFIED.);
#995=PLANE('',#10108);
#996=PLANE('',#10113);
#997=PLANE('',#10122);
#998=PLANE('',#10126);
#999=PLANE('',#10180);
#1000=PLANE('',#10206);
#1001=PLANE('',#10217);
#1002=PLANE('',#10225);
#1003=PLANE('',#10245);
#1004=PLANE('',#10247);
#1005=PLANE('',#10264);
#1006=PLANE('',#10270);
#1007=PLANE('',#10272);
#1008=PLANE('',#10273);
#1009=PLANE('',#10294);
#1010=PLANE('',#10300);
#1011=PLANE('',#10301);
#1012=PLANE('',#10302);
#1199=LINE('',#13229,#1735);
#1200=LINE('',#13236,#1736);
#1201=LINE('',#13243,#1737);
#1202=LINE('',#13245,#1738);
#1203=LINE('',#13306,#1739);
#1204=LINE('',#13414,#1740);
#1205=LINE('',#13421,#1741);
#1206=LINE('',#13431,#1742);
#1207=LINE('',#13626,#1743);
#1208=LINE('',#13662,#1744);
#1209=LINE('',#13665,#1745);
#1210=LINE('',#13697,#1746);
#1211=LINE('',#14824,#1747);
#1212=LINE('',#15430,#1748);
#1213=LINE('',#15655,#1749);
#1214=LINE('',#15961,#1750);
#1215=LINE('',#16625,#1751);
#1216=LINE('',#17097,#1752);
#1217=LINE('',#17753,#1753);
#1218=LINE('',#17756,#1754);
#1219=LINE('',#17768,#1755);
#1220=LINE('',#17783,#1756);
#1221=LINE('',#17784,#1757);
#1222=LINE('',#18904,#1758);
#1223=LINE('',#20174,#1759);
#1224=LINE('',#20177,#1760);
#1225=LINE('',#20445,#1761);
#1226=LINE('',#20760,#1762);
#1227=LINE('',#20764,#1763);
#1228=LINE('',#21021,#1764);
#1229=LINE('',#21030,#1765);
#1230=LINE('',#21032,#1766);
#1231=LINE('',#21042,#1767);
#1232=LINE('',#21049,#1768);
#1233=LINE('',#21060,#1769);
#1234=LINE('',#21066,#1770);
#1235=LINE('',#21069,#1771);
#1236=LINE('',#21072,#1772);
#1237=LINE('',#21074,#1773);
#1238=LINE('',#21081,#1774);
#1239=LINE('',#21085,#1775);
#1240=LINE('',#21095,#1776);
#1241=LINE('',#21097,#1777);
#1242=LINE('',#21136,#1778);
#1243=LINE('',#21162,#1779);
#1244=LINE('',#21169,#1780);
#1245=LINE('',#21170,#1781);
#1246=LINE('',#21176,#1782);
#1247=LINE('',#21177,#1783);
#1248=LINE('',#21179,#1784);
#1249=LINE('',#21851,#1785);
#1250=LINE('',#22028,#1786);
#1251=LINE('',#22045,#1787);
#1252=LINE('',#22082,#1788);
#1253=LINE('',#22116,#1789);
#1254=LINE('',#22623,#1790);
#1255=LINE('',#22650,#1791);
#1256=LINE('',#22795,#1792);
#1257=LINE('',#22798,#1793);
#1258=LINE('',#23320,#1794);
#1259=LINE('',#23322,#1795);
#1260=LINE('',#23324,#1796);
#1261=LINE('',#23326,#1797);
#1735=VECTOR('',#10975,1.35);
#1736=VECTOR('',#10982,1.);
#1737=VECTOR('',#10983,1.);
#1738=VECTOR('',#10984,1.);
#1739=VECTOR('',#10995,1.);
#1740=VECTOR('',#11008,1.35);
#1741=VECTOR('',#11015,1.);
#1742=VECTOR('',#11016,1.);
#1743=VECTOR('',#11025,1.);
#1744=VECTOR('',#11026,1.);
#1745=VECTOR('',#11029,1.);
#1746=VECTOR('',#11034,1.);
#1747=VECTOR('',#11075,1.);
#1748=VECTOR('',#11088,1.);
#1749=VECTOR('',#11089,1.);
#1750=VECTOR('',#11110,1.);
#1751=VECTOR('',#11113,1.);
#1752=VECTOR('',#11142,1.);
#1753=VECTOR('',#11145,1.);
#1754=VECTOR('',#11150,1.);
#1755=VECTOR('',#11151,1.);
#1756=VECTOR('',#11156,1.);
#1757=VECTOR('',#11157,1.);
#1758=VECTOR('',#11186,1.);
#1759=VECTOR('',#11203,1.);
#1760=VECTOR('',#11206,1.);
#1761=VECTOR('',#11219,1.);
#1762=VECTOR('',#11226,1.);
#1763=VECTOR('',#11231,1.);
#1764=VECTOR('',#11242,1.);
#1765=VECTOR('',#11245,1.);
#1766=VECTOR('',#11246,1.);
#1767=VECTOR('',#11251,1.);
#1768=VECTOR('',#11252,1.);
#1769=VECTOR('',#11263,1.);
#1770=VECTOR('',#11270,1.);
#1771=VECTOR('',#11273,1.);
#1772=VECTOR('',#11276,1.);
#1773=VECTOR('',#11279,1.);
#1774=VECTOR('',#11290,1.);
#1775=VECTOR('',#11295,1.);
#1776=VECTOR('',#11296,1.);
#1777=VECTOR('',#11299,1.);
#1778=VECTOR('',#11302,1.);
#1779=VECTOR('',#11303,1.);
#1780=VECTOR('',#11304,1.);
#1781=VECTOR('',#11305,1.);
#1782=VECTOR('',#11306,1.);
#1783=VECTOR('',#11307,1.);
#1784=VECTOR('',#11308,1.);
#1785=VECTOR('',#11337,1.);
#1786=VECTOR('',#11352,1.);
#1787=VECTOR('',#11353,1.);
#1788=VECTOR('',#11354,1.);
#1789=VECTOR('',#11365,1.);
#1790=VECTOR('',#11394,1.);
#1791=VECTOR('',#11395,1.);
#1792=VECTOR('',#11408,1.);
#1793=VECTOR('',#11413,1.);
#1794=VECTOR('',#11416,0.3);
#1795=VECTOR('',#11419,0.36);
#1796=VECTOR('',#11422,0.36);
#1797=VECTOR('',#11425,0.3);
#2271=CYLINDRICAL_SURFACE('',#10105,1.35);
#2272=CYLINDRICAL_SURFACE('',#10119,1.35);
#2273=CYLINDRICAL_SURFACE('',#10128,0.08);
#2274=CYLINDRICAL_SURFACE('',#10148,0.9);
#2275=CYLINDRICAL_SURFACE('',#10183,0.9);
#2276=CYLINDRICAL_SURFACE('',#10184,0.0800457110804505);
#2277=CYLINDRICAL_SURFACE('',#10203,0.08);
#2278=CYLINDRICAL_SURFACE('',#10207,0.08);
#2279=CYLINDRICAL_SURFACE('',#10219,0.9);
#2280=CYLINDRICAL_SURFACE('',#10224,0.9);
#2281=CYLINDRICAL_SURFACE('',#10232,0.08);
#2282=CYLINDRICAL_SURFACE('',#10234,0.08);
#2283=CYLINDRICAL_SURFACE('',#10237,0.08);
#2284=CYLINDRICAL_SURFACE('',#10243,0.08);
#2285=CYLINDRICAL_SURFACE('',#10246,0.08);
#2286=CYLINDRICAL_SURFACE('',#10262,0.0800457110810776);
#2287=CYLINDRICAL_SURFACE('',#10267,0.4);
#2288=CYLINDRICAL_SURFACE('',#10268,0.4);
#2289=CYLINDRICAL_SURFACE('',#10293,0.4);
#2290=CYLINDRICAL_SURFACE('',#10295,0.4);
#2291=CYLINDRICAL_SURFACE('',#10296,0.3);
#2292=CYLINDRICAL_SURFACE('',#10297,0.36);
#2293=CYLINDRICAL_SURFACE('',#10298,0.36);
#2294=CYLINDRICAL_SURFACE('',#10299,0.3);
#2402=FACE_OUTER_BOUND('',#2903,.T.);
#2403=FACE_OUTER_BOUND('',#2904,.T.);
#2404=FACE_OUTER_BOUND('',#2905,.T.);
#2405=FACE_OUTER_BOUND('',#2907,.T.);
#2406=FACE_OUTER_BOUND('',#2908,.T.);
#2407=FACE_OUTER_BOUND('',#2910,.T.);
#2408=FACE_OUTER_BOUND('',#2911,.T.);
#2409=FACE_OUTER_BOUND('',#2912,.T.);
#2410=FACE_OUTER_BOUND('',#2914,.T.);
#2411=FACE_OUTER_BOUND('',#2915,.T.);
#2412=FACE_OUTER_BOUND('',#2917,.T.);
#2413=FACE_OUTER_BOUND('',#2918,.T.);
#2414=FACE_OUTER_BOUND('',#2919,.T.);
#2415=FACE_OUTER_BOUND('',#2920,.T.);
#2416=FACE_OUTER_BOUND('',#2921,.T.);
#2417=FACE_OUTER_BOUND('',#2922,.T.);
#2418=FACE_OUTER_BOUND('',#2923,.T.);
#2419=FACE_OUTER_BOUND('',#2924,.T.);
#2420=FACE_OUTER_BOUND('',#2925,.T.);
#2421=FACE_OUTER_BOUND('',#2926,.T.);
#2422=FACE_OUTER_BOUND('',#2927,.T.);
#2423=FACE_OUTER_BOUND('',#2928,.T.);
#2424=FACE_OUTER_BOUND('',#2929,.T.);
#2425=FACE_OUTER_BOUND('',#2930,.T.);
#2426=FACE_OUTER_BOUND('',#2931,.T.);
#2427=FACE_OUTER_BOUND('',#2932,.T.);
#2428=FACE_OUTER_BOUND('',#2933,.T.);
#2429=FACE_OUTER_BOUND('',#2934,.T.);
#2430=FACE_OUTER_BOUND('',#2935,.T.);
#2431=FACE_OUTER_BOUND('',#2936,.T.);
#2432=FACE_OUTER_BOUND('',#2937,.T.);
#2433=FACE_OUTER_BOUND('',#2938,.T.);
#2434=FACE_OUTER_BOUND('',#2939,.T.);
#2435=FACE_OUTER_BOUND('',#2940,.T.);
#2436=FACE_OUTER_BOUND('',#2941,.T.);
#2437=FACE_OUTER_BOUND('',#2942,.T.);
#2438=FACE_OUTER_BOUND('',#2943,.T.);
#2439=FACE_OUTER_BOUND('',#2944,.T.);
#2440=FACE_OUTER_BOUND('',#2945,.T.);
#2441=FACE_OUTER_BOUND('',#2946,.T.);
#2442=FACE_OUTER_BOUND('',#2947,.T.);
#2443=FACE_OUTER_BOUND('',#2948,.T.);
#2444=FACE_OUTER_BOUND('',#2949,.T.);
#2445=FACE_OUTER_BOUND('',#2950,.T.);
#2446=FACE_OUTER_BOUND('',#2951,.T.);
#2447=FACE_OUTER_BOUND('',#2952,.T.);
#2448=FACE_OUTER_BOUND('',#2953,.T.);
#2449=FACE_OUTER_BOUND('',#2954,.T.);
#2450=FACE_OUTER_BOUND('',#2955,.T.);
#2451=FACE_OUTER_BOUND('',#2956,.T.);
#2452=FACE_OUTER_BOUND('',#2957,.T.);
#2453=FACE_OUTER_BOUND('',#2958,.T.);
#2454=FACE_OUTER_BOUND('',#2959,.T.);
#2455=FACE_OUTER_BOUND('',#2960,.T.);
#2456=FACE_OUTER_BOUND('',#2961,.T.);
#2457=FACE_OUTER_BOUND('',#2962,.T.);
#2458=FACE_OUTER_BOUND('',#2963,.T.);
#2459=FACE_OUTER_BOUND('',#2964,.T.);
#2460=FACE_OUTER_BOUND('',#2965,.T.);
#2461=FACE_OUTER_BOUND('',#2966,.T.);
#2462=FACE_OUTER_BOUND('',#2967,.T.);
#2463=FACE_OUTER_BOUND('',#2968,.T.);
#2464=FACE_OUTER_BOUND('',#2969,.T.);
#2465=FACE_OUTER_BOUND('',#2970,.T.);
#2466=FACE_OUTER_BOUND('',#2971,.T.);
#2467=FACE_OUTER_BOUND('',#2972,.T.);
#2468=FACE_OUTER_BOUND('',#2973,.T.);
#2469=FACE_OUTER_BOUND('',#2974,.T.);
#2470=FACE_OUTER_BOUND('',#2975,.T.);
#2471=FACE_OUTER_BOUND('',#2976,.T.);
#2472=FACE_OUTER_BOUND('',#2977,.T.);
#2473=FACE_OUTER_BOUND('',#2978,.T.);
#2474=FACE_OUTER_BOUND('',#2979,.T.);
#2475=FACE_OUTER_BOUND('',#2980,.T.);
#2476=FACE_OUTER_BOUND('',#2981,.T.);
#2477=FACE_OUTER_BOUND('',#2982,.T.);
#2478=FACE_OUTER_BOUND('',#2983,.T.);
#2479=FACE_OUTER_BOUND('',#2984,.T.);
#2480=FACE_OUTER_BOUND('',#2985,.T.);
#2481=FACE_OUTER_BOUND('',#2986,.T.);
#2482=FACE_OUTER_BOUND('',#2987,.T.);
#2483=FACE_OUTER_BOUND('',#2988,.T.);
#2484=FACE_OUTER_BOUND('',#2989,.T.);
#2485=FACE_OUTER_BOUND('',#2990,.T.);
#2486=FACE_OUTER_BOUND('',#2991,.T.);
#2487=FACE_OUTER_BOUND('',#2992,.T.);
#2488=FACE_OUTER_BOUND('',#2993,.T.);
#2489=FACE_OUTER_BOUND('',#2994,.T.);
#2490=FACE_OUTER_BOUND('',#2995,.T.);
#2491=FACE_OUTER_BOUND('',#2996,.T.);
#2492=FACE_OUTER_BOUND('',#2997,.T.);
#2493=FACE_OUTER_BOUND('',#2998,.T.);
#2494=FACE_OUTER_BOUND('',#2999,.T.);
#2495=FACE_OUTER_BOUND('',#3000,.T.);
#2496=FACE_OUTER_BOUND('',#3001,.T.);
#2497=FACE_OUTER_BOUND('',#3002,.T.);
#2498=FACE_OUTER_BOUND('',#3003,.T.);
#2499=FACE_OUTER_BOUND('',#3004,.T.);
#2500=FACE_OUTER_BOUND('',#3009,.T.);
#2501=FACE_OUTER_BOUND('',#3010,.T.);
#2502=FACE_OUTER_BOUND('',#3011,.T.);
#2503=FACE_OUTER_BOUND('',#3012,.T.);
#2504=FACE_OUTER_BOUND('',#3013,.T.);
#2505=FACE_OUTER_BOUND('',#3014,.T.);
#2506=FACE_OUTER_BOUND('',#3015,.T.);
#2507=FACE_OUTER_BOUND('',#3016,.T.);
#2508=FACE_OUTER_BOUND('',#3017,.T.);
#2509=FACE_OUTER_BOUND('',#3022,.T.);
#2510=FACE_OUTER_BOUND('',#3023,.T.);
#2511=FACE_OUTER_BOUND('',#3024,.T.);
#2512=FACE_OUTER_BOUND('',#3025,.T.);
#2513=FACE_OUTER_BOUND('',#3026,.T.);
#2514=FACE_OUTER_BOUND('',#3027,.T.);
#2515=FACE_OUTER_BOUND('',#3028,.T.);
#2516=FACE_OUTER_BOUND('',#3029,.T.);
#2517=FACE_OUTER_BOUND('',#3030,.T.);
#2518=FACE_OUTER_BOUND('',#3031,.T.);
#2519=FACE_OUTER_BOUND('',#3032,.T.);
#2520=FACE_OUTER_BOUND('',#3033,.T.);
#2521=FACE_OUTER_BOUND('',#3034,.T.);
#2522=FACE_OUTER_BOUND('',#3035,.T.);
#2523=FACE_OUTER_BOUND('',#3036,.T.);
#2524=FACE_OUTER_BOUND('',#3037,.T.);
#2525=FACE_OUTER_BOUND('',#3038,.T.);
#2526=FACE_OUTER_BOUND('',#3039,.T.);
#2527=FACE_OUTER_BOUND('',#3040,.T.);
#2528=FACE_OUTER_BOUND('',#3041,.T.);
#2529=FACE_OUTER_BOUND('',#3042,.T.);
#2530=FACE_OUTER_BOUND('',#3043,.T.);
#2531=FACE_OUTER_BOUND('',#3044,.T.);
#2532=FACE_OUTER_BOUND('',#3045,.T.);
#2533=FACE_OUTER_BOUND('',#3046,.T.);
#2534=FACE_OUTER_BOUND('',#3047,.T.);
#2535=FACE_OUTER_BOUND('',#3048,.T.);
#2536=FACE_OUTER_BOUND('',#3049,.T.);
#2537=FACE_OUTER_BOUND('',#3050,.T.);
#2538=FACE_OUTER_BOUND('',#3051,.T.);
#2539=FACE_OUTER_BOUND('',#3052,.T.);
#2540=FACE_OUTER_BOUND('',#3053,.T.);
#2541=FACE_OUTER_BOUND('',#3054,.T.);
#2542=FACE_OUTER_BOUND('',#3055,.T.);
#2543=FACE_OUTER_BOUND('',#3056,.T.);
#2544=FACE_OUTER_BOUND('',#3057,.T.);
#2545=FACE_OUTER_BOUND('',#3058,.T.);
#2546=FACE_OUTER_BOUND('',#3059,.T.);
#2547=FACE_OUTER_BOUND('',#3060,.T.);
#2548=FACE_OUTER_BOUND('',#3061,.T.);
#2549=FACE_OUTER_BOUND('',#3062,.T.);
#2550=FACE_OUTER_BOUND('',#3063,.T.);
#2551=FACE_OUTER_BOUND('',#3064,.T.);
#2552=FACE_OUTER_BOUND('',#3065,.T.);
#2553=FACE_OUTER_BOUND('',#3066,.T.);
#2554=FACE_OUTER_BOUND('',#3067,.T.);
#2555=FACE_OUTER_BOUND('',#3068,.T.);
#2556=FACE_OUTER_BOUND('',#3069,.T.);
#2557=FACE_OUTER_BOUND('',#3070,.T.);
#2903=EDGE_LOOP('',(#6415,#6416,#6417,#6418,#6419));
#2904=EDGE_LOOP('',(#6420,#6421,#6422,#6423,#6424,#6425));
#2905=EDGE_LOOP('',(#6426,#6427,#6428,#6429,#6430,#6431));
#2906=EDGE_LOOP('',(#6432));
#2907=EDGE_LOOP('',(#6433,#6434,#6435,#6436,#6437));
#2908=EDGE_LOOP('',(#6438,#6439,#6440,#6441,#6442,#6443,#6444,#6445,#6446));
#2909=EDGE_LOOP('',(#6447));
#2910=EDGE_LOOP('',(#6448,#6449,#6450,#6451,#6452));
#2911=EDGE_LOOP('',(#6453,#6454,#6455,#6456,#6457,#6458));
#2912=EDGE_LOOP('',(#6459,#6460,#6461,#6462,#6463));
#2913=EDGE_LOOP('',(#6464));
#2914=EDGE_LOOP('',(#6465,#6466,#6467,#6468,#6469));
#2915=EDGE_LOOP('',(#6470,#6471,#6472,#6473,#6474,#6475,#6476,#6477,#6478,
#6479,#6480));
#2916=EDGE_LOOP('',(#6481));
#2917=EDGE_LOOP('',(#6482,#6483,#6484,#6485,#6486));
#2918=EDGE_LOOP('',(#6487,#6488,#6489,#6490));
#2919=EDGE_LOOP('',(#6491,#6492,#6493));
#2920=EDGE_LOOP('',(#6494,#6495,#6496,#6497,#6498,#6499,#6500,#6501));
#2921=EDGE_LOOP('',(#6502,#6503,#6504,#6505));
#2922=EDGE_LOOP('',(#6506,#6507,#6508));
#2923=EDGE_LOOP('',(#6509,#6510,#6511,#6512));
#2924=EDGE_LOOP('',(#6513,#6514,#6515));
#2925=EDGE_LOOP('',(#6516,#6517,#6518,#6519));
#2926=EDGE_LOOP('',(#6520,#6521,#6522,#6523,#6524));
#2927=EDGE_LOOP('',(#6525,#6526,#6527,#6528));
#2928=EDGE_LOOP('',(#6529,#6530,#6531,#6532));
#2929=EDGE_LOOP('',(#6533,#6534,#6535,#6536));
#2930=EDGE_LOOP('',(#6537,#6538,#6539,#6540));
#2931=EDGE_LOOP('',(#6541,#6542,#6543,#6544));
#2932=EDGE_LOOP('',(#6545,#6546,#6547,#6548,#6549,#6550));
#2933=EDGE_LOOP('',(#6551,#6552,#6553,#6554));
#2934=EDGE_LOOP('',(#6555,#6556,#6557,#6558));
#2935=EDGE_LOOP('',(#6559,#6560,#6561,#6562,#6563,#6564));
#2936=EDGE_LOOP('',(#6565,#6566));
#2937=EDGE_LOOP('',(#6567,#6568,#6569));
#2938=EDGE_LOOP('',(#6570,#6571,#6572,#6573));
#2939=EDGE_LOOP('',(#6574,#6575,#6576,#6577,#6578,#6579));
#2940=EDGE_LOOP('',(#6580,#6581,#6582,#6583,#6584));
#2941=EDGE_LOOP('',(#6585,#6586,#6587,#6588,#6589));
#2942=EDGE_LOOP('',(#6590,#6591,#6592,#6593));
#2943=EDGE_LOOP('',(#6594,#6595,#6596,#6597));
#2944=EDGE_LOOP('',(#6598,#6599,#6600));
#2945=EDGE_LOOP('',(#6601,#6602,#6603,#6604));
#2946=EDGE_LOOP('',(#6605,#6606,#6607,#6608));
#2947=EDGE_LOOP('',(#6609,#6610,#6611,#6612,#6613));
#2948=EDGE_LOOP('',(#6614,#6615,#6616,#6617,#6618,#6619,#6620,#6621,#6622,
#6623));
#2949=EDGE_LOOP('',(#6624,#6625,#6626,#6627,#6628,#6629,#6630));
#2950=EDGE_LOOP('',(#6631,#6632,#6633,#6634));
#2951=EDGE_LOOP('',(#6635,#6636,#6637,#6638));
#2952=EDGE_LOOP('',(#6639,#6640,#6641,#6642));
#2953=EDGE_LOOP('',(#6643,#6644,#6645,#6646));
#2954=EDGE_LOOP('',(#6647,#6648,#6649,#6650));
#2955=EDGE_LOOP('',(#6651,#6652,#6653));
#2956=EDGE_LOOP('',(#6654,#6655,#6656));
#2957=EDGE_LOOP('',(#6657,#6658,#6659,#6660));
#2958=EDGE_LOOP('',(#6661,#6662,#6663,#6664,#6665));
#2959=EDGE_LOOP('',(#6666,#6667,#6668,#6669,#6670));
#2960=EDGE_LOOP('',(#6671,#6672,#6673,#6674));
#2961=EDGE_LOOP('',(#6675,#6676,#6677,#6678,#6679,#6680,#6681,#6682,#6683));
#2962=EDGE_LOOP('',(#6684,#6685,#6686,#6687,#6688));
#2963=EDGE_LOOP('',(#6689,#6690,#6691,#6692));
#2964=EDGE_LOOP('',(#6693,#6694,#6695,#6696,#6697,#6698,#6699,#6700));
#2965=EDGE_LOOP('',(#6701,#6702,#6703,#6704,#6705));
#2966=EDGE_LOOP('',(#6706,#6707,#6708,#6709));
#2967=EDGE_LOOP('',(#6710,#6711,#6712));
#2968=EDGE_LOOP('',(#6713,#6714,#6715,#6716));
#2969=EDGE_LOOP('',(#6717,#6718,#6719,#6720));
#2970=EDGE_LOOP('',(#6721,#6722,#6723,#6724,#6725));
#2971=EDGE_LOOP('',(#6726,#6727,#6728,#6729));
#2972=EDGE_LOOP('',(#6730,#6731,#6732,#6733,#6734));
#2973=EDGE_LOOP('',(#6735,#6736,#6737,#6738));
#2974=EDGE_LOOP('',(#6739,#6740,#6741,#6742));
#2975=EDGE_LOOP('',(#6743,#6744,#6745,#6746));
#2976=EDGE_LOOP('',(#6747,#6748,#6749,#6750));
#2977=EDGE_LOOP('',(#6751,#6752,#6753,#6754));
#2978=EDGE_LOOP('',(#6755,#6756,#6757,#6758));
#2979=EDGE_LOOP('',(#6759,#6760,#6761,#6762,#6763));
#2980=EDGE_LOOP('',(#6764,#6765,#6766,#6767,#6768));
#2981=EDGE_LOOP('',(#6769,#6770,#6771,#6772,#6773));
#2982=EDGE_LOOP('',(#6774,#6775,#6776,#6777));
#2983=EDGE_LOOP('',(#6778,#6779,#6780,#6781));
#2984=EDGE_LOOP('',(#6782,#6783,#6784,#6785,#6786));
#2985=EDGE_LOOP('',(#6787,#6788,#6789,#6790));
#2986=EDGE_LOOP('',(#6791,#6792,#6793,#6794));
#2987=EDGE_LOOP('',(#6795,#6796,#6797,#6798));
#2988=EDGE_LOOP('',(#6799,#6800,#6801,#6802));
#2989=EDGE_LOOP('',(#6803,#6804,#6805,#6806));
#2990=EDGE_LOOP('',(#6807,#6808,#6809,#6810));
#2991=EDGE_LOOP('',(#6811,#6812,#6813,#6814));
#2992=EDGE_LOOP('',(#6815,#6816,#6817,#6818));
#2993=EDGE_LOOP('',(#6819,#6820,#6821,#6822,#6823));
#2994=EDGE_LOOP('',(#6824,#6825,#6826,#6827));
#2995=EDGE_LOOP('',(#6828,#6829,#6830,#6831));
#2996=EDGE_LOOP('',(#6832,#6833,#6834,#6835));
#2997=EDGE_LOOP('',(#6836,#6837,#6838,#6839,#6840,#6841,#6842,#6843));
#2998=EDGE_LOOP('',(#6844,#6845,#6846,#6847,#6848,#6849));
#2999=EDGE_LOOP('',(#6850,#6851,#6852,#6853));
#3000=EDGE_LOOP('',(#6854,#6855,#6856,#6857));
#3001=EDGE_LOOP('',(#6858,#6859,#6860,#6861));
#3002=EDGE_LOOP('',(#6862,#6863,#6864,#6865));
#3003=EDGE_LOOP('',(#6866,#6867,#6868,#6869));
#3004=EDGE_LOOP('',(#6870,#6871,#6872,#6873,#6874,#6875,#6876,#6877,#6878,
#6879,#6880,#6881,#6882,#6883,#6884,#6885,#6886,#6887,#6888));
#3005=EDGE_LOOP('',(#6889));
#3006=EDGE_LOOP('',(#6890));
#3007=EDGE_LOOP('',(#6891));
#3008=EDGE_LOOP('',(#6892));
#3009=EDGE_LOOP('',(#6893,#6894,#6895,#6896));
#3010=EDGE_LOOP('',(#6897,#6898,#6899,#6900));
#3011=EDGE_LOOP('',(#6901,#6902,#6903,#6904));
#3012=EDGE_LOOP('',(#6905,#6906,#6907));
#3013=EDGE_LOOP('',(#6908,#6909,#6910));
#3014=EDGE_LOOP('',(#6911,#6912,#6913,#6914));
#3015=EDGE_LOOP('',(#6915,#6916,#6917,#6918,#6919));
#3016=EDGE_LOOP('',(#6920,#6921,#6922,#6923,#6924));
#3017=EDGE_LOOP('',(#6925,#6926,#6927,#6928,#6929,#6930,#6931,#6932,#6933,
#6934,#6935,#6936,#6937,#6938,#6939,#6940,#6941,#6942,#6943,#6944,#6945,
#6946,#6947,#6948,#6949,#6950,#6951));
#3018=EDGE_LOOP('',(#6952));
#3019=EDGE_LOOP('',(#6953));
#3020=EDGE_LOOP('',(#6954));
#3021=EDGE_LOOP('',(#6955));
#3022=EDGE_LOOP('',(#6956,#6957,#6958,#6959));
#3023=EDGE_LOOP('',(#6960,#6961,#6962,#6963));
#3024=EDGE_LOOP('',(#6964,#6965,#6966,#6967));
#3025=EDGE_LOOP('',(#6968,#6969,#6970,#6971));
#3026=EDGE_LOOP('',(#6972,#6973,#6974,#6975));
#3027=EDGE_LOOP('',(#6976,#6977,#6978));
#3028=EDGE_LOOP('',(#6979,#6980,#6981));
#3029=EDGE_LOOP('',(#6982,#6983,#6984,#6985));
#3030=EDGE_LOOP('',(#6986,#6987,#6988,#6989));
#3031=EDGE_LOOP('',(#6990,#6991,#6992,#6993,#6994,#6995));
#3032=EDGE_LOOP('',(#6996,#6997,#6998,#6999,#7000,#7001,#7002,#7003,#7004,
#7005,#7006,#7007,#7008,#7009));
#3033=EDGE_LOOP('',(#7010,#7011,#7012,#7013,#7014));
#3034=EDGE_LOOP('',(#7015,#7016,#7017,#7018));
#3035=EDGE_LOOP('',(#7019,#7020,#7021,#7022,#7023));
#3036=EDGE_LOOP('',(#7024,#7025,#7026,#7027,#7028));
#3037=EDGE_LOOP('',(#7029,#7030,#7031,#7032,#7033,#7034,#7035,#7036));
#3038=EDGE_LOOP('',(#7037,#7038,#7039,#7040,#7041));
#3039=EDGE_LOOP('',(#7042,#7043,#7044));
#3040=EDGE_LOOP('',(#7045,#7046,#7047));
#3041=EDGE_LOOP('',(#7048,#7049,#7050,#7051));
#3042=EDGE_LOOP('',(#7052,#7053,#7054,#7055));
#3043=EDGE_LOOP('',(#7056,#7057,#7058,#7059,#7060));
#3044=EDGE_LOOP('',(#7061,#7062,#7063,#7064,#7065));
#3045=EDGE_LOOP('',(#7066,#7067,#7068,#7069));
#3046=EDGE_LOOP('',(#7070,#7071,#7072,#7073,#7074,#7075));
#3047=EDGE_LOOP('',(#7076,#7077,#7078));
#3048=EDGE_LOOP('',(#7079,#7080,#7081));
#3049=EDGE_LOOP('',(#7082,#7083,#7084,#7085));
#3050=EDGE_LOOP('',(#7086,#7087,#7088,#7089));
#3051=EDGE_LOOP('',(#7090,#7091,#7092,#7093,#7094,#7095));
#3052=EDGE_LOOP('',(#7096,#7097,#7098,#7099));
#3053=EDGE_LOOP('',(#7100,#7101,#7102,#7103,#7104));
#3054=EDGE_LOOP('',(#7105,#7106,#7107,#7108));
#3055=EDGE_LOOP('',(#7109,#7110,#7111,#7112));
#3056=EDGE_LOOP('',(#7113,#7114,#7115,#7116));
#3057=EDGE_LOOP('',(#7117,#7118,#7119));
#3058=EDGE_LOOP('',(#7120,#7121,#7122,#7123,#7124,#7125));
#3059=EDGE_LOOP('',(#7126,#7127,#7128,#7129));
#3060=EDGE_LOOP('',(#7130,#7131,#7132,#7133,#7134));
#3061=EDGE_LOOP('',(#7135,#7136,#7137,#7138));
#3062=EDGE_LOOP('',(#7139,#7140,#7141,#7142,#7143,#7144,#7145,#7146));
#3063=EDGE_LOOP('',(#7147,#7148,#7149,#7150,#7151,#7152,#7153));
#3064=EDGE_LOOP('',(#7154,#7155,#7156,#7157));
#3065=EDGE_LOOP('',(#7158,#7159,#7160,#7161));
#3066=EDGE_LOOP('',(#7162,#7163,#7164,#7165));
#3067=EDGE_LOOP('',(#7166,#7167,#7168,#7169));
#3068=EDGE_LOOP('',(#7170,#7171,#7172));
#3069=EDGE_LOOP('',(#7173,#7174,#7175));
#3070=EDGE_LOOP('',(#7176,#7177,#7178));
#3493=CIRCLE('',#10101,1.35);
#3494=CIRCLE('',#10102,0.1);
#3495=CIRCLE('',#10103,1.45);
#3496=CIRCLE('',#10104,1.35);
#3497=CIRCLE('',#10106,1.35);
#3498=CIRCLE('',#10107,1.35);
#3499=CIRCLE('',#10111,1.45);
#3500=CIRCLE('',#10112,0.1);
#3501=CIRCLE('',#10115,1.35);
#3502=CIRCLE('',#10116,0.1);
#3503=CIRCLE('',#10117,1.45);
#3504=CIRCLE('',#10118,1.35);
#3505=CIRCLE('',#10120,1.35);
#3506=CIRCLE('',#10121,1.35);
#3507=CIRCLE('',#10124,1.45);
#3508=CIRCLE('',#10125,0.1);
#3509=CIRCLE('',#10127,0.0799999999999994);
#3510=CIRCLE('',#10129,0.0799999999999999);
#3511=CIRCLE('',#10131,0.0799999999999997);
#3512=CIRCLE('',#10132,5.07999306553394);
#3513=CIRCLE('',#10133,4.3279926764569);
#3514=CIRCLE('',#10134,4.06447495376015);
#3515=CIRCLE('',#10135,0.08);
#3516=CIRCLE('',#10136,0.0800000000000001);
#3517=CIRCLE('',#10137,0.0799999999999998);
#3518=CIRCLE('',#10139,0.0800000000000027);
#3519=CIRCLE('',#10140,0.0800000000000007);
#3520=CIRCLE('',#10141,0.0800000000000003);
#3521=CIRCLE('',#10142,0.0799999999999987);
#3522=CIRCLE('',#10143,0.0799999999999991);
#3523=CIRCLE('',#10144,0.0800000000000008);
#3524=CIRCLE('',#10145,10.2333842526355);
#3525=CIRCLE('',#10146,42.0215436445756);
#3526=CIRCLE('',#10147,0.0800000000000006);
#3527=CIRCLE('',#10149,0.0800261246651755);
#3528=CIRCLE('',#10150,0.0800000000000003);
#3529=CIRCLE('',#10151,0.0799999999999982);
#3530=CIRCLE('',#10152,0.0799999999999997);
#3531=CIRCLE('',#10153,0.0800000000000006);
#3532=CIRCLE('',#10154,0.08);
#3533=CIRCLE('',#10155,0.0800000000000001);
#3534=CIRCLE('',#10156,1.70356712371079);
#3535=CIRCLE('',#10157,0.0799999999999989);
#3536=CIRCLE('',#10158,0.0799999999999979);
#3537=CIRCLE('',#10159,0.0800000000000002);
#3538=CIRCLE('',#10162,0.0785861158743583);
#3539=CIRCLE('',#10164,0.0800000000000012);
#3540=CIRCLE('',#10166,0.0796968010654983);
#3541=CIRCLE('',#10167,0.900090261485887);
#3542=CIRCLE('',#10168,0.08);
#3543=CIRCLE('',#10169,0.0800000001034237);
#3544=CIRCLE('',#10170,0.0800000000000002);
#3545=CIRCLE('',#10171,0.0800000000000002);
#3546=CIRCLE('',#10172,0.08);
#3547=CIRCLE('',#10173,0.0800000000013423);
#3548=CIRCLE('',#10174,0.0800000000000002);
#3549=CIRCLE('',#10175,0.08);
#3550=CIRCLE('',#10176,0.160164856730608);
#3551=CIRCLE('',#10179,0.0800000000000005);
#3552=CIRCLE('',#10181,0.0786789453077166);
#3553=CIRCLE('',#10182,0.400861721832437);
#3554=CIRCLE('',#10185,0.0800261745356576);
#3555=CIRCLE('',#10186,0.0799999999999995);
#3556=CIRCLE('',#10187,0.08);
#3557=CIRCLE('',#10188,0.0800000000000001);
#3558=CIRCLE('',#10189,0.08);
#3559=CIRCLE('',#10190,0.0800000000000003);
#3560=CIRCLE('',#10191,0.0800000000000001);
#3561=CIRCLE('',#10192,0.0800000000000005);
#3562=CIRCLE('',#10193,0.0799999999999994);
#3563=CIRCLE('',#10194,0.0799999999999999);
#3564=CIRCLE('',#10195,0.0800000000000008);
#3565=CIRCLE('',#10196,0.0798672614997588);
#3566=CIRCLE('',#10197,0.159293405838516);
#3567=CIRCLE('',#10198,0.0799999999999999);
#3568=CIRCLE('',#10199,0.0799999999999984);
#3569=CIRCLE('',#10201,0.08);
#3570=CIRCLE('',#10202,0.0800000000000024);
#3571=CIRCLE('',#10205,0.08);
#3572=CIRCLE('',#10208,0.08);
#3573=CIRCLE('',#10209,0.0799999999999999);
#3574=CIRCLE('',#10210,0.0800000000000002);
#3575=CIRCLE('',#10211,0.08);
#3576=CIRCLE('',#10212,0.0800000000000001);
#3577=CIRCLE('',#10213,0.160172033197375);
#3578=CIRCLE('',#10215,0.0800000000000002);
#3579=CIRCLE('',#10216,0.0800000000000001);
#3580=CIRCLE('',#10218,0.160207196111625);
#3581=CIRCLE('',#10220,0.0799999999999994);
#3582=CIRCLE('',#10221,0.080000000000001);
#3583=CIRCLE('',#10222,0.08);
#3584=CIRCLE('',#10223,0.0799999999999999);
#3585=CIRCLE('',#10226,0.160052182261364);
#3586=CIRCLE('',#10228,0.3);
#3587=CIRCLE('',#10229,0.36);
#3588=CIRCLE('',#10230,0.36);
#3589=CIRCLE('',#10231,0.3);
#3590=CIRCLE('',#10233,0.0800000000000003);
#3591=CIRCLE('',#10235,0.0800000000000001);
#3592=CIRCLE('',#10236,0.0800000000000003);
#3593=CIRCLE('',#10238,0.08);
#3594=CIRCLE('',#10240,0.0800000000000002);
#3595=CIRCLE('',#10242,0.0800000000000002);
#3596=CIRCLE('',#10244,0.0800000000000001);
#3597=CIRCLE('',#10248,0.3);
#3598=CIRCLE('',#10249,0.36);
#3599=CIRCLE('',#10250,0.36);
#3600=CIRCLE('',#10251,0.3);
#3601=CIRCLE('',#10252,0.0799999999999996);
#3602=CIRCLE('',#10253,0.0800260911298561);
#3603=CIRCLE('',#10254,0.0800000000000002);
#3604=CIRCLE('',#10255,0.0800000000000007);
#3605=CIRCLE('',#10256,0.0799999999999999);
#3606=CIRCLE('',#10258,0.0800000000000018);
#3607=CIRCLE('',#10261,0.0800000000000009);
#3608=CIRCLE('',#10263,0.264924618445784);
#3609=CIRCLE('',#10265,0.999721614072078);
#3610=CIRCLE('',#10266,0.08);
#3611=CIRCLE('',#10269,0.0799999999999983);
#3612=CIRCLE('',#10271,0.159956770110596);
#3613=CIRCLE('',#10274,0.0800000000000106);
#3614=CIRCLE('',#10275,0.0799999999999999);
#3615=CIRCLE('',#10276,0.487504928302448);
#3616=CIRCLE('',#10278,0.0799999999999999);
#3617=CIRCLE('',#10279,0.0661513100184898);
#3618=CIRCLE('',#10280,0.0799999999999999);
#3619=CIRCLE('',#10281,0.0799999999999998);
#3620=CIRCLE('',#10283,0.0800000000000001);
#3621=CIRCLE('',#10284,0.0800000000000001);
#3622=CIRCLE('',#10287,0.0800000000000004);
#3623=CIRCLE('',#10288,0.0799999999999999);
#3624=CIRCLE('',#10289,0.0799999999999998);
#3625=CIRCLE('',#10290,0.0799999999999995);
#3895=VERTEX_POINT('',#13220);
#3896=VERTEX_POINT('',#13221);
#3897=VERTEX_POINT('',#13223);
#3898=VERTEX_POINT('',#13228);
#3899=VERTEX_POINT('',#13230);
#3900=VERTEX_POINT('',#13234);
#3901=VERTEX_POINT('',#13235);
#3902=VERTEX_POINT('',#13237);
#3903=VERTEX_POINT('',#13242);
#3904=VERTEX_POINT('',#13244);
#3905=VERTEX_POINT('',#13246);
#3906=VERTEX_POINT('',#13283);
#3907=VERTEX_POINT('',#13287);
#3908=VERTEX_POINT('',#13288);
#3909=VERTEX_POINT('',#13293);
#3910=VERTEX_POINT('',#13298);
#3911=VERTEX_POINT('',#13305);
#3912=VERTEX_POINT('',#13307);
#3913=VERTEX_POINT('',#13314);
#3914=VERTEX_POINT('',#13320);
#3915=VERTEX_POINT('',#13390);
#3916=VERTEX_POINT('',#13405);
#3917=VERTEX_POINT('',#13406);
#3918=VERTEX_POINT('',#13408);
#3919=VERTEX_POINT('',#13413);
#3920=VERTEX_POINT('',#13415);
#3921=VERTEX_POINT('',#13419);
#3922=VERTEX_POINT('',#13420);
#3923=VERTEX_POINT('',#13422);
#3924=VERTEX_POINT('',#13430);
#3925=VERTEX_POINT('',#13432);
#3926=VERTEX_POINT('',#13473);
#3927=VERTEX_POINT('',#13477);
#3928=VERTEX_POINT('',#13478);
#3929=VERTEX_POINT('',#13486);
#3930=VERTEX_POINT('',#13493);
#3931=VERTEX_POINT('',#13561);
#3932=VERTEX_POINT('',#13568);
#3933=VERTEX_POINT('',#13575);
#3934=VERTEX_POINT('',#13596);
#3935=VERTEX_POINT('',#13603);
#3936=VERTEX_POINT('',#13610);
#3937=VERTEX_POINT('',#13617);
#3938=VERTEX_POINT('',#13641);
#3939=VERTEX_POINT('',#13661);
#3940=VERTEX_POINT('',#13663);
#3941=VERTEX_POINT('',#13667);
#3942=VERTEX_POINT('',#14220);
#3943=VERTEX_POINT('',#14256);
#3944=VERTEX_POINT('',#14265);
#3945=VERTEX_POINT('',#14267);
#3946=VERTEX_POINT('',#14272);
#3947=VERTEX_POINT('',#14475);
#3948=VERTEX_POINT('',#14477);
#3949=VERTEX_POINT('',#14523);
#3950=VERTEX_POINT('',#14588);
#3951=VERTEX_POINT('',#14628);
#3952=VERTEX_POINT('',#14656);
#3953=VERTEX_POINT('',#14658);
#3954=VERTEX_POINT('',#14687);
#3955=VERTEX_POINT('',#14794);
#3956=VERTEX_POINT('',#14798);
#3957=VERTEX_POINT('',#14821);
#3958=VERTEX_POINT('',#14823);
#3959=VERTEX_POINT('',#14849);
#3960=VERTEX_POINT('',#14875);
#3961=VERTEX_POINT('',#14967);
#3962=VERTEX_POINT('',#14989);
#3963=VERTEX_POINT('',#15100);
#3964=VERTEX_POINT('',#15324);
#3965=VERTEX_POINT('',#15429);
#3966=VERTEX_POINT('',#15431);
#3967=VERTEX_POINT('',#15796);
#3968=VERTEX_POINT('',#15826);
#3969=VERTEX_POINT('',#15827);
#3970=VERTEX_POINT('',#15829);
#3971=VERTEX_POINT('',#15836);
#3972=VERTEX_POINT('',#15876);
#3973=VERTEX_POINT('',#15877);
#3974=VERTEX_POINT('',#15908);
#3975=VERTEX_POINT('',#15927);
#3976=VERTEX_POINT('',#15929);
#3977=VERTEX_POINT('',#15948);
#3978=VERTEX_POINT('',#15949);
#3979=VERTEX_POINT('',#16002);
#3980=VERTEX_POINT('',#16011);
#3981=VERTEX_POINT('',#16594);
#3982=VERTEX_POINT('',#16602);
#3983=VERTEX_POINT('',#16609);
#3984=VERTEX_POINT('',#16624);
#3985=VERTEX_POINT('',#16626);
#3986=VERTEX_POINT('',#16643);
#3987=VERTEX_POINT('',#16746);
#3988=VERTEX_POINT('',#16766);
#3989=VERTEX_POINT('',#16965);
#3990=VERTEX_POINT('',#16966);
#3991=VERTEX_POINT('',#16968);
#3992=VERTEX_POINT('',#16970);
#3993=VERTEX_POINT('',#16997);
#3994=VERTEX_POINT('',#16998);
#3995=VERTEX_POINT('',#17000);
#3996=VERTEX_POINT('',#17005);
#3997=VERTEX_POINT('',#17031);
#3998=VERTEX_POINT('',#17032);
#3999=VERTEX_POINT('',#17090);
#4000=VERTEX_POINT('',#17146);
#4001=VERTEX_POINT('',#17191);
#4002=VERTEX_POINT('',#17196);
#4003=VERTEX_POINT('',#17220);
#4004=VERTEX_POINT('',#17752);
#4005=VERTEX_POINT('',#17767);
#4006=VERTEX_POINT('',#17780);
#4007=VERTEX_POINT('',#17781);
#4008=VERTEX_POINT('',#18331);
#4009=VERTEX_POINT('',#18332);
#4010=VERTEX_POINT('',#18334);
#4011=VERTEX_POINT('',#18339);
#4012=VERTEX_POINT('',#18341);
#4013=VERTEX_POINT('',#18366);
#4014=VERTEX_POINT('',#18367);
#4015=VERTEX_POINT('',#18393);
#4016=VERTEX_POINT('',#18432);
#4017=VERTEX_POINT('',#18439);
#4018=VERTEX_POINT('',#18446);
#4019=VERTEX_POINT('',#18492);
#4020=VERTEX_POINT('',#18571);
#4021=VERTEX_POINT('',#18597);
#4022=VERTEX_POINT('',#18604);
#4023=VERTEX_POINT('',#18672);
#4024=VERTEX_POINT('',#18673);
#4025=VERTEX_POINT('',#18675);
#4026=VERTEX_POINT('',#18680);
#4027=VERTEX_POINT('',#18716);
#4028=VERTEX_POINT('',#18742);
#4029=VERTEX_POINT('',#18743);
#4030=VERTEX_POINT('',#18789);
#4031=VERTEX_POINT('',#18832);
#4032=VERTEX_POINT('',#18833);
#4033=VERTEX_POINT('',#18865);
#4034=VERTEX_POINT('',#18866);
#4035=VERTEX_POINT('',#18881);
#4036=VERTEX_POINT('',#18902);
#4037=VERTEX_POINT('',#19954);
#4038=VERTEX_POINT('',#20173);
#4039=VERTEX_POINT('',#20175);
#4040=VERTEX_POINT('',#20198);
#4041=VERTEX_POINT('',#20199);
#4042=VERTEX_POINT('',#20201);
#4043=VERTEX_POINT('',#20206);
#4044=VERTEX_POINT('',#20232);
#4045=VERTEX_POINT('',#20237);
#4046=VERTEX_POINT('',#20263);
#4047=VERTEX_POINT('',#20264);
#4048=VERTEX_POINT('',#20334);
#4049=VERTEX_POINT('',#20335);
#4050=VERTEX_POINT('',#20430);
#4051=VERTEX_POINT('',#20432);
#4052=VERTEX_POINT('',#20437);
#4053=VERTEX_POINT('',#20563);
#4054=VERTEX_POINT('',#20584);
#4055=VERTEX_POINT('',#20759);
#4056=VERTEX_POINT('',#20763);
#4057=VERTEX_POINT('',#20765);
#4058=VERTEX_POINT('',#20776);
#4059=VERTEX_POINT('',#20805);
#4060=VERTEX_POINT('',#20810);
#4061=VERTEX_POINT('',#20921);
#4062=VERTEX_POINT('',#20923);
#4063=VERTEX_POINT('',#21020);
#4064=VERTEX_POINT('',#21029);
#4065=VERTEX_POINT('',#21031);
#4066=VERTEX_POINT('',#21033);
#4067=VERTEX_POINT('',#21035);
#4068=VERTEX_POINT('',#21041);
#4069=VERTEX_POINT('',#21043);
#4070=VERTEX_POINT('',#21050);
#4071=VERTEX_POINT('',#21052);
#4072=VERTEX_POINT('',#21054);
#4073=VERTEX_POINT('',#21056);
#4074=VERTEX_POINT('',#21059);
#4075=VERTEX_POINT('',#21063);
#4076=VERTEX_POINT('',#21065);
#4077=VERTEX_POINT('',#21067);
#4078=VERTEX_POINT('',#21071);
#4079=VERTEX_POINT('',#21080);
#4080=VERTEX_POINT('',#21084);
#4081=VERTEX_POINT('',#21086);
#4082=VERTEX_POINT('',#21113);
#4083=VERTEX_POINT('',#21114);
#4084=VERTEX_POINT('',#21119);
#4085=VERTEX_POINT('',#21126);
#4086=VERTEX_POINT('',#21135);
#4087=VERTEX_POINT('',#21137);
#4088=VERTEX_POINT('',#21146);
#4089=VERTEX_POINT('',#21161);
#4090=VERTEX_POINT('',#21163);
#4091=VERTEX_POINT('',#21171);
#4092=VERTEX_POINT('',#21178);
#4093=VERTEX_POINT('',#21191);
#4094=VERTEX_POINT('',#21193);
#4095=VERTEX_POINT('',#21195);
#4096=VERTEX_POINT('',#21197);
#4097=VERTEX_POINT('',#21219);
#4098=VERTEX_POINT('',#21242);
#4099=VERTEX_POINT('',#21278);
#4100=VERTEX_POINT('',#21280);
#4101=VERTEX_POINT('',#21325);
#4102=VERTEX_POINT('',#21850);
#4103=VERTEX_POINT('',#21890);
#4104=VERTEX_POINT('',#21977);
#4105=VERTEX_POINT('',#22019);
#4106=VERTEX_POINT('',#22020);
#4107=VERTEX_POINT('',#22027);
#4108=VERTEX_POINT('',#22029);
#4109=VERTEX_POINT('',#22083);
#4110=VERTEX_POINT('',#22115);
#4111=VERTEX_POINT('',#22174);
#4112=VERTEX_POINT('',#22179);
#4113=VERTEX_POINT('',#22202);
#4114=VERTEX_POINT('',#22204);
#4115=VERTEX_POINT('',#22307);
#4116=VERTEX_POINT('',#22312);
#4117=VERTEX_POINT('',#22479);
#4118=VERTEX_POINT('',#22481);
#4119=VERTEX_POINT('',#22524);
#4120=VERTEX_POINT('',#22569);
#4121=VERTEX_POINT('',#22671);
#4122=VERTEX_POINT('',#22697);
#4935=EDGE_CURVE('',#3895,#3896,#3493,.T.);
#4936=EDGE_CURVE('',#3896,#3897,#3494,.T.);
#4937=EDGE_CURVE('',#3897,#3897,#3495,.T.);
#4938=EDGE_CURVE('',#3896,#3895,#3496,.T.);
#4939=EDGE_CURVE('',#3895,#3898,#1199,.T.);
#4940=EDGE_CURVE('',#3899,#3898,#3497,.T.);
#4941=EDGE_CURVE('',#3898,#3899,#3498,.T.);
#4942=EDGE_CURVE('',#3900,#3901,#1200,.T.);
#4943=EDGE_CURVE('',#3902,#3900,#490,.T.);
#4944=EDGE_CURVE('',#3903,#3902,#1201,.T.);
#4945=EDGE_CURVE('',#3904,#3903,#1202,.T.);
#4946=EDGE_CURVE('',#3905,#3904,#475,.T.);
#4947=EDGE_CURVE('',#3901,#3905,#491,.T.);
#4948=EDGE_CURVE('',#3906,#3906,#3499,.T.);
#4949=EDGE_CURVE('',#3906,#3899,#3500,.T.);
#4950=EDGE_CURVE('',#3907,#3908,#492,.T.);
#4951=EDGE_CURVE('',#3909,#3907,#493,.T.);
#4952=EDGE_CURVE('',#3910,#3909,#494,.T.);
#4953=EDGE_CURVE('',#3911,#3910,#1203,.T.);
#4954=EDGE_CURVE('',#3912,#3911,#495,.T.);
#4955=EDGE_CURVE('',#3913,#3912,#496,.T.);
#4956=EDGE_CURVE('',#3913,#3914,#497,.T.);
#4957=EDGE_CURVE('',#3914,#3915,#498,.T.);
#4958=EDGE_CURVE('',#3908,#3915,#499,.T.);
#4959=EDGE_CURVE('',#3916,#3917,#3501,.T.);
#4960=EDGE_CURVE('',#3917,#3918,#3502,.T.);
#4961=EDGE_CURVE('',#3918,#3918,#3503,.T.);
#4962=EDGE_CURVE('',#3917,#3916,#3504,.T.);
#4963=EDGE_CURVE('',#3916,#3919,#1204,.T.);
#4964=EDGE_CURVE('',#3920,#3919,#3505,.T.);
#4965=EDGE_CURVE('',#3919,#3920,#3506,.T.);
#4966=EDGE_CURVE('',#3921,#3922,#1205,.T.);
#4967=EDGE_CURVE('',#3923,#3921,#500,.T.);
#4968=EDGE_CURVE('',#3923,#3924,#1206,.T.);
#4969=EDGE_CURVE('',#3925,#3924,#501,.T.);
#4970=EDGE_CURVE('',#3922,#3925,#502,.T.);
#4971=EDGE_CURVE('',#3926,#3926,#3507,.T.);
#4972=EDGE_CURVE('',#3926,#3920,#3508,.T.);
#4973=EDGE_CURVE('',#3927,#3928,#503,.T.);
#4974=EDGE_CURVE('',#3929,#3927,#504,.T.);
#4975=EDGE_CURVE('',#3929,#3930,#505,.T.);
#4976=EDGE_CURVE('',#3931,#3930,#506,.T.);
#4977=EDGE_CURVE('',#3932,#3931,#507,.T.);
#4978=EDGE_CURVE('',#3933,#3932,#508,.T.);
#4979=EDGE_CURVE('',#3934,#3933,#509,.T.);
#4980=EDGE_CURVE('',#3935,#3934,#510,.T.);
#4981=EDGE_CURVE('',#3936,#3935,#511,.T.);
#4982=EDGE_CURVE('',#3937,#3936,#512,.T.);
#4983=EDGE_CURVE('',#3937,#3928,#1207,.T.);
#4984=EDGE_CURVE('',#3938,#3927,#513,.T.);
#4985=EDGE_CURVE('',#3938,#3939,#1208,.T.);
#4986=EDGE_CURVE('',#3939,#3940,#3509,.T.);
#4987=EDGE_CURVE('',#3940,#3929,#1209,.T.);
#4988=EDGE_CURVE('',#3921,#3941,#514,.T.);
#4989=EDGE_CURVE('',#3922,#3939,#3510,.T.);
#4990=EDGE_CURVE('',#3939,#3941,#1210,.T.);
#4991=EDGE_CURVE('',#3922,#3940,#3511,.T.);
#4992=EDGE_CURVE('',#3942,#3940,#515,.T.);
#4993=EDGE_CURVE('',#3943,#3942,#516,.T.);
#4994=EDGE_CURVE('',#3944,#3943,#3512,.T.);
#4995=EDGE_CURVE('',#3945,#3944,#517,.T.);
#4996=EDGE_CURVE('',#3946,#3945,#3513,.T.);
#4997=EDGE_CURVE('',#3930,#3946,#3514,.T.);
#4998=EDGE_CURVE('',#3925,#3942,#3515,.T.);
#4999=EDGE_CURVE('',#3947,#3924,#3516,.T.);
#5000=EDGE_CURVE('',#3924,#3948,#518,.T.);
#5001=EDGE_CURVE('',#3948,#3947,#519,.T.);
#5002=EDGE_CURVE('',#3949,#3925,#3517,.T.);
#5003=EDGE_CURVE('',#3947,#3949,#520,.T.);
#5004=EDGE_CURVE('',#3949,#3942,#3518,.T.);
#5005=EDGE_CURVE('',#3949,#3950,#521,.T.);
#5006=EDGE_CURVE('',#3943,#3950,#3519,.T.);
#5007=EDGE_CURVE('',#3948,#3951,#522,.T.);
#5008=EDGE_CURVE('',#3950,#3951,#3520,.T.);
#5009=EDGE_CURVE('',#3952,#3945,#3521,.T.);
#5010=EDGE_CURVE('',#3944,#3953,#3522,.T.);
#5011=EDGE_CURVE('',#3953,#3952,#523,.T.);
#5012=EDGE_CURVE('',#3954,#3946,#3523,.T.);
#5013=EDGE_CURVE('',#3952,#3954,#524,.T.);
#5014=EDGE_CURVE('',#3950,#3953,#3524,.T.);
#5015=EDGE_CURVE('',#3954,#3931,#525,.T.);
#5016=EDGE_CURVE('',#3951,#3955,#3525,.T.);
#5017=EDGE_CURVE('',#3955,#3953,#3526,.T.);
#5018=EDGE_CURVE('',#3956,#3923,#526,.T.);
#5019=EDGE_CURVE('',#3957,#3956,#3527,.T.);
#5020=EDGE_CURVE('',#3957,#3958,#1211,.T.);
#5021=EDGE_CURVE('',#3948,#3958,#527,.T.);
#5022=EDGE_CURVE('',#3955,#3959,#528,.T.);
#5023=EDGE_CURVE('',#3959,#3952,#3528,.T.);
#5024=EDGE_CURVE('',#3959,#3960,#529,.T.);
#5025=EDGE_CURVE('',#3960,#3954,#3529,.T.);
#5026=EDGE_CURVE('',#3960,#3934,#530,.T.);
#5027=EDGE_CURVE('',#3933,#3932,#3530,.T.);
#5028=EDGE_CURVE('',#3936,#3961,#3531,.T.);
#5029=EDGE_CURVE('',#3961,#3937,#531,.T.);
#5030=EDGE_CURVE('',#3962,#3935,#3532,.T.);
#5031=EDGE_CURVE('',#3962,#3961,#532,.T.);
#5032=EDGE_CURVE('',#3960,#3963,#533,.T.);
#5033=EDGE_CURVE('',#3963,#3964,#3533,.T.);
#5034=EDGE_CURVE('',#3964,#3962,#534,.T.);
#5035=EDGE_CURVE('',#3965,#3959,#1212,.T.);
#5036=EDGE_CURVE('',#3966,#3965,#535,.T.);
#5037=EDGE_CURVE('',#3966,#3963,#1213,.T.);
#5038=EDGE_CURVE('',#3967,#3951,#3534,.T.);
#5039=EDGE_CURVE('',#3965,#3967,#536,.T.);
#5040=EDGE_CURVE('',#3968,#3969,#3535,.T.);
#5041=EDGE_CURVE('',#3969,#3970,#537,.T.);
#5042=EDGE_CURVE('',#3970,#3971,#3536,.T.);
#5043=EDGE_CURVE('',#3971,#3968,#538,.T.);
#5044=EDGE_CURVE('',#3972,#3973,#3537,.T.);
#5045=EDGE_CURVE('',#3973,#3969,#539,.T.);
#5046=EDGE_CURVE('',#3972,#3968,#476,.T.);
#5047=EDGE_CURVE('',#3970,#3974,#477,.T.);
#5048=EDGE_CURVE('',#3974,#3971,#3538,.T.);
#5049=EDGE_CURVE('',#3975,#3972,#478,.T.);
#5050=EDGE_CURVE('',#3975,#3976,#3539,.T.);
#5051=EDGE_CURVE('',#3976,#3973,#479,.T.);
#5052=EDGE_CURVE('',#3977,#3978,#540,.T.);
#5053=EDGE_CURVE('',#3978,#3976,#541,.T.);
#5054=EDGE_CURVE('',#3975,#3977,#1214,.T.);
#5055=EDGE_CURVE('',#3973,#3979,#542,.T.);
#5056=EDGE_CURVE('',#3979,#3980,#3540,.T.);
#5057=EDGE_CURVE('',#3980,#3970,#543,.T.);
#5058=EDGE_CURVE('',#3978,#3981,#544,.T.);
#5059=EDGE_CURVE('',#3981,#3982,#545,.T.);
#5060=EDGE_CURVE('',#3982,#3983,#546,.T.);
#5061=EDGE_CURVE('',#3984,#3983,#1215,.T.);
#5062=EDGE_CURVE('',#3985,#3984,#547,.F.);
#5063=EDGE_CURVE('',#3985,#3986,#548,.T.);
#5064=EDGE_CURVE('',#3986,#3979,#3541,.T.);
#5065=EDGE_CURVE('',#3974,#3987,#549,.T.);
#5066=EDGE_CURVE('',#3987,#3988,#3542,.T.);
#5067=EDGE_CURVE('',#3988,#3975,#550,.T.);
#5068=EDGE_CURVE('',#3989,#3990,#3543,.F.);
#5069=EDGE_CURVE('',#3991,#3990,#3544,.T.);
#5070=EDGE_CURVE('',#3991,#3992,#3545,.T.);
#5071=EDGE_CURVE('',#3992,#3989,#551,.T.);
#5072=EDGE_CURVE('',#3993,#3994,#3546,.T.);
#5073=EDGE_CURVE('',#3994,#3995,#552,.T.);
#5074=EDGE_CURVE('',#3995,#3996,#3547,.T.);
#5075=EDGE_CURVE('',#3996,#3993,#553,.T.);
#5076=EDGE_CURVE('',#3997,#3998,#3548,.T.);
#5077=EDGE_CURVE('',#3998,#3996,#554,.T.);
#5078=EDGE_CURVE('',#3995,#3997,#555,.T.);
#5079=EDGE_CURVE('',#3993,#3992,#556,.T.);
#5080=EDGE_CURVE('',#3991,#3994,#557,.T.);
#5081=EDGE_CURVE('',#3999,#3987,#3549,.T.);
#5082=EDGE_CURVE('',#3987,#3998,#3550,.T.);
#5083=EDGE_CURVE('',#3997,#3999,#480,.T.);
#5084=EDGE_CURVE('',#3999,#3988,#3551,.T.);
#5085=EDGE_CURVE('',#3998,#3974,#1216,.T.);
#5086=EDGE_CURVE('',#4000,#3988,#558,.T.);
#5087=EDGE_CURVE('',#3977,#4000,#559,.T.);
#5088=EDGE_CURVE('',#3999,#4001,#560,.T.);
#5089=EDGE_CURVE('',#4001,#4002,#3552,.T.);
#5090=EDGE_CURVE('',#4002,#4000,#561,.T.);
#5091=EDGE_CURVE('',#3995,#4003,#562,.T.);
#5092=EDGE_CURVE('',#4003,#4001,#563,.T.);
#5093=EDGE_CURVE('',#4004,#3994,#1217,.T.);
#5094=EDGE_CURVE('',#4004,#4003,#3553,.T.);
#5095=EDGE_CURVE('',#3992,#3986,#1218,.T.);
#5096=EDGE_CURVE('',#3990,#4005,#1219,.T.);
#5097=EDGE_CURVE('',#4004,#4005,#564,.F.);
#5098=EDGE_CURVE('',#4006,#4007,#3554,.T.);
#5099=EDGE_CURVE('',#4007,#3957,#1220,.T.);
#5100=EDGE_CURVE('',#3956,#4006,#1221,.T.);
#5101=EDGE_CURVE('',#3938,#3941,#565,.T.);
#5102=EDGE_CURVE('',#3928,#4006,#566,.T.);
#5103=EDGE_CURVE('',#4008,#4009,#3555,.T.);
#5104=EDGE_CURVE('',#4009,#4010,#567,.T.);
#5105=EDGE_CURVE('',#4010,#4011,#3556,.T.);
#5106=EDGE_CURVE('',#4011,#4012,#568,.T.);
#5107=EDGE_CURVE('',#4008,#4012,#569,.T.);
#5108=EDGE_CURVE('',#4013,#4014,#3557,.T.);
#5109=EDGE_CURVE('',#4014,#4011,#570,.T.);
#5110=EDGE_CURVE('',#4010,#4013,#571,.T.);
#5111=EDGE_CURVE('',#4015,#4008,#572,.F.);
#5112=EDGE_CURVE('',#4015,#4009,#573,.T.);
#5113=EDGE_CURVE('',#4016,#3910,#574,.T.);
#5114=EDGE_CURVE('',#3910,#4017,#575,.T.);
#5115=EDGE_CURVE('',#4017,#4018,#576,.T.);
#5116=EDGE_CURVE('',#4018,#4016,#3558,.T.);
#5117=EDGE_CURVE('',#4018,#4014,#577,.T.);
#5118=EDGE_CURVE('',#4013,#4016,#578,.T.);
#5119=EDGE_CURVE('',#4012,#4019,#579,.F.);
#5120=EDGE_CURVE('',#3907,#4011,#3559,.T.);
#5121=EDGE_CURVE('',#3908,#4019,#580,.T.);
#5122=EDGE_CURVE('',#4014,#3909,#3560,.T.);
#5123=EDGE_CURVE('',#4015,#4020,#581,.T.);
#5124=EDGE_CURVE('',#4020,#4021,#582,.T.);
#5125=EDGE_CURVE('',#4021,#4022,#583,.T.);
#5126=EDGE_CURVE('',#4022,#4015,#584,.T.);
#5127=EDGE_CURVE('',#4023,#4024,#3561,.T.);
#5128=EDGE_CURVE('',#4024,#4025,#585,.T.);
#5129=EDGE_CURVE('',#4025,#4026,#3562,.T.);
#5130=EDGE_CURVE('',#4026,#4023,#586,.T.);
#5131=EDGE_CURVE('',#4023,#3912,#587,.T.);
#5132=EDGE_CURVE('',#3912,#4027,#3563,.T.);
#5133=EDGE_CURVE('',#4027,#4024,#588,.T.);
#5134=EDGE_CURVE('',#4028,#4029,#3564,.T.);
#5135=EDGE_CURVE('',#4029,#4026,#3565,.T.);
#5136=EDGE_CURVE('',#4025,#4028,#3566,.T.);
#5137=EDGE_CURVE('',#4030,#3911,#589,.F.);
#5138=EDGE_CURVE('',#4030,#4027,#590,.T.);
#5139=EDGE_CURVE('',#4031,#4032,#3567,.T.);
#5140=EDGE_CURVE('',#4032,#4029,#591,.T.);
#5141=EDGE_CURVE('',#4028,#4031,#592,.T.);
#5142=EDGE_CURVE('',#4033,#4034,#593,.T.);
#5143=EDGE_CURVE('',#4033,#4032,#594,.T.);
#5144=EDGE_CURVE('',#4031,#4035,#595,.T.);
#5145=EDGE_CURVE('',#4034,#4035,#596,.T.);
#5146=EDGE_CURVE('',#4026,#4036,#3568,.T.);
#5147=EDGE_CURVE('',#4036,#3913,#1222,.T.);
#5148=EDGE_CURVE('',#3901,#4032,#3569,.T.);
#5149=EDGE_CURVE('',#3901,#4036,#3570,.T.);
#5150=EDGE_CURVE('',#3900,#4033,#481,.T.);
#5151=EDGE_CURVE('',#4034,#3902,#597,.T.);
#5152=EDGE_CURVE('',#4037,#4036,#598,.T.);
#5153=EDGE_CURVE('',#3915,#4037,#599,.T.);
#5154=EDGE_CURVE('',#3905,#4037,#3571,.T.);
#5155=EDGE_CURVE('',#3903,#4035,#600,.F.);
#5156=EDGE_CURVE('',#3989,#4038,#1223,.T.);
#5157=EDGE_CURVE('',#4038,#4039,#3572,.T.);
#5158=EDGE_CURVE('',#4039,#3990,#1224,.T.);
#5159=EDGE_CURVE('',#4040,#4041,#3573,.T.);
#5160=EDGE_CURVE('',#4041,#4042,#601,.T.);
#5161=EDGE_CURVE('',#4042,#4043,#3574,.T.);
#5162=EDGE_CURVE('',#4043,#4040,#602,.T.);
#5163=EDGE_CURVE('',#4042,#4044,#603,.T.);
#5164=EDGE_CURVE('',#4044,#4045,#3575,.T.);
#5165=EDGE_CURVE('',#4045,#4043,#604,.T.);
#5166=EDGE_CURVE('',#4046,#4047,#3576,.T.);
#5167=EDGE_CURVE('',#4047,#4041,#605,.T.);
#5168=EDGE_CURVE('',#4040,#4046,#606,.T.);
#5169=EDGE_CURVE('',#4044,#4039,#607,.T.);
#5170=EDGE_CURVE('',#4038,#4045,#608,.T.);
#5171=EDGE_CURVE('',#4048,#4049,#609,.T.);
#5172=EDGE_CURVE('',#4049,#4047,#610,.T.);
#5173=EDGE_CURVE('',#4046,#4048,#3577,.T.);
#5174=EDGE_CURVE('',#4050,#4041,#482,.T.);
#5175=EDGE_CURVE('',#4051,#4050,#611,.T.);
#5176=EDGE_CURVE('',#4052,#4051,#612,.T.);
#5177=EDGE_CURVE('',#4042,#4052,#1225,.T.);
#5178=EDGE_CURVE('',#4049,#4050,#3578,.T.);
#5179=EDGE_CURVE('',#4048,#4053,#613,.T.);
#5180=EDGE_CURVE('',#4053,#4054,#3579,.T.);
#5181=EDGE_CURVE('',#4054,#4049,#614,.T.);
#5182=EDGE_CURVE('',#4055,#4046,#1226,.T.);
#5183=EDGE_CURVE('',#4053,#4055,#3580,.T.);
#5184=EDGE_CURVE('',#4056,#4045,#1227,.T.);
#5185=EDGE_CURVE('',#4057,#4056,#615,.T.);
#5186=EDGE_CURVE('',#4058,#4057,#616,.T.);
#5187=EDGE_CURVE('',#4055,#4058,#617,.T.);
#5188=EDGE_CURVE('',#4028,#4059,#618,.T.);
#5189=EDGE_CURVE('',#4059,#4060,#3581,.T.);
#5190=EDGE_CURVE('',#4060,#3903,#619,.T.);
#5191=EDGE_CURVE('',#3965,#4061,#3582,.T.);
#5192=EDGE_CURVE('',#4061,#4062,#620,.T.);
#5193=EDGE_CURVE('',#4062,#3966,#3583,.T.);
#5194=EDGE_CURVE('',#4062,#4060,#621,.T.);
#5195=EDGE_CURVE('',#4059,#3966,#622,.T.);
#5196=EDGE_CURVE('',#3958,#3967,#3584,.T.);
#5197=EDGE_CURVE('',#3958,#4061,#623,.T.);
#5198=EDGE_CURVE('',#4063,#4060,#1228,.T.);
#5199=EDGE_CURVE('',#3904,#4063,#624,.T.);
#5200=EDGE_CURVE('',#4064,#3985,#1229,.T.);
#5201=EDGE_CURVE('',#4065,#4064,#1230,.T.);
#5202=EDGE_CURVE('',#4066,#4065,#3585,.T.);
#5203=EDGE_CURVE('',#4067,#4066,#625,.T.);
#5204=EDGE_CURVE('',#4063,#4067,#483,.T.);
#5205=EDGE_CURVE('',#4068,#3957,#1231,.T.);
#5206=EDGE_CURVE('',#4069,#4068,#626,.T.);
#5207=EDGE_CURVE('',#4069,#4056,#1232,.T.);
#5208=EDGE_CURVE('',#4070,#4070,#3586,.T.);
#5209=EDGE_CURVE('',#4071,#4071,#3587,.T.);
#5210=EDGE_CURVE('',#4072,#4072,#3588,.T.);
#5211=EDGE_CURVE('',#4073,#4073,#3589,.T.);
#5212=EDGE_CURVE('',#3984,#4074,#1233,.T.);
#5213=EDGE_CURVE('',#4074,#4064,#3590,.T.);
#5214=EDGE_CURVE('',#4075,#4074,#3591,.T.);
#5215=EDGE_CURVE('',#4074,#4076,#1234,.T.);
#5216=EDGE_CURVE('',#4076,#4077,#3592,.T.);
#5217=EDGE_CURVE('',#4077,#4075,#1235,.T.);
#5218=EDGE_CURVE('',#3982,#4078,#1236,.T.);
#5219=EDGE_CURVE('',#4078,#4076,#3593,.T.);
#5220=EDGE_CURVE('',#4076,#3983,#1237,.T.);
#5221=EDGE_CURVE('',#4078,#4077,#3594,.T.);
#5222=EDGE_CURVE('',#4075,#4064,#3595,.T.);
#5223=EDGE_CURVE('',#4075,#4079,#1238,.T.);
#5224=EDGE_CURVE('',#4079,#4065,#3596,.T.);
#5225=EDGE_CURVE('',#4080,#4077,#1239,.T.);
#5226=EDGE_CURVE('',#4080,#4081,#627,.T.);
#5227=EDGE_CURVE('',#4079,#4081,#1240,.T.);
#5228=EDGE_CURVE('',#4078,#4022,#1241,.T.);
#5229=EDGE_CURVE('',#4021,#4080,#628,.T.);
#5230=EDGE_CURVE('',#4082,#4083,#629,.T.);
#5231=EDGE_CURVE('',#4083,#4084,#630,.T.);
#5232=EDGE_CURVE('',#4084,#4085,#631,.T.);
#5233=EDGE_CURVE('',#4085,#4086,#1242,.T.);
#5234=EDGE_CURVE('',#4087,#4086,#632,.T.);
#5235=EDGE_CURVE('',#4087,#4088,#633,.F.);
#5236=EDGE_CURVE('',#4088,#4089,#1243,.T.);
#5237=EDGE_CURVE('',#4090,#4089,#634,.T.);
#5238=EDGE_CURVE('',#4090,#4007,#1244,.T.);
#5239=EDGE_CURVE('',#4007,#3961,#1245,.T.);
#5240=EDGE_CURVE('',#4091,#3964,#635,.T.);
#5241=EDGE_CURVE('',#4091,#4016,#1246,.T.);
#5242=EDGE_CURVE('',#3981,#4005,#1247,.T.);
#5243=EDGE_CURVE('',#4005,#4092,#1248,.T.);
#5244=EDGE_CURVE('',#4092,#4052,#636,.T.);
#5245=EDGE_CURVE('',#4051,#4082,#637,.T.);
#5246=EDGE_CURVE('',#4093,#4093,#3597,.T.);
#5247=EDGE_CURVE('',#4094,#4094,#3598,.T.);
#5248=EDGE_CURVE('',#4095,#4095,#3599,.T.);
#5249=EDGE_CURVE('',#4096,#4096,#3600,.T.);
#5250=EDGE_CURVE('',#4097,#4066,#3601,.T.);
#5251=EDGE_CURVE('',#4079,#4097,#3602,.T.);
#5252=EDGE_CURVE('',#4098,#4067,#3603,.T.);
#5253=EDGE_CURVE('',#4097,#4098,#638,.T.);
#5254=EDGE_CURVE('',#4063,#4099,#3604,.T.);
#5255=EDGE_CURVE('',#4099,#4100,#639,.T.);
#5256=EDGE_CURVE('',#4100,#3904,#3605,.T.);
#5257=EDGE_CURVE('',#4098,#4099,#484,.T.);
#5258=EDGE_CURVE('',#4101,#3905,#3606,.T.);
#5259=EDGE_CURVE('',#4100,#4101,#485,.T.);
#5260=EDGE_CURVE('',#4101,#4037,#3607,.T.);
#5261=EDGE_CURVE('',#4102,#4097,#1249,.T.);
#5262=EDGE_CURVE('',#4098,#4102,#640,.T.);
#5263=EDGE_CURVE('',#4081,#4102,#3608,.T.);
#5264=EDGE_CURVE('',#4101,#4103,#641,.T.);
#5265=EDGE_CURVE('',#4019,#4103,#642,.F.);
#5266=EDGE_CURVE('',#4030,#4091,#3609,.T.);
#5267=EDGE_CURVE('',#4091,#4104,#3610,.T.);
#5268=EDGE_CURVE('',#4104,#4024,#643,.T.);
#5269=EDGE_CURVE('',#3963,#4104,#644,.T.);
#5270=EDGE_CURVE('',#4105,#4106,#645,.T.);
#5271=EDGE_CURVE('',#4106,#4107,#1250,.T.);
#5272=EDGE_CURVE('',#4107,#4108,#646,.T.);
#5273=EDGE_CURVE('',#4108,#4069,#647,.T.);
#5274=EDGE_CURVE('',#4068,#4090,#1251,.T.);
#5275=EDGE_CURVE('',#4089,#4105,#648,.T.);
#5276=EDGE_CURVE('',#4105,#4088,#1252,.T.);
#5277=EDGE_CURVE('',#4087,#4109,#649,.T.);
#5278=EDGE_CURVE('',#4106,#4109,#3611,.T.);
#5279=EDGE_CURVE('',#4056,#4108,#3612,.T.);
#5280=EDGE_CURVE('',#4109,#4110,#1253,.T.);
#5281=EDGE_CURVE('',#4110,#4107,#3613,.T.);
#5282=EDGE_CURVE('',#4110,#4057,#650,.T.);
#5283=EDGE_CURVE('',#4086,#4111,#651,.T.);
#5284=EDGE_CURVE('',#4112,#4111,#3614,.T.);
#5285=EDGE_CURVE('',#4112,#4109,#3615,.T.);
#5286=EDGE_CURVE('',#4111,#4113,#486,.T.);
#5287=EDGE_CURVE('',#4113,#4114,#3616,.T.);
#5288=EDGE_CURVE('',#4114,#4112,#3617,.T.);
#5289=EDGE_CURVE('',#4083,#4115,#652,.T.);
#5290=EDGE_CURVE('',#4115,#4116,#653,.T.);
#5291=EDGE_CURVE('',#4116,#4117,#3618,.T.);
#5292=EDGE_CURVE('',#4117,#4118,#654,.T.);
#5293=EDGE_CURVE('',#4118,#4084,#3619,.T.);
#5294=EDGE_CURVE('',#4118,#4085,#655,.T.);
#5295=EDGE_CURVE('',#4116,#4119,#3620,.T.);
#5296=EDGE_CURVE('',#4119,#4117,#3621,.T.);
#5297=EDGE_CURVE('',#4119,#4114,#487,.T.);
#5298=EDGE_CURVE('',#4113,#4117,#488,.T.);
#5299=EDGE_CURVE('',#4116,#4054,#656,.T.);
#5300=EDGE_CURVE('',#4120,#4054,#3622,.T.);
#5301=EDGE_CURVE('',#4120,#4119,#657,.T.);
#5302=EDGE_CURVE('',#4049,#4082,#1254,.T.);
#5303=EDGE_CURVE('',#4092,#4039,#1255,.T.);
#5304=EDGE_CURVE('',#4110,#4121,#658,.T.);
#5305=EDGE_CURVE('',#4121,#4058,#3623,.T.);
#5306=EDGE_CURVE('',#4122,#4055,#3624,.T.);
#5307=EDGE_CURVE('',#4121,#4122,#659,.T.);
#5308=EDGE_CURVE('',#4120,#4053,#3625,.T.);
#5309=EDGE_CURVE('',#4122,#4120,#489,.T.);
#5310=EDGE_CURVE('',#4121,#4112,#660,.T.);
#5311=EDGE_CURVE('',#4113,#4118,#1256,.T.);
#5312=EDGE_CURVE('',#4002,#3977,#1257,.T.);
#5313=EDGE_CURVE('',#4073,#4093,#1258,.T.);
#5314=EDGE_CURVE('',#4072,#4094,#1259,.T.);
#5315=EDGE_CURVE('',#4071,#4095,#1260,.T.);
#5316=EDGE_CURVE('',#4070,#4096,#1261,.T.);
#6415=ORIENTED_EDGE('',*,*,#4935,.T.);
#6416=ORIENTED_EDGE('',*,*,#4936,.T.);
#6417=ORIENTED_EDGE('',*,*,#4937,.T.);
#6418=ORIENTED_EDGE('',*,*,#4936,.F.);
#6419=ORIENTED_EDGE('',*,*,#4938,.T.);
#6420=ORIENTED_EDGE('',*,*,#4935,.F.);
#6421=ORIENTED_EDGE('',*,*,#4939,.T.);
#6422=ORIENTED_EDGE('',*,*,#4940,.F.);
#6423=ORIENTED_EDGE('',*,*,#4941,.F.);
#6424=ORIENTED_EDGE('',*,*,#4939,.F.);
#6425=ORIENTED_EDGE('',*,*,#4938,.F.);
#6426=ORIENTED_EDGE('',*,*,#4942,.F.);
#6427=ORIENTED_EDGE('',*,*,#4943,.F.);
#6428=ORIENTED_EDGE('',*,*,#4944,.F.);
#6429=ORIENTED_EDGE('',*,*,#4945,.F.);
#6430=ORIENTED_EDGE('',*,*,#4946,.F.);
#6431=ORIENTED_EDGE('',*,*,#4947,.F.);
#6432=ORIENTED_EDGE('',*,*,#4937,.F.);
#6433=ORIENTED_EDGE('',*,*,#4948,.T.);
#6434=ORIENTED_EDGE('',*,*,#4949,.T.);
#6435=ORIENTED_EDGE('',*,*,#4940,.T.);
#6436=ORIENTED_EDGE('',*,*,#4941,.T.);
#6437=ORIENTED_EDGE('',*,*,#4949,.F.);
#6438=ORIENTED_EDGE('',*,*,#4950,.F.);
#6439=ORIENTED_EDGE('',*,*,#4951,.F.);
#6440=ORIENTED_EDGE('',*,*,#4952,.F.);
#6441=ORIENTED_EDGE('',*,*,#4953,.F.);
#6442=ORIENTED_EDGE('',*,*,#4954,.F.);
#6443=ORIENTED_EDGE('',*,*,#4955,.F.);
#6444=ORIENTED_EDGE('',*,*,#4956,.T.);
#6445=ORIENTED_EDGE('',*,*,#4957,.T.);
#6446=ORIENTED_EDGE('',*,*,#4958,.F.);
#6447=ORIENTED_EDGE('',*,*,#4948,.F.);
#6448=ORIENTED_EDGE('',*,*,#4959,.T.);
#6449=ORIENTED_EDGE('',*,*,#4960,.T.);
#6450=ORIENTED_EDGE('',*,*,#4961,.T.);
#6451=ORIENTED_EDGE('',*,*,#4960,.F.);
#6452=ORIENTED_EDGE('',*,*,#4962,.T.);
#6453=ORIENTED_EDGE('',*,*,#4959,.F.);
#6454=ORIENTED_EDGE('',*,*,#4963,.T.);
#6455=ORIENTED_EDGE('',*,*,#4964,.F.);
#6456=ORIENTED_EDGE('',*,*,#4965,.F.);
#6457=ORIENTED_EDGE('',*,*,#4963,.F.);
#6458=ORIENTED_EDGE('',*,*,#4962,.F.);
#6459=ORIENTED_EDGE('',*,*,#4966,.F.);
#6460=ORIENTED_EDGE('',*,*,#4967,.F.);
#6461=ORIENTED_EDGE('',*,*,#4968,.T.);
#6462=ORIENTED_EDGE('',*,*,#4969,.F.);
#6463=ORIENTED_EDGE('',*,*,#4970,.F.);
#6464=ORIENTED_EDGE('',*,*,#4961,.F.);
#6465=ORIENTED_EDGE('',*,*,#4971,.T.);
#6466=ORIENTED_EDGE('',*,*,#4972,.T.);
#6467=ORIENTED_EDGE('',*,*,#4964,.T.);
#6468=ORIENTED_EDGE('',*,*,#4965,.T.);
#6469=ORIENTED_EDGE('',*,*,#4972,.F.);
#6470=ORIENTED_EDGE('',*,*,#4973,.F.);
#6471=ORIENTED_EDGE('',*,*,#4974,.F.);
#6472=ORIENTED_EDGE('',*,*,#4975,.T.);
#6473=ORIENTED_EDGE('',*,*,#4976,.F.);
#6474=ORIENTED_EDGE('',*,*,#4977,.F.);
#6475=ORIENTED_EDGE('',*,*,#4978,.F.);
#6476=ORIENTED_EDGE('',*,*,#4979,.F.);
#6477=ORIENTED_EDGE('',*,*,#4980,.F.);
#6478=ORIENTED_EDGE('',*,*,#4981,.F.);
#6479=ORIENTED_EDGE('',*,*,#4982,.F.);
#6480=ORIENTED_EDGE('',*,*,#4983,.T.);
#6481=ORIENTED_EDGE('',*,*,#4971,.F.);
#6482=ORIENTED_EDGE('',*,*,#4974,.T.);
#6483=ORIENTED_EDGE('',*,*,#4984,.F.);
#6484=ORIENTED_EDGE('',*,*,#4985,.T.);
#6485=ORIENTED_EDGE('',*,*,#4986,.T.);
#6486=ORIENTED_EDGE('',*,*,#4987,.T.);
#6487=ORIENTED_EDGE('',*,*,#4988,.F.);
#6488=ORIENTED_EDGE('',*,*,#4966,.T.);
#6489=ORIENTED_EDGE('',*,*,#4989,.T.);
#6490=ORIENTED_EDGE('',*,*,#4990,.T.);
#6491=ORIENTED_EDGE('',*,*,#4989,.F.);
#6492=ORIENTED_EDGE('',*,*,#4991,.T.);
#6493=ORIENTED_EDGE('',*,*,#4986,.F.);
#6494=ORIENTED_EDGE('',*,*,#4987,.F.);
#6495=ORIENTED_EDGE('',*,*,#4992,.F.);
#6496=ORIENTED_EDGE('',*,*,#4993,.F.);
#6497=ORIENTED_EDGE('',*,*,#4994,.F.);
#6498=ORIENTED_EDGE('',*,*,#4995,.F.);
#6499=ORIENTED_EDGE('',*,*,#4996,.F.);
#6500=ORIENTED_EDGE('',*,*,#4997,.F.);
#6501=ORIENTED_EDGE('',*,*,#4975,.F.);
#6502=ORIENTED_EDGE('',*,*,#4991,.F.);
#6503=ORIENTED_EDGE('',*,*,#4970,.T.);
#6504=ORIENTED_EDGE('',*,*,#4998,.T.);
#6505=ORIENTED_EDGE('',*,*,#4992,.T.);
#6506=ORIENTED_EDGE('',*,*,#4999,.T.);
#6507=ORIENTED_EDGE('',*,*,#5000,.T.);
#6508=ORIENTED_EDGE('',*,*,#5001,.T.);
#6509=ORIENTED_EDGE('',*,*,#5002,.T.);
#6510=ORIENTED_EDGE('',*,*,#4969,.T.);
#6511=ORIENTED_EDGE('',*,*,#4999,.F.);
#6512=ORIENTED_EDGE('',*,*,#5003,.T.);
#6513=ORIENTED_EDGE('',*,*,#5002,.F.);
#6514=ORIENTED_EDGE('',*,*,#5004,.T.);
#6515=ORIENTED_EDGE('',*,*,#4998,.F.);
#6516=ORIENTED_EDGE('',*,*,#5004,.F.);
#6517=ORIENTED_EDGE('',*,*,#5005,.T.);
#6518=ORIENTED_EDGE('',*,*,#5006,.F.);
#6519=ORIENTED_EDGE('',*,*,#4993,.T.);
#6520=ORIENTED_EDGE('',*,*,#5003,.F.);
#6521=ORIENTED_EDGE('',*,*,#5001,.F.);
#6522=ORIENTED_EDGE('',*,*,#5007,.T.);
#6523=ORIENTED_EDGE('',*,*,#5008,.F.);
#6524=ORIENTED_EDGE('',*,*,#5005,.F.);
#6525=ORIENTED_EDGE('',*,*,#5009,.T.);
#6526=ORIENTED_EDGE('',*,*,#4995,.T.);
#6527=ORIENTED_EDGE('',*,*,#5010,.T.);
#6528=ORIENTED_EDGE('',*,*,#5011,.T.);
#6529=ORIENTED_EDGE('',*,*,#5012,.T.);
#6530=ORIENTED_EDGE('',*,*,#4996,.T.);
#6531=ORIENTED_EDGE('',*,*,#5009,.F.);
#6532=ORIENTED_EDGE('',*,*,#5013,.T.);
#6533=ORIENTED_EDGE('',*,*,#5010,.F.);
#6534=ORIENTED_EDGE('',*,*,#4994,.T.);
#6535=ORIENTED_EDGE('',*,*,#5006,.T.);
#6536=ORIENTED_EDGE('',*,*,#5014,.T.);
#6537=ORIENTED_EDGE('',*,*,#4976,.T.);
#6538=ORIENTED_EDGE('',*,*,#4997,.T.);
#6539=ORIENTED_EDGE('',*,*,#5012,.F.);
#6540=ORIENTED_EDGE('',*,*,#5015,.T.);
#6541=ORIENTED_EDGE('',*,*,#5014,.F.);
#6542=ORIENTED_EDGE('',*,*,#5008,.T.);
#6543=ORIENTED_EDGE('',*,*,#5016,.T.);
#6544=ORIENTED_EDGE('',*,*,#5017,.T.);
#6545=ORIENTED_EDGE('',*,*,#5000,.F.);
#6546=ORIENTED_EDGE('',*,*,#4968,.F.);
#6547=ORIENTED_EDGE('',*,*,#5018,.F.);
#6548=ORIENTED_EDGE('',*,*,#5019,.F.);
#6549=ORIENTED_EDGE('',*,*,#5020,.T.);
#6550=ORIENTED_EDGE('',*,*,#5021,.F.);
#6551=ORIENTED_EDGE('',*,*,#5011,.F.);
#6552=ORIENTED_EDGE('',*,*,#5017,.F.);
#6553=ORIENTED_EDGE('',*,*,#5022,.T.);
#6554=ORIENTED_EDGE('',*,*,#5023,.T.);
#6555=ORIENTED_EDGE('',*,*,#5013,.F.);
#6556=ORIENTED_EDGE('',*,*,#5023,.F.);
#6557=ORIENTED_EDGE('',*,*,#5024,.T.);
#6558=ORIENTED_EDGE('',*,*,#5025,.T.);
#6559=ORIENTED_EDGE('',*,*,#5015,.F.);
#6560=ORIENTED_EDGE('',*,*,#5025,.F.);
#6561=ORIENTED_EDGE('',*,*,#5026,.T.);
#6562=ORIENTED_EDGE('',*,*,#4979,.T.);
#6563=ORIENTED_EDGE('',*,*,#5027,.T.);
#6564=ORIENTED_EDGE('',*,*,#4977,.T.);
#6565=ORIENTED_EDGE('',*,*,#4978,.T.);
#6566=ORIENTED_EDGE('',*,*,#5027,.F.);
#6567=ORIENTED_EDGE('',*,*,#4982,.T.);
#6568=ORIENTED_EDGE('',*,*,#5028,.T.);
#6569=ORIENTED_EDGE('',*,*,#5029,.T.);
#6570=ORIENTED_EDGE('',*,*,#4981,.T.);
#6571=ORIENTED_EDGE('',*,*,#5030,.F.);
#6572=ORIENTED_EDGE('',*,*,#5031,.T.);
#6573=ORIENTED_EDGE('',*,*,#5028,.F.);
#6574=ORIENTED_EDGE('',*,*,#4980,.T.);
#6575=ORIENTED_EDGE('',*,*,#5026,.F.);
#6576=ORIENTED_EDGE('',*,*,#5032,.T.);
#6577=ORIENTED_EDGE('',*,*,#5033,.T.);
#6578=ORIENTED_EDGE('',*,*,#5034,.T.);
#6579=ORIENTED_EDGE('',*,*,#5030,.T.);
#6580=ORIENTED_EDGE('',*,*,#5024,.F.);
#6581=ORIENTED_EDGE('',*,*,#5035,.F.);
#6582=ORIENTED_EDGE('',*,*,#5036,.F.);
#6583=ORIENTED_EDGE('',*,*,#5037,.T.);
#6584=ORIENTED_EDGE('',*,*,#5032,.F.);
#6585=ORIENTED_EDGE('',*,*,#5022,.F.);
#6586=ORIENTED_EDGE('',*,*,#5016,.F.);
#6587=ORIENTED_EDGE('',*,*,#5038,.F.);
#6588=ORIENTED_EDGE('',*,*,#5039,.F.);
#6589=ORIENTED_EDGE('',*,*,#5035,.T.);
#6590=ORIENTED_EDGE('',*,*,#5040,.T.);
#6591=ORIENTED_EDGE('',*,*,#5041,.T.);
#6592=ORIENTED_EDGE('',*,*,#5042,.T.);
#6593=ORIENTED_EDGE('',*,*,#5043,.T.);
#6594=ORIENTED_EDGE('',*,*,#5044,.T.);
#6595=ORIENTED_EDGE('',*,*,#5045,.T.);
#6596=ORIENTED_EDGE('',*,*,#5040,.F.);
#6597=ORIENTED_EDGE('',*,*,#5046,.F.);
#6598=ORIENTED_EDGE('',*,*,#5042,.F.);
#6599=ORIENTED_EDGE('',*,*,#5047,.T.);
#6600=ORIENTED_EDGE('',*,*,#5048,.T.);
#6601=ORIENTED_EDGE('',*,*,#5044,.F.);
#6602=ORIENTED_EDGE('',*,*,#5049,.F.);
#6603=ORIENTED_EDGE('',*,*,#5050,.T.);
#6604=ORIENTED_EDGE('',*,*,#5051,.T.);
#6605=ORIENTED_EDGE('',*,*,#5052,.T.);
#6606=ORIENTED_EDGE('',*,*,#5053,.T.);
#6607=ORIENTED_EDGE('',*,*,#5050,.F.);
#6608=ORIENTED_EDGE('',*,*,#5054,.T.);
#6609=ORIENTED_EDGE('',*,*,#5045,.F.);
#6610=ORIENTED_EDGE('',*,*,#5055,.T.);
#6611=ORIENTED_EDGE('',*,*,#5056,.T.);
#6612=ORIENTED_EDGE('',*,*,#5057,.T.);
#6613=ORIENTED_EDGE('',*,*,#5041,.F.);
#6614=ORIENTED_EDGE('',*,*,#5053,.F.);
#6615=ORIENTED_EDGE('',*,*,#5058,.T.);
#6616=ORIENTED_EDGE('',*,*,#5059,.T.);
#6617=ORIENTED_EDGE('',*,*,#5060,.T.);
#6618=ORIENTED_EDGE('',*,*,#5061,.F.);
#6619=ORIENTED_EDGE('',*,*,#5062,.F.);
#6620=ORIENTED_EDGE('',*,*,#5063,.T.);
#6621=ORIENTED_EDGE('',*,*,#5064,.T.);
#6622=ORIENTED_EDGE('',*,*,#5055,.F.);
#6623=ORIENTED_EDGE('',*,*,#5051,.F.);
#6624=ORIENTED_EDGE('',*,*,#5048,.F.);
#6625=ORIENTED_EDGE('',*,*,#5065,.T.);
#6626=ORIENTED_EDGE('',*,*,#5066,.T.);
#6627=ORIENTED_EDGE('',*,*,#5067,.T.);
#6628=ORIENTED_EDGE('',*,*,#5049,.T.);
#6629=ORIENTED_EDGE('',*,*,#5046,.T.);
#6630=ORIENTED_EDGE('',*,*,#5043,.F.);
#6631=ORIENTED_EDGE('',*,*,#5068,.T.);
#6632=ORIENTED_EDGE('',*,*,#5069,.F.);
#6633=ORIENTED_EDGE('',*,*,#5070,.T.);
#6634=ORIENTED_EDGE('',*,*,#5071,.T.);
#6635=ORIENTED_EDGE('',*,*,#5072,.T.);
#6636=ORIENTED_EDGE('',*,*,#5073,.T.);
#6637=ORIENTED_EDGE('',*,*,#5074,.T.);
#6638=ORIENTED_EDGE('',*,*,#5075,.T.);
#6639=ORIENTED_EDGE('',*,*,#5076,.T.);
#6640=ORIENTED_EDGE('',*,*,#5077,.T.);
#6641=ORIENTED_EDGE('',*,*,#5074,.F.);
#6642=ORIENTED_EDGE('',*,*,#5078,.T.);
#6643=ORIENTED_EDGE('',*,*,#5072,.F.);
#6644=ORIENTED_EDGE('',*,*,#5079,.T.);
#6645=ORIENTED_EDGE('',*,*,#5070,.F.);
#6646=ORIENTED_EDGE('',*,*,#5080,.T.);
#6647=ORIENTED_EDGE('',*,*,#5081,.T.);
#6648=ORIENTED_EDGE('',*,*,#5082,.T.);
#6649=ORIENTED_EDGE('',*,*,#5076,.F.);
#6650=ORIENTED_EDGE('',*,*,#5083,.T.);
#6651=ORIENTED_EDGE('',*,*,#5081,.F.);
#6652=ORIENTED_EDGE('',*,*,#5084,.T.);
#6653=ORIENTED_EDGE('',*,*,#5066,.F.);
#6654=ORIENTED_EDGE('',*,*,#5082,.F.);
#6655=ORIENTED_EDGE('',*,*,#5065,.F.);
#6656=ORIENTED_EDGE('',*,*,#5085,.F.);
#6657=ORIENTED_EDGE('',*,*,#5067,.F.);
#6658=ORIENTED_EDGE('',*,*,#5086,.F.);
#6659=ORIENTED_EDGE('',*,*,#5087,.F.);
#6660=ORIENTED_EDGE('',*,*,#5054,.F.);
#6661=ORIENTED_EDGE('',*,*,#5084,.F.);
#6662=ORIENTED_EDGE('',*,*,#5088,.T.);
#6663=ORIENTED_EDGE('',*,*,#5089,.T.);
#6664=ORIENTED_EDGE('',*,*,#5090,.T.);
#6665=ORIENTED_EDGE('',*,*,#5086,.T.);
#6666=ORIENTED_EDGE('',*,*,#5083,.F.);
#6667=ORIENTED_EDGE('',*,*,#5078,.F.);
#6668=ORIENTED_EDGE('',*,*,#5091,.T.);
#6669=ORIENTED_EDGE('',*,*,#5092,.T.);
#6670=ORIENTED_EDGE('',*,*,#5088,.F.);
#6671=ORIENTED_EDGE('',*,*,#5073,.F.);
#6672=ORIENTED_EDGE('',*,*,#5093,.F.);
#6673=ORIENTED_EDGE('',*,*,#5094,.T.);
#6674=ORIENTED_EDGE('',*,*,#5091,.F.);
#6675=ORIENTED_EDGE('',*,*,#5056,.F.);
#6676=ORIENTED_EDGE('',*,*,#5064,.F.);
#6677=ORIENTED_EDGE('',*,*,#5095,.F.);
#6678=ORIENTED_EDGE('',*,*,#5079,.F.);
#6679=ORIENTED_EDGE('',*,*,#5075,.F.);
#6680=ORIENTED_EDGE('',*,*,#5077,.F.);
#6681=ORIENTED_EDGE('',*,*,#5085,.T.);
#6682=ORIENTED_EDGE('',*,*,#5047,.F.);
#6683=ORIENTED_EDGE('',*,*,#5057,.F.);
#6684=ORIENTED_EDGE('',*,*,#5080,.F.);
#6685=ORIENTED_EDGE('',*,*,#5069,.T.);
#6686=ORIENTED_EDGE('',*,*,#5096,.T.);
#6687=ORIENTED_EDGE('',*,*,#5097,.F.);
#6688=ORIENTED_EDGE('',*,*,#5093,.T.);
#6689=ORIENTED_EDGE('',*,*,#5098,.T.);
#6690=ORIENTED_EDGE('',*,*,#5099,.T.);
#6691=ORIENTED_EDGE('',*,*,#5019,.T.);
#6692=ORIENTED_EDGE('',*,*,#5100,.T.);
#6693=ORIENTED_EDGE('',*,*,#5100,.F.);
#6694=ORIENTED_EDGE('',*,*,#5018,.T.);
#6695=ORIENTED_EDGE('',*,*,#4967,.T.);
#6696=ORIENTED_EDGE('',*,*,#4988,.T.);
#6697=ORIENTED_EDGE('',*,*,#5101,.F.);
#6698=ORIENTED_EDGE('',*,*,#4984,.T.);
#6699=ORIENTED_EDGE('',*,*,#4973,.T.);
#6700=ORIENTED_EDGE('',*,*,#5102,.T.);
#6701=ORIENTED_EDGE('',*,*,#5103,.T.);
#6702=ORIENTED_EDGE('',*,*,#5104,.T.);
#6703=ORIENTED_EDGE('',*,*,#5105,.T.);
#6704=ORIENTED_EDGE('',*,*,#5106,.T.);
#6705=ORIENTED_EDGE('',*,*,#5107,.F.);
#6706=ORIENTED_EDGE('',*,*,#5108,.T.);
#6707=ORIENTED_EDGE('',*,*,#5109,.T.);
#6708=ORIENTED_EDGE('',*,*,#5105,.F.);
#6709=ORIENTED_EDGE('',*,*,#5110,.T.);
#6710=ORIENTED_EDGE('',*,*,#5103,.F.);
#6711=ORIENTED_EDGE('',*,*,#5111,.F.);
#6712=ORIENTED_EDGE('',*,*,#5112,.T.);
#6713=ORIENTED_EDGE('',*,*,#5113,.T.);
#6714=ORIENTED_EDGE('',*,*,#5114,.T.);
#6715=ORIENTED_EDGE('',*,*,#5115,.T.);
#6716=ORIENTED_EDGE('',*,*,#5116,.T.);
#6717=ORIENTED_EDGE('',*,*,#5116,.F.);
#6718=ORIENTED_EDGE('',*,*,#5117,.T.);
#6719=ORIENTED_EDGE('',*,*,#5108,.F.);
#6720=ORIENTED_EDGE('',*,*,#5118,.T.);
#6721=ORIENTED_EDGE('',*,*,#5119,.F.);
#6722=ORIENTED_EDGE('',*,*,#5106,.F.);
#6723=ORIENTED_EDGE('',*,*,#5120,.F.);
#6724=ORIENTED_EDGE('',*,*,#4950,.T.);
#6725=ORIENTED_EDGE('',*,*,#5121,.T.);
#6726=ORIENTED_EDGE('',*,*,#5109,.F.);
#6727=ORIENTED_EDGE('',*,*,#5122,.T.);
#6728=ORIENTED_EDGE('',*,*,#4951,.T.);
#6729=ORIENTED_EDGE('',*,*,#5120,.T.);
#6730=ORIENTED_EDGE('',*,*,#5117,.F.);
#6731=ORIENTED_EDGE('',*,*,#5115,.F.);
#6732=ORIENTED_EDGE('',*,*,#5114,.F.);
#6733=ORIENTED_EDGE('',*,*,#4952,.T.);
#6734=ORIENTED_EDGE('',*,*,#5122,.F.);
#6735=ORIENTED_EDGE('',*,*,#5123,.T.);
#6736=ORIENTED_EDGE('',*,*,#5124,.T.);
#6737=ORIENTED_EDGE('',*,*,#5125,.T.);
#6738=ORIENTED_EDGE('',*,*,#5126,.T.);
#6739=ORIENTED_EDGE('',*,*,#5127,.T.);
#6740=ORIENTED_EDGE('',*,*,#5128,.T.);
#6741=ORIENTED_EDGE('',*,*,#5129,.T.);
#6742=ORIENTED_EDGE('',*,*,#5130,.T.);
#6743=ORIENTED_EDGE('',*,*,#5127,.F.);
#6744=ORIENTED_EDGE('',*,*,#5131,.T.);
#6745=ORIENTED_EDGE('',*,*,#5132,.T.);
#6746=ORIENTED_EDGE('',*,*,#5133,.T.);
#6747=ORIENTED_EDGE('',*,*,#5134,.T.);
#6748=ORIENTED_EDGE('',*,*,#5135,.T.);
#6749=ORIENTED_EDGE('',*,*,#5129,.F.);
#6750=ORIENTED_EDGE('',*,*,#5136,.T.);
#6751=ORIENTED_EDGE('',*,*,#5137,.F.);
#6752=ORIENTED_EDGE('',*,*,#5138,.T.);
#6753=ORIENTED_EDGE('',*,*,#5132,.F.);
#6754=ORIENTED_EDGE('',*,*,#4954,.T.);
#6755=ORIENTED_EDGE('',*,*,#5139,.T.);
#6756=ORIENTED_EDGE('',*,*,#5140,.T.);
#6757=ORIENTED_EDGE('',*,*,#5134,.F.);
#6758=ORIENTED_EDGE('',*,*,#5141,.T.);
#6759=ORIENTED_EDGE('',*,*,#5142,.F.);
#6760=ORIENTED_EDGE('',*,*,#5143,.T.);
#6761=ORIENTED_EDGE('',*,*,#5139,.F.);
#6762=ORIENTED_EDGE('',*,*,#5144,.T.);
#6763=ORIENTED_EDGE('',*,*,#5145,.F.);
#6764=ORIENTED_EDGE('',*,*,#5131,.F.);
#6765=ORIENTED_EDGE('',*,*,#5130,.F.);
#6766=ORIENTED_EDGE('',*,*,#5146,.T.);
#6767=ORIENTED_EDGE('',*,*,#5147,.T.);
#6768=ORIENTED_EDGE('',*,*,#4955,.T.);
#6769=ORIENTED_EDGE('',*,*,#5135,.F.);
#6770=ORIENTED_EDGE('',*,*,#5140,.F.);
#6771=ORIENTED_EDGE('',*,*,#5148,.F.);
#6772=ORIENTED_EDGE('',*,*,#5149,.T.);
#6773=ORIENTED_EDGE('',*,*,#5146,.F.);
#6774=ORIENTED_EDGE('',*,*,#5143,.F.);
#6775=ORIENTED_EDGE('',*,*,#5150,.F.);
#6776=ORIENTED_EDGE('',*,*,#4942,.T.);
#6777=ORIENTED_EDGE('',*,*,#5148,.T.);
#6778=ORIENTED_EDGE('',*,*,#5142,.T.);
#6779=ORIENTED_EDGE('',*,*,#5151,.T.);
#6780=ORIENTED_EDGE('',*,*,#4943,.T.);
#6781=ORIENTED_EDGE('',*,*,#5150,.T.);
#6782=ORIENTED_EDGE('',*,*,#5147,.F.);
#6783=ORIENTED_EDGE('',*,*,#5152,.F.);
#6784=ORIENTED_EDGE('',*,*,#5153,.F.);
#6785=ORIENTED_EDGE('',*,*,#4957,.F.);
#6786=ORIENTED_EDGE('',*,*,#4956,.F.);
#6787=ORIENTED_EDGE('',*,*,#5149,.F.);
#6788=ORIENTED_EDGE('',*,*,#4947,.T.);
#6789=ORIENTED_EDGE('',*,*,#5154,.T.);
#6790=ORIENTED_EDGE('',*,*,#5152,.T.);
#6791=ORIENTED_EDGE('',*,*,#5145,.T.);
#6792=ORIENTED_EDGE('',*,*,#5155,.F.);
#6793=ORIENTED_EDGE('',*,*,#4944,.T.);
#6794=ORIENTED_EDGE('',*,*,#5151,.F.);
#6795=ORIENTED_EDGE('',*,*,#5156,.T.);
#6796=ORIENTED_EDGE('',*,*,#5157,.T.);
#6797=ORIENTED_EDGE('',*,*,#5158,.T.);
#6798=ORIENTED_EDGE('',*,*,#5068,.F.);
#6799=ORIENTED_EDGE('',*,*,#5159,.T.);
#6800=ORIENTED_EDGE('',*,*,#5160,.T.);
#6801=ORIENTED_EDGE('',*,*,#5161,.T.);
#6802=ORIENTED_EDGE('',*,*,#5162,.T.);
#6803=ORIENTED_EDGE('',*,*,#5161,.F.);
#6804=ORIENTED_EDGE('',*,*,#5163,.T.);
#6805=ORIENTED_EDGE('',*,*,#5164,.T.);
#6806=ORIENTED_EDGE('',*,*,#5165,.T.);
#6807=ORIENTED_EDGE('',*,*,#5166,.T.);
#6808=ORIENTED_EDGE('',*,*,#5167,.T.);
#6809=ORIENTED_EDGE('',*,*,#5159,.F.);
#6810=ORIENTED_EDGE('',*,*,#5168,.T.);
#6811=ORIENTED_EDGE('',*,*,#5164,.F.);
#6812=ORIENTED_EDGE('',*,*,#5169,.T.);
#6813=ORIENTED_EDGE('',*,*,#5157,.F.);
#6814=ORIENTED_EDGE('',*,*,#5170,.T.);
#6815=ORIENTED_EDGE('',*,*,#5171,.T.);
#6816=ORIENTED_EDGE('',*,*,#5172,.T.);
#6817=ORIENTED_EDGE('',*,*,#5166,.F.);
#6818=ORIENTED_EDGE('',*,*,#5173,.T.);
#6819=ORIENTED_EDGE('',*,*,#5160,.F.);
#6820=ORIENTED_EDGE('',*,*,#5174,.F.);
#6821=ORIENTED_EDGE('',*,*,#5175,.F.);
#6822=ORIENTED_EDGE('',*,*,#5176,.F.);
#6823=ORIENTED_EDGE('',*,*,#5177,.F.);
#6824=ORIENTED_EDGE('',*,*,#5167,.F.);
#6825=ORIENTED_EDGE('',*,*,#5172,.F.);
#6826=ORIENTED_EDGE('',*,*,#5178,.T.);
#6827=ORIENTED_EDGE('',*,*,#5174,.T.);
#6828=ORIENTED_EDGE('',*,*,#5171,.F.);
#6829=ORIENTED_EDGE('',*,*,#5179,.T.);
#6830=ORIENTED_EDGE('',*,*,#5180,.T.);
#6831=ORIENTED_EDGE('',*,*,#5181,.T.);
#6832=ORIENTED_EDGE('',*,*,#5173,.F.);
#6833=ORIENTED_EDGE('',*,*,#5182,.F.);
#6834=ORIENTED_EDGE('',*,*,#5183,.F.);
#6835=ORIENTED_EDGE('',*,*,#5179,.F.);
#6836=ORIENTED_EDGE('',*,*,#5168,.F.);
#6837=ORIENTED_EDGE('',*,*,#5162,.F.);
#6838=ORIENTED_EDGE('',*,*,#5165,.F.);
#6839=ORIENTED_EDGE('',*,*,#5184,.F.);
#6840=ORIENTED_EDGE('',*,*,#5185,.F.);
#6841=ORIENTED_EDGE('',*,*,#5186,.F.);
#6842=ORIENTED_EDGE('',*,*,#5187,.F.);
#6843=ORIENTED_EDGE('',*,*,#5182,.T.);
#6844=ORIENTED_EDGE('',*,*,#5141,.F.);
#6845=ORIENTED_EDGE('',*,*,#5188,.T.);
#6846=ORIENTED_EDGE('',*,*,#5189,.T.);
#6847=ORIENTED_EDGE('',*,*,#5190,.T.);
#6848=ORIENTED_EDGE('',*,*,#5155,.T.);
#6849=ORIENTED_EDGE('',*,*,#5144,.F.);
#6850=ORIENTED_EDGE('',*,*,#5191,.T.);
#6851=ORIENTED_EDGE('',*,*,#5192,.T.);
#6852=ORIENTED_EDGE('',*,*,#5193,.T.);
#6853=ORIENTED_EDGE('',*,*,#5036,.T.);
#6854=ORIENTED_EDGE('',*,*,#5193,.F.);
#6855=ORIENTED_EDGE('',*,*,#5194,.T.);
#6856=ORIENTED_EDGE('',*,*,#5189,.F.);
#6857=ORIENTED_EDGE('',*,*,#5195,.T.);
#6858=ORIENTED_EDGE('',*,*,#5007,.F.);
#6859=ORIENTED_EDGE('',*,*,#5021,.T.);
#6860=ORIENTED_EDGE('',*,*,#5196,.T.);
#6861=ORIENTED_EDGE('',*,*,#5038,.T.);
#6862=ORIENTED_EDGE('',*,*,#5196,.F.);
#6863=ORIENTED_EDGE('',*,*,#5197,.T.);
#6864=ORIENTED_EDGE('',*,*,#5191,.F.);
#6865=ORIENTED_EDGE('',*,*,#5039,.T.);
#6866=ORIENTED_EDGE('',*,*,#5190,.F.);
#6867=ORIENTED_EDGE('',*,*,#5198,.F.);
#6868=ORIENTED_EDGE('',*,*,#5199,.F.);
#6869=ORIENTED_EDGE('',*,*,#4945,.T.);
#6870=ORIENTED_EDGE('',*,*,#5071,.F.);
#6871=ORIENTED_EDGE('',*,*,#5095,.T.);
#6872=ORIENTED_EDGE('',*,*,#5063,.F.);
#6873=ORIENTED_EDGE('',*,*,#5200,.F.);
#6874=ORIENTED_EDGE('',*,*,#5201,.F.);
#6875=ORIENTED_EDGE('',*,*,#5202,.F.);
#6876=ORIENTED_EDGE('',*,*,#5203,.F.);
#6877=ORIENTED_EDGE('',*,*,#5204,.F.);
#6878=ORIENTED_EDGE('',*,*,#5198,.T.);
#6879=ORIENTED_EDGE('',*,*,#5194,.F.);
#6880=ORIENTED_EDGE('',*,*,#5192,.F.);
#6881=ORIENTED_EDGE('',*,*,#5197,.F.);
#6882=ORIENTED_EDGE('',*,*,#5020,.F.);
#6883=ORIENTED_EDGE('',*,*,#5205,.F.);
#6884=ORIENTED_EDGE('',*,*,#5206,.F.);
#6885=ORIENTED_EDGE('',*,*,#5207,.T.);
#6886=ORIENTED_EDGE('',*,*,#5184,.T.);
#6887=ORIENTED_EDGE('',*,*,#5170,.F.);
#6888=ORIENTED_EDGE('',*,*,#5156,.F.);
#6889=ORIENTED_EDGE('',*,*,#5208,.F.);
#6890=ORIENTED_EDGE('',*,*,#5209,.F.);
#6891=ORIENTED_EDGE('',*,*,#5210,.F.);
#6892=ORIENTED_EDGE('',*,*,#5211,.F.);
#6893=ORIENTED_EDGE('',*,*,#5062,.T.);
#6894=ORIENTED_EDGE('',*,*,#5212,.T.);
#6895=ORIENTED_EDGE('',*,*,#5213,.T.);
#6896=ORIENTED_EDGE('',*,*,#5200,.T.);
#6897=ORIENTED_EDGE('',*,*,#5214,.T.);
#6898=ORIENTED_EDGE('',*,*,#5215,.T.);
#6899=ORIENTED_EDGE('',*,*,#5216,.T.);
#6900=ORIENTED_EDGE('',*,*,#5217,.T.);
#6901=ORIENTED_EDGE('',*,*,#5060,.F.);
#6902=ORIENTED_EDGE('',*,*,#5218,.T.);
#6903=ORIENTED_EDGE('',*,*,#5219,.T.);
#6904=ORIENTED_EDGE('',*,*,#5220,.T.);
#6905=ORIENTED_EDGE('',*,*,#5219,.F.);
#6906=ORIENTED_EDGE('',*,*,#5221,.T.);
#6907=ORIENTED_EDGE('',*,*,#5216,.F.);
#6908=ORIENTED_EDGE('',*,*,#5214,.F.);
#6909=ORIENTED_EDGE('',*,*,#5222,.T.);
#6910=ORIENTED_EDGE('',*,*,#5213,.F.);
#6911=ORIENTED_EDGE('',*,*,#5222,.F.);
#6912=ORIENTED_EDGE('',*,*,#5223,.T.);
#6913=ORIENTED_EDGE('',*,*,#5224,.T.);
#6914=ORIENTED_EDGE('',*,*,#5201,.T.);
#6915=ORIENTED_EDGE('',*,*,#5217,.F.);
#6916=ORIENTED_EDGE('',*,*,#5225,.F.);
#6917=ORIENTED_EDGE('',*,*,#5226,.T.);
#6918=ORIENTED_EDGE('',*,*,#5227,.F.);
#6919=ORIENTED_EDGE('',*,*,#5223,.F.);
#6920=ORIENTED_EDGE('',*,*,#5221,.F.);
#6921=ORIENTED_EDGE('',*,*,#5228,.T.);
#6922=ORIENTED_EDGE('',*,*,#5125,.F.);
#6923=ORIENTED_EDGE('',*,*,#5229,.T.);
#6924=ORIENTED_EDGE('',*,*,#5225,.T.);
#6925=ORIENTED_EDGE('',*,*,#5230,.T.);
#6926=ORIENTED_EDGE('',*,*,#5231,.T.);
#6927=ORIENTED_EDGE('',*,*,#5232,.T.);
#6928=ORIENTED_EDGE('',*,*,#5233,.T.);
#6929=ORIENTED_EDGE('',*,*,#5234,.F.);
#6930=ORIENTED_EDGE('',*,*,#5235,.T.);
#6931=ORIENTED_EDGE('',*,*,#5236,.T.);
#6932=ORIENTED_EDGE('',*,*,#5237,.F.);
#6933=ORIENTED_EDGE('',*,*,#5238,.T.);
#6934=ORIENTED_EDGE('',*,*,#5239,.T.);
#6935=ORIENTED_EDGE('',*,*,#5031,.F.);
#6936=ORIENTED_EDGE('',*,*,#5034,.F.);
#6937=ORIENTED_EDGE('',*,*,#5240,.F.);
#6938=ORIENTED_EDGE('',*,*,#5241,.T.);
#6939=ORIENTED_EDGE('',*,*,#5118,.F.);
#6940=ORIENTED_EDGE('',*,*,#5110,.F.);
#6941=ORIENTED_EDGE('',*,*,#5104,.F.);
#6942=ORIENTED_EDGE('',*,*,#5112,.F.);
#6943=ORIENTED_EDGE('',*,*,#5126,.F.);
#6944=ORIENTED_EDGE('',*,*,#5228,.F.);
#6945=ORIENTED_EDGE('',*,*,#5218,.F.);
#6946=ORIENTED_EDGE('',*,*,#5059,.F.);
#6947=ORIENTED_EDGE('',*,*,#5242,.T.);
#6948=ORIENTED_EDGE('',*,*,#5243,.T.);
#6949=ORIENTED_EDGE('',*,*,#5244,.T.);
#6950=ORIENTED_EDGE('',*,*,#5176,.T.);
#6951=ORIENTED_EDGE('',*,*,#5245,.T.);
#6952=ORIENTED_EDGE('',*,*,#5246,.T.);
#6953=ORIENTED_EDGE('',*,*,#5247,.T.);
#6954=ORIENTED_EDGE('',*,*,#5248,.T.);
#6955=ORIENTED_EDGE('',*,*,#5249,.T.);
#6956=ORIENTED_EDGE('',*,*,#5250,.T.);
#6957=ORIENTED_EDGE('',*,*,#5202,.T.);
#6958=ORIENTED_EDGE('',*,*,#5224,.F.);
#6959=ORIENTED_EDGE('',*,*,#5251,.T.);
#6960=ORIENTED_EDGE('',*,*,#5252,.T.);
#6961=ORIENTED_EDGE('',*,*,#5203,.T.);
#6962=ORIENTED_EDGE('',*,*,#5250,.F.);
#6963=ORIENTED_EDGE('',*,*,#5253,.T.);
#6964=ORIENTED_EDGE('',*,*,#5254,.T.);
#6965=ORIENTED_EDGE('',*,*,#5255,.T.);
#6966=ORIENTED_EDGE('',*,*,#5256,.T.);
#6967=ORIENTED_EDGE('',*,*,#5199,.T.);
#6968=ORIENTED_EDGE('',*,*,#5254,.F.);
#6969=ORIENTED_EDGE('',*,*,#5204,.T.);
#6970=ORIENTED_EDGE('',*,*,#5252,.F.);
#6971=ORIENTED_EDGE('',*,*,#5257,.T.);
#6972=ORIENTED_EDGE('',*,*,#5258,.T.);
#6973=ORIENTED_EDGE('',*,*,#4946,.T.);
#6974=ORIENTED_EDGE('',*,*,#5256,.F.);
#6975=ORIENTED_EDGE('',*,*,#5259,.T.);
#6976=ORIENTED_EDGE('',*,*,#5258,.F.);
#6977=ORIENTED_EDGE('',*,*,#5260,.T.);
#6978=ORIENTED_EDGE('',*,*,#5154,.F.);
#6979=ORIENTED_EDGE('',*,*,#5253,.F.);
#6980=ORIENTED_EDGE('',*,*,#5261,.F.);
#6981=ORIENTED_EDGE('',*,*,#5262,.F.);
#6982=ORIENTED_EDGE('',*,*,#5251,.F.);
#6983=ORIENTED_EDGE('',*,*,#5227,.T.);
#6984=ORIENTED_EDGE('',*,*,#5263,.T.);
#6985=ORIENTED_EDGE('',*,*,#5261,.T.);
#6986=ORIENTED_EDGE('',*,*,#5212,.F.);
#6987=ORIENTED_EDGE('',*,*,#5061,.T.);
#6988=ORIENTED_EDGE('',*,*,#5220,.F.);
#6989=ORIENTED_EDGE('',*,*,#5215,.F.);
#6990=ORIENTED_EDGE('',*,*,#5260,.F.);
#6991=ORIENTED_EDGE('',*,*,#5264,.T.);
#6992=ORIENTED_EDGE('',*,*,#5265,.F.);
#6993=ORIENTED_EDGE('',*,*,#5121,.F.);
#6994=ORIENTED_EDGE('',*,*,#4958,.T.);
#6995=ORIENTED_EDGE('',*,*,#5153,.T.);
#6996=ORIENTED_EDGE('',*,*,#5257,.F.);
#6997=ORIENTED_EDGE('',*,*,#5262,.T.);
#6998=ORIENTED_EDGE('',*,*,#5263,.F.);
#6999=ORIENTED_EDGE('',*,*,#5226,.F.);
#7000=ORIENTED_EDGE('',*,*,#5229,.F.);
#7001=ORIENTED_EDGE('',*,*,#5124,.F.);
#7002=ORIENTED_EDGE('',*,*,#5123,.F.);
#7003=ORIENTED_EDGE('',*,*,#5111,.T.);
#7004=ORIENTED_EDGE('',*,*,#5107,.T.);
#7005=ORIENTED_EDGE('',*,*,#5119,.T.);
#7006=ORIENTED_EDGE('',*,*,#5265,.T.);
#7007=ORIENTED_EDGE('',*,*,#5264,.F.);
#7008=ORIENTED_EDGE('',*,*,#5259,.F.);
#7009=ORIENTED_EDGE('',*,*,#5255,.F.);
#7010=ORIENTED_EDGE('',*,*,#5138,.F.);
#7011=ORIENTED_EDGE('',*,*,#5266,.T.);
#7012=ORIENTED_EDGE('',*,*,#5267,.T.);
#7013=ORIENTED_EDGE('',*,*,#5268,.T.);
#7014=ORIENTED_EDGE('',*,*,#5133,.F.);
#7015=ORIENTED_EDGE('',*,*,#5267,.F.);
#7016=ORIENTED_EDGE('',*,*,#5240,.T.);
#7017=ORIENTED_EDGE('',*,*,#5033,.F.);
#7018=ORIENTED_EDGE('',*,*,#5269,.T.);
#7019=ORIENTED_EDGE('',*,*,#5029,.F.);
#7020=ORIENTED_EDGE('',*,*,#5239,.F.);
#7021=ORIENTED_EDGE('',*,*,#5098,.F.);
#7022=ORIENTED_EDGE('',*,*,#5102,.F.);
#7023=ORIENTED_EDGE('',*,*,#4983,.F.);
#7024=ORIENTED_EDGE('',*,*,#5113,.F.);
#7025=ORIENTED_EDGE('',*,*,#5241,.F.);
#7026=ORIENTED_EDGE('',*,*,#5266,.F.);
#7027=ORIENTED_EDGE('',*,*,#5137,.T.);
#7028=ORIENTED_EDGE('',*,*,#4953,.T.);
#7029=ORIENTED_EDGE('',*,*,#5270,.T.);
#7030=ORIENTED_EDGE('',*,*,#5271,.T.);
#7031=ORIENTED_EDGE('',*,*,#5272,.T.);
#7032=ORIENTED_EDGE('',*,*,#5273,.T.);
#7033=ORIENTED_EDGE('',*,*,#5206,.T.);
#7034=ORIENTED_EDGE('',*,*,#5274,.T.);
#7035=ORIENTED_EDGE('',*,*,#5237,.T.);
#7036=ORIENTED_EDGE('',*,*,#5275,.T.);
#7037=ORIENTED_EDGE('',*,*,#5270,.F.);
#7038=ORIENTED_EDGE('',*,*,#5276,.T.);
#7039=ORIENTED_EDGE('',*,*,#5235,.F.);
#7040=ORIENTED_EDGE('',*,*,#5277,.T.);
#7041=ORIENTED_EDGE('',*,*,#5278,.F.);
#7042=ORIENTED_EDGE('',*,*,#5273,.F.);
#7043=ORIENTED_EDGE('',*,*,#5279,.F.);
#7044=ORIENTED_EDGE('',*,*,#5207,.F.);
#7045=ORIENTED_EDGE('',*,*,#5275,.F.);
#7046=ORIENTED_EDGE('',*,*,#5236,.F.);
#7047=ORIENTED_EDGE('',*,*,#5276,.F.);
#7048=ORIENTED_EDGE('',*,*,#5099,.F.);
#7049=ORIENTED_EDGE('',*,*,#5238,.F.);
#7050=ORIENTED_EDGE('',*,*,#5274,.F.);
#7051=ORIENTED_EDGE('',*,*,#5205,.T.);
#7052=ORIENTED_EDGE('',*,*,#5271,.F.);
#7053=ORIENTED_EDGE('',*,*,#5278,.T.);
#7054=ORIENTED_EDGE('',*,*,#5280,.T.);
#7055=ORIENTED_EDGE('',*,*,#5281,.T.);
#7056=ORIENTED_EDGE('',*,*,#5272,.F.);
#7057=ORIENTED_EDGE('',*,*,#5281,.F.);
#7058=ORIENTED_EDGE('',*,*,#5282,.T.);
#7059=ORIENTED_EDGE('',*,*,#5185,.T.);
#7060=ORIENTED_EDGE('',*,*,#5279,.T.);
#7061=ORIENTED_EDGE('',*,*,#5277,.F.);
#7062=ORIENTED_EDGE('',*,*,#5234,.T.);
#7063=ORIENTED_EDGE('',*,*,#5283,.T.);
#7064=ORIENTED_EDGE('',*,*,#5284,.F.);
#7065=ORIENTED_EDGE('',*,*,#5285,.T.);
#7066=ORIENTED_EDGE('',*,*,#5284,.T.);
#7067=ORIENTED_EDGE('',*,*,#5286,.T.);
#7068=ORIENTED_EDGE('',*,*,#5287,.T.);
#7069=ORIENTED_EDGE('',*,*,#5288,.T.);
#7070=ORIENTED_EDGE('',*,*,#5231,.F.);
#7071=ORIENTED_EDGE('',*,*,#5289,.T.);
#7072=ORIENTED_EDGE('',*,*,#5290,.T.);
#7073=ORIENTED_EDGE('',*,*,#5291,.T.);
#7074=ORIENTED_EDGE('',*,*,#5292,.T.);
#7075=ORIENTED_EDGE('',*,*,#5293,.T.);
#7076=ORIENTED_EDGE('',*,*,#5232,.F.);
#7077=ORIENTED_EDGE('',*,*,#5293,.F.);
#7078=ORIENTED_EDGE('',*,*,#5294,.T.);
#7079=ORIENTED_EDGE('',*,*,#5291,.F.);
#7080=ORIENTED_EDGE('',*,*,#5295,.T.);
#7081=ORIENTED_EDGE('',*,*,#5296,.T.);
#7082=ORIENTED_EDGE('',*,*,#5296,.F.);
#7083=ORIENTED_EDGE('',*,*,#5297,.T.);
#7084=ORIENTED_EDGE('',*,*,#5287,.F.);
#7085=ORIENTED_EDGE('',*,*,#5298,.T.);
#7086=ORIENTED_EDGE('',*,*,#5295,.F.);
#7087=ORIENTED_EDGE('',*,*,#5299,.T.);
#7088=ORIENTED_EDGE('',*,*,#5300,.F.);
#7089=ORIENTED_EDGE('',*,*,#5301,.T.);
#7090=ORIENTED_EDGE('',*,*,#5290,.F.);
#7091=ORIENTED_EDGE('',*,*,#5289,.F.);
#7092=ORIENTED_EDGE('',*,*,#5230,.F.);
#7093=ORIENTED_EDGE('',*,*,#5302,.F.);
#7094=ORIENTED_EDGE('',*,*,#5181,.F.);
#7095=ORIENTED_EDGE('',*,*,#5299,.F.);
#7096=ORIENTED_EDGE('',*,*,#5245,.F.);
#7097=ORIENTED_EDGE('',*,*,#5175,.T.);
#7098=ORIENTED_EDGE('',*,*,#5178,.F.);
#7099=ORIENTED_EDGE('',*,*,#5302,.T.);
#7100=ORIENTED_EDGE('',*,*,#5163,.F.);
#7101=ORIENTED_EDGE('',*,*,#5177,.T.);
#7102=ORIENTED_EDGE('',*,*,#5244,.F.);
#7103=ORIENTED_EDGE('',*,*,#5303,.T.);
#7104=ORIENTED_EDGE('',*,*,#5169,.F.);
#7105=ORIENTED_EDGE('',*,*,#5282,.F.);
#7106=ORIENTED_EDGE('',*,*,#5304,.T.);
#7107=ORIENTED_EDGE('',*,*,#5305,.T.);
#7108=ORIENTED_EDGE('',*,*,#5186,.T.);
#7109=ORIENTED_EDGE('',*,*,#5306,.T.);
#7110=ORIENTED_EDGE('',*,*,#5187,.T.);
#7111=ORIENTED_EDGE('',*,*,#5305,.F.);
#7112=ORIENTED_EDGE('',*,*,#5307,.T.);
#7113=ORIENTED_EDGE('',*,*,#5308,.T.);
#7114=ORIENTED_EDGE('',*,*,#5183,.T.);
#7115=ORIENTED_EDGE('',*,*,#5306,.F.);
#7116=ORIENTED_EDGE('',*,*,#5309,.T.);
#7117=ORIENTED_EDGE('',*,*,#5308,.F.);
#7118=ORIENTED_EDGE('',*,*,#5300,.T.);
#7119=ORIENTED_EDGE('',*,*,#5180,.F.);
#7120=ORIENTED_EDGE('',*,*,#5297,.F.);
#7121=ORIENTED_EDGE('',*,*,#5301,.F.);
#7122=ORIENTED_EDGE('',*,*,#5309,.F.);
#7123=ORIENTED_EDGE('',*,*,#5307,.F.);
#7124=ORIENTED_EDGE('',*,*,#5310,.T.);
#7125=ORIENTED_EDGE('',*,*,#5288,.F.);
#7126=ORIENTED_EDGE('',*,*,#5280,.F.);
#7127=ORIENTED_EDGE('',*,*,#5285,.F.);
#7128=ORIENTED_EDGE('',*,*,#5310,.F.);
#7129=ORIENTED_EDGE('',*,*,#5304,.F.);
#7130=ORIENTED_EDGE('',*,*,#5283,.F.);
#7131=ORIENTED_EDGE('',*,*,#5233,.F.);
#7132=ORIENTED_EDGE('',*,*,#5294,.F.);
#7133=ORIENTED_EDGE('',*,*,#5311,.F.);
#7134=ORIENTED_EDGE('',*,*,#5286,.F.);
#7135=ORIENTED_EDGE('',*,*,#5096,.F.);
#7136=ORIENTED_EDGE('',*,*,#5158,.F.);
#7137=ORIENTED_EDGE('',*,*,#5303,.F.);
#7138=ORIENTED_EDGE('',*,*,#5243,.F.);
#7139=ORIENTED_EDGE('',*,*,#5089,.F.);
#7140=ORIENTED_EDGE('',*,*,#5092,.F.);
#7141=ORIENTED_EDGE('',*,*,#5094,.F.);
#7142=ORIENTED_EDGE('',*,*,#5097,.T.);
#7143=ORIENTED_EDGE('',*,*,#5242,.F.);
#7144=ORIENTED_EDGE('',*,*,#5058,.F.);
#7145=ORIENTED_EDGE('',*,*,#5052,.F.);
#7146=ORIENTED_EDGE('',*,*,#5312,.F.);
#7147=ORIENTED_EDGE('',*,*,#5128,.F.);
#7148=ORIENTED_EDGE('',*,*,#5268,.F.);
#7149=ORIENTED_EDGE('',*,*,#5269,.F.);
#7150=ORIENTED_EDGE('',*,*,#5037,.F.);
#7151=ORIENTED_EDGE('',*,*,#5195,.F.);
#7152=ORIENTED_EDGE('',*,*,#5188,.F.);
#7153=ORIENTED_EDGE('',*,*,#5136,.F.);
#7154=ORIENTED_EDGE('',*,*,#5211,.T.);
#7155=ORIENTED_EDGE('',*,*,#5313,.T.);
#7156=ORIENTED_EDGE('',*,*,#5246,.F.);
#7157=ORIENTED_EDGE('',*,*,#5313,.F.);
#7158=ORIENTED_EDGE('',*,*,#5210,.T.);
#7159=ORIENTED_EDGE('',*,*,#5314,.T.);
#7160=ORIENTED_EDGE('',*,*,#5247,.F.);
#7161=ORIENTED_EDGE('',*,*,#5314,.F.);
#7162=ORIENTED_EDGE('',*,*,#5209,.T.);
#7163=ORIENTED_EDGE('',*,*,#5315,.T.);
#7164=ORIENTED_EDGE('',*,*,#5248,.F.);
#7165=ORIENTED_EDGE('',*,*,#5315,.F.);
#7166=ORIENTED_EDGE('',*,*,#5208,.T.);
#7167=ORIENTED_EDGE('',*,*,#5316,.T.);
#7168=ORIENTED_EDGE('',*,*,#5249,.F.);
#7169=ORIENTED_EDGE('',*,*,#5316,.F.);
#7170=ORIENTED_EDGE('',*,*,#5090,.F.);
#7171=ORIENTED_EDGE('',*,*,#5312,.T.);
#7172=ORIENTED_EDGE('',*,*,#5087,.T.);
#7173=ORIENTED_EDGE('',*,*,#4985,.F.);
#7174=ORIENTED_EDGE('',*,*,#5101,.T.);
#7175=ORIENTED_EDGE('',*,*,#4990,.F.);
#7176=ORIENTED_EDGE('',*,*,#5298,.F.);
#7177=ORIENTED_EDGE('',*,*,#5311,.T.);
#7178=ORIENTED_EDGE('',*,*,#5292,.F.);
#9375=TOROIDAL_SURFACE('',#10100,1.45,0.1);
#9376=TOROIDAL_SURFACE('',#10110,1.45,0.1);
#9377=TOROIDAL_SURFACE('',#10114,1.45,0.1);
#9378=TOROIDAL_SURFACE('',#10123,1.45,0.1);
#9380=ADVANCED_FACE('',(#2402),#9375,.T.);
#9381=ADVANCED_FACE('',(#2403),#2271,.F.);
#9382=ADVANCED_FACE('',(#2404,#386),#995,.F.);
#9383=ADVANCED_FACE('',(#2405),#9376,.T.);
#9384=ADVANCED_FACE('',(#2406,#387),#996,.T.);
#9385=ADVANCED_FACE('',(#2407),#9377,.T.);
#9386=ADVANCED_FACE('',(#2408),#2272,.F.);
#9387=ADVANCED_FACE('',(#2409,#388),#997,.F.);
#9388=ADVANCED_FACE('',(#2410),#9378,.T.);
#9389=ADVANCED_FACE('',(#2411,#389),#998,.T.);
#9390=ADVANCED_FACE('',(#2412),#280,.F.);
#9391=ADVANCED_FACE('',(#2413),#2273,.T.);
#9392=ADVANCED_FACE('',(#2414),#270,.T.);
#9393=ADVANCED_FACE('',(#2415),#281,.T.);
#9394=ADVANCED_FACE('',(#2416),#282,.F.);
#9395=ADVANCED_FACE('',(#2417),#283,.F.);
#9396=ADVANCED_FACE('',(#2418),#284,.F.);
#9397=ADVANCED_FACE('',(#2419),#271,.T.);
#9398=ADVANCED_FACE('',(#2420),#285,.F.);
#9399=ADVANCED_FACE('',(#2421),#286,.T.);
#9400=ADVANCED_FACE('',(#2422),#287,.F.);
#9401=ADVANCED_FACE('',(#2423),#288,.F.);
#9402=ADVANCED_FACE('',(#2424),#289,.F.);
#9403=ADVANCED_FACE('',(#2425),#290,.F.);
#9404=ADVANCED_FACE('',(#2426),#291,.T.);
#9405=ADVANCED_FACE('',(#2427),#2274,.T.);
#9406=ADVANCED_FACE('',(#2428),#292,.T.);
#9407=ADVANCED_FACE('',(#2429),#293,.T.);
#9408=ADVANCED_FACE('',(#2430),#294,.T.);
#9409=ADVANCED_FACE('',(#2431),#295,.T.);
#9410=ADVANCED_FACE('',(#2432),#296,.F.);
#9411=ADVANCED_FACE('',(#2433),#297,.F.);
#9412=ADVANCED_FACE('',(#2434),#298,.F.);
#9413=ADVANCED_FACE('',(#2435),#299,.T.);
#9414=ADVANCED_FACE('',(#2436),#300,.T.);
#9415=ADVANCED_FACE('',(#2437),#301,.T.);
#9416=ADVANCED_FACE('',(#2438),#302,.T.);
#9417=ADVANCED_FACE('',(#2439),#303,.T.);
#9418=ADVANCED_FACE('',(#2440),#304,.T.);
#9419=ADVANCED_FACE('',(#2441),#305,.T.);
#9420=ADVANCED_FACE('',(#2442),#306,.F.);
#9421=ADVANCED_FACE('',(#2443),#307,.T.);
#9422=ADVANCED_FACE('',(#2444),#308,.F.);
#9423=ADVANCED_FACE('',(#2445),#309,.F.);
#9424=ADVANCED_FACE('',(#2446),#310,.F.);
#9425=ADVANCED_FACE('',(#2447),#311,.F.);
#9426=ADVANCED_FACE('',(#2448),#312,.F.);
#9427=ADVANCED_FACE('',(#2449),#313,.F.);
#9428=ADVANCED_FACE('',(#2450),#272,.T.);
#9429=ADVANCED_FACE('',(#2451),#999,.F.);
#9430=ADVANCED_FACE('',(#2452),#314,.T.);
#9431=ADVANCED_FACE('',(#2453),#315,.F.);
#9432=ADVANCED_FACE('',(#2454),#316,.T.);
#9433=ADVANCED_FACE('',(#2455),#317,.T.);
#9434=ADVANCED_FACE('',(#2456),#2275,.T.);
#9435=ADVANCED_FACE('',(#2457),#318,.T.);
#9436=ADVANCED_FACE('',(#2458),#2276,.F.);
#9437=ADVANCED_FACE('',(#2459),#319,.T.);
#9438=ADVANCED_FACE('',(#2460),#320,.F.);
#9439=ADVANCED_FACE('',(#2461),#321,.F.);
#9440=ADVANCED_FACE('',(#2462),#322,.F.);
#9441=ADVANCED_FACE('',(#2463),#323,.F.);
#9442=ADVANCED_FACE('',(#2464),#324,.F.);
#9443=ADVANCED_FACE('',(#2465),#325,.T.);
#9444=ADVANCED_FACE('',(#2466),#326,.T.);
#9445=ADVANCED_FACE('',(#2467),#327,.T.);
#9446=ADVANCED_FACE('',(#2468),#328,.T.);
#9447=ADVANCED_FACE('',(#2469),#329,.T.);
#9448=ADVANCED_FACE('',(#2470),#330,.T.);
#9449=ADVANCED_FACE('',(#2471),#331,.T.);
#9450=ADVANCED_FACE('',(#2472),#332,.T.);
#9451=ADVANCED_FACE('',(#2473),#333,.T.);
#9452=ADVANCED_FACE('',(#2474),#334,.T.);
#9453=ADVANCED_FACE('',(#2475),#335,.F.);
#9454=ADVANCED_FACE('',(#2476),#273,.T.);
#9455=ADVANCED_FACE('',(#2477),#2277,.T.);
#9456=ADVANCED_FACE('',(#2478),#336,.T.);
#9457=ADVANCED_FACE('',(#2479),#337,.T.);
#9458=ADVANCED_FACE('',(#2480),#338,.F.);
#9459=ADVANCED_FACE('',(#2481),#1000,.T.);
#9460=ADVANCED_FACE('',(#2482),#2278,.T.);
#9461=ADVANCED_FACE('',(#2483),#339,.F.);
#9462=ADVANCED_FACE('',(#2484),#340,.F.);
#9463=ADVANCED_FACE('',(#2485),#341,.F.);
#9464=ADVANCED_FACE('',(#2486),#342,.F.);
#9465=ADVANCED_FACE('',(#2487),#343,.F.);
#9466=ADVANCED_FACE('',(#2488),#344,.T.);
#9467=ADVANCED_FACE('',(#2489),#345,.T.);
#9468=ADVANCED_FACE('',(#2490),#346,.F.);
#9469=ADVANCED_FACE('',(#2491),#1001,.F.);
#9470=ADVANCED_FACE('',(#2492),#2279,.T.);
#9471=ADVANCED_FACE('',(#2493),#347,.F.);
#9472=ADVANCED_FACE('',(#2494),#348,.F.);
#9473=ADVANCED_FACE('',(#2495),#349,.F.);
#9474=ADVANCED_FACE('',(#2496),#350,.F.);
#9475=ADVANCED_FACE('',(#2497),#351,.F.);
#9476=ADVANCED_FACE('',(#2498),#2280,.T.);
#9477=ADVANCED_FACE('',(#2499,#390,#391,#392,#393),#1002,.F.);
#9478=ADVANCED_FACE('',(#2500),#2281,.T.);
#9479=ADVANCED_FACE('',(#2501),#2282,.T.);
#9480=ADVANCED_FACE('',(#2502),#2283,.T.);
#9481=ADVANCED_FACE('',(#2503),#274,.T.);
#9482=ADVANCED_FACE('',(#2504),#275,.T.);
#9483=ADVANCED_FACE('',(#2505),#2284,.T.);
#9484=ADVANCED_FACE('',(#2506),#1003,.T.);
#9485=ADVANCED_FACE('',(#2507),#2285,.T.);
#9486=ADVANCED_FACE('',(#2508,#394,#395,#396,#397),#1004,.T.);
#9487=ADVANCED_FACE('',(#2509),#352,.F.);
#9488=ADVANCED_FACE('',(#2510),#353,.F.);
#9489=ADVANCED_FACE('',(#2511),#354,.F.);
#9490=ADVANCED_FACE('',(#2512),#355,.F.);
#9491=ADVANCED_FACE('',(#2513),#356,.F.);
#9492=ADVANCED_FACE('',(#2514),#276,.T.);
#9493=ADVANCED_FACE('',(#2515),#357,.T.);
#9494=ADVANCED_FACE('',(#2516),#2286,.F.);
#9495=ADVANCED_FACE('',(#2517),#1005,.T.);
#9496=ADVANCED_FACE('',(#2518),#358,.F.);
#9497=ADVANCED_FACE('',(#2519),#359,.T.);
#9498=ADVANCED_FACE('',(#2520),#360,.F.);
#9499=ADVANCED_FACE('',(#2521),#361,.F.);
#9500=ADVANCED_FACE('',(#2522),#2287,.F.);
#9501=ADVANCED_FACE('',(#2523),#2288,.F.);
#9502=ADVANCED_FACE('',(#2524),#362,.F.);
#9503=ADVANCED_FACE('',(#2525),#363,.T.);
#9504=ADVANCED_FACE('',(#2526),#1006,.T.);
#9505=ADVANCED_FACE('',(#2527),#1007,.T.);
#9506=ADVANCED_FACE('',(#2528),#1008,.T.);
#9507=ADVANCED_FACE('',(#2529),#364,.T.);
#9508=ADVANCED_FACE('',(#2530),#365,.T.);
#9509=ADVANCED_FACE('',(#2531),#366,.F.);
#9510=ADVANCED_FACE('',(#2532),#367,.F.);
#9511=ADVANCED_FACE('',(#2533),#368,.F.);
#9512=ADVANCED_FACE('',(#2534),#369,.F.);
#9513=ADVANCED_FACE('',(#2535),#277,.T.);
#9514=ADVANCED_FACE('',(#2536),#370,.F.);
#9515=ADVANCED_FACE('',(#2537),#371,.F.);
#9516=ADVANCED_FACE('',(#2538),#372,.T.);
#9517=ADVANCED_FACE('',(#2539),#373,.T.);
#9518=ADVANCED_FACE('',(#2540),#374,.T.);
#9519=ADVANCED_FACE('',(#2541),#375,.F.);
#9520=ADVANCED_FACE('',(#2542),#376,.F.);
#9521=ADVANCED_FACE('',(#2543),#377,.F.);
#9522=ADVANCED_FACE('',(#2544),#278,.T.);
#9523=ADVANCED_FACE('',(#2545),#378,.T.);
#9524=ADVANCED_FACE('',(#2546),#379,.T.);
#9525=ADVANCED_FACE('',(#2547),#2289,.F.);
#9526=ADVANCED_FACE('',(#2548),#1009,.T.);
#9527=ADVANCED_FACE('',(#2549),#2290,.F.);
#9528=ADVANCED_FACE('',(#2550),#380,.T.);
#9529=ADVANCED_FACE('',(#2551),#2291,.F.);
#9530=ADVANCED_FACE('',(#2552),#2292,.F.);
#9531=ADVANCED_FACE('',(#2553),#2293,.F.);
#9532=ADVANCED_FACE('',(#2554),#2294,.F.);
#9533=ADVANCED_FACE('',(#2555),#1010,.T.);
#9534=ADVANCED_FACE('',(#2556),#1011,.T.);
#9535=ADVANCED_FACE('',(#2557),#1012,.T.);
#9881=CLOSED_SHELL('',(#9380,#9381,#9382,#9383,#9384,#9385,#9386,#9387,
#9388,#9389,#9390,#9391,#9392,#9393,#9394,#9395,#9396,#9397,#9398,#9399,
#9400,#9401,#9402,#9403,#9404,#9405,#9406,#9407,#9408,#9409,#9410,#9411,
#9412,#9413,#9414,#9415,#9416,#9417,#9418,#9419,#9420,#9421,#9422,#9423,
#9424,#9425,#9426,#9427,#9428,#9429,#9430,#9431,#9432,#9433,#9434,#9435,
#9436,#9437,#9438,#9439,#9440,#9441,#9442,#9443,#9444,#9445,#9446,#9447,
#9448,#9449,#9450,#9451,#9452,#9453,#9454,#9455,#9456,#9457,#9458,#9459,
#9460,#9461,#9462,#9463,#9464,#9465,#9466,#9467,#9468,#9469,#9470,#9471,
#9472,#9473,#9474,#9475,#9476,#9477,#9478,#9479,#9480,#9481,#9482,#9483,
#9484,#9485,#9486,#9487,#9488,#9489,#9490,#9491,#9492,#9493,#9494,#9495,
#9496,#9497,#9498,#9499,#9500,#9501,#9502,#9503,#9504,#9505,#9506,#9507,
#9508,#9509,#9510,#9511,#9512,#9513,#9514,#9515,#9516,#9517,#9518,#9519,
#9520,#9521,#9522,#9523,#9524,#9525,#9526,#9527,#9528,#9529,#9530,#9531,
#9532,#9533,#9534,#9535));
#10099=AXIS2_PLACEMENT_3D('',#13218,#10961,#10962);
#10100=AXIS2_PLACEMENT_3D('',#13219,#10963,#10964);
#10101=AXIS2_PLACEMENT_3D('',#13222,#10965,#10966);
#10102=AXIS2_PLACEMENT_3D('',#13224,#10967,#10968);
#10103=AXIS2_PLACEMENT_3D('',#13225,#10969,#10970);
#10104=AXIS2_PLACEMENT_3D('',#13226,#10971,#10972);
#10105=AXIS2_PLACEMENT_3D('',#13227,#10973,#10974);
#10106=AXIS2_PLACEMENT_3D('',#13231,#10976,#10977);
#10107=AXIS2_PLACEMENT_3D('',#13232,#10978,#10979);
#10108=AXIS2_PLACEMENT_3D('',#13233,#10980,#10981);
#10109=AXIS2_PLACEMENT_3D('',#13247,#10985,#10986);
#10110=AXIS2_PLACEMENT_3D('',#13282,#10987,#10988);
#10111=AXIS2_PLACEMENT_3D('',#13284,#10989,#10990);
#10112=AXIS2_PLACEMENT_3D('',#13285,#10991,#10992);
#10113=AXIS2_PLACEMENT_3D('',#13286,#10993,#10994);
#10114=AXIS2_PLACEMENT_3D('',#13404,#10996,#10997);
#10115=AXIS2_PLACEMENT_3D('',#13407,#10998,#10999);
#10116=AXIS2_PLACEMENT_3D('',#13409,#11000,#11001);
#10117=AXIS2_PLACEMENT_3D('',#13410,#11002,#11003);
#10118=AXIS2_PLACEMENT_3D('',#13411,#11004,#11005);
#10119=AXIS2_PLACEMENT_3D('',#13412,#11006,#11007);
#10120=AXIS2_PLACEMENT_3D('',#13416,#11009,#11010);
#10121=AXIS2_PLACEMENT_3D('',#13417,#11011,#11012);
#10122=AXIS2_PLACEMENT_3D('',#13418,#11013,#11014);
#10123=AXIS2_PLACEMENT_3D('',#13472,#11017,#11018);
#10124=AXIS2_PLACEMENT_3D('',#13474,#11019,#11020);
#10125=AXIS2_PLACEMENT_3D('',#13475,#11021,#11022);
#10126=AXIS2_PLACEMENT_3D('',#13476,#11023,#11024);
#10127=AXIS2_PLACEMENT_3D('',#13664,#11027,#11028);
#10128=AXIS2_PLACEMENT_3D('',#13666,#11030,#11031);
#10129=AXIS2_PLACEMENT_3D('',#13696,#11032,#11033);
#10130=AXIS2_PLACEMENT_3D('',#13698,#11035,#11036);
#10131=AXIS2_PLACEMENT_3D('',#13699,#11037,#11038);
#10132=AXIS2_PLACEMENT_3D('',#14266,#11039,#11040);
#10133=AXIS2_PLACEMENT_3D('',#14273,#11041,#11042);
#10134=AXIS2_PLACEMENT_3D('',#14274,#11043,#11044);
#10135=AXIS2_PLACEMENT_3D('',#14450,#11045,#11046);
#10136=AXIS2_PLACEMENT_3D('',#14476,#11047,#11048);
#10137=AXIS2_PLACEMENT_3D('',#14524,#11049,#11050);
#10138=AXIS2_PLACEMENT_3D('',#14538,#11051,#11052);
#10139=AXIS2_PLACEMENT_3D('',#14539,#11053,#11054);
#10140=AXIS2_PLACEMENT_3D('',#14597,#11055,#11056);
#10141=AXIS2_PLACEMENT_3D('',#14635,#11057,#11058);
#10142=AXIS2_PLACEMENT_3D('',#14657,#11059,#11060);
#10143=AXIS2_PLACEMENT_3D('',#14659,#11061,#11062);
#10144=AXIS2_PLACEMENT_3D('',#14688,#11063,#11064);
#10145=AXIS2_PLACEMENT_3D('',#14713,#11065,#11066);
#10146=AXIS2_PLACEMENT_3D('',#14795,#11067,#11068);
#10147=AXIS2_PLACEMENT_3D('',#14796,#11069,#11070);
#10148=AXIS2_PLACEMENT_3D('',#14797,#11071,#11072);
#10149=AXIS2_PLACEMENT_3D('',#14822,#11073,#11074);
#10150=AXIS2_PLACEMENT_3D('',#14854,#11076,#11077);
#10151=AXIS2_PLACEMENT_3D('',#14880,#11078,#11079);
#10152=AXIS2_PLACEMENT_3D('',#14930,#11080,#11081);
#10153=AXIS2_PLACEMENT_3D('',#14968,#11082,#11083);
#10154=AXIS2_PLACEMENT_3D('',#14990,#11084,#11085);
#10155=AXIS2_PLACEMENT_3D('',#15325,#11086,#11087);
#10156=AXIS2_PLACEMENT_3D('',#15797,#11090,#11091);
#10157=AXIS2_PLACEMENT_3D('',#15828,#11092,#11093);
#10158=AXIS2_PLACEMENT_3D('',#15837,#11094,#11095);
#10159=AXIS2_PLACEMENT_3D('',#15878,#11096,#11097);
#10160=AXIS2_PLACEMENT_3D('',#15883,#11098,#11099);
#10161=AXIS2_PLACEMENT_3D('',#15909,#11100,#11101);
#10162=AXIS2_PLACEMENT_3D('',#15910,#11102,#11103);
#10163=AXIS2_PLACEMENT_3D('',#15928,#11104,#11105);
#10164=AXIS2_PLACEMENT_3D('',#15930,#11106,#11107);
#10165=AXIS2_PLACEMENT_3D('',#15931,#11108,#11109);
#10166=AXIS2_PLACEMENT_3D('',#16012,#11111,#11112);
#10167=AXIS2_PLACEMENT_3D('',#16650,#11114,#11115);
#10168=AXIS2_PLACEMENT_3D('',#16767,#11116,#11117);
#10169=AXIS2_PLACEMENT_3D('',#16967,#11118,#11119);
#10170=AXIS2_PLACEMENT_3D('',#16969,#11120,#11121);
#10171=AXIS2_PLACEMENT_3D('',#16971,#11122,#11123);
#10172=AXIS2_PLACEMENT_3D('',#16999,#11124,#11125);
#10173=AXIS2_PLACEMENT_3D('',#17006,#11126,#11127);
#10174=AXIS2_PLACEMENT_3D('',#17033,#11128,#11129);
#10175=AXIS2_PLACEMENT_3D('',#17091,#11130,#11131);
#10176=AXIS2_PLACEMENT_3D('',#17092,#11132,#11133);
#10177=AXIS2_PLACEMENT_3D('',#17093,#11134,#11135);
#10178=AXIS2_PLACEMENT_3D('',#17094,#11136,#11137);
#10179=AXIS2_PLACEMENT_3D('',#17095,#11138,#11139);
#10180=AXIS2_PLACEMENT_3D('',#17096,#11140,#11141);
#10181=AXIS2_PLACEMENT_3D('',#17197,#11143,#11144);
#10182=AXIS2_PLACEMENT_3D('',#17754,#11146,#11147);
#10183=AXIS2_PLACEMENT_3D('',#17755,#11148,#11149);
#10184=AXIS2_PLACEMENT_3D('',#17779,#11152,#11153);
#10185=AXIS2_PLACEMENT_3D('',#17782,#11154,#11155);
#10186=AXIS2_PLACEMENT_3D('',#18333,#11158,#11159);
#10187=AXIS2_PLACEMENT_3D('',#18340,#11160,#11161);
#10188=AXIS2_PLACEMENT_3D('',#18368,#11162,#11163);
#10189=AXIS2_PLACEMENT_3D('',#18451,#11164,#11165);
#10190=AXIS2_PLACEMENT_3D('',#18499,#11166,#11167);
#10191=AXIS2_PLACEMENT_3D('',#18522,#11168,#11169);
#10192=AXIS2_PLACEMENT_3D('',#18674,#11170,#11171);
#10193=AXIS2_PLACEMENT_3D('',#18681,#11172,#11173);
#10194=AXIS2_PLACEMENT_3D('',#18717,#11174,#11175);
#10195=AXIS2_PLACEMENT_3D('',#18744,#11176,#11177);
#10196=AXIS2_PLACEMENT_3D('',#18745,#11178,#11179);
#10197=AXIS2_PLACEMENT_3D('',#18746,#11180,#11181);
#10198=AXIS2_PLACEMENT_3D('',#18834,#11182,#11183);
#10199=AXIS2_PLACEMENT_3D('',#18903,#11184,#11185);
#10200=AXIS2_PLACEMENT_3D('',#18905,#11187,#11188);
#10201=AXIS2_PLACEMENT_3D('',#18906,#11189,#11190);
#10202=AXIS2_PLACEMENT_3D('',#18907,#11191,#11192);
#10203=AXIS2_PLACEMENT_3D('',#18908,#11193,#11194);
#10204=AXIS2_PLACEMENT_3D('',#18909,#11195,#11196);
#10205=AXIS2_PLACEMENT_3D('',#20164,#11197,#11198);
#10206=AXIS2_PLACEMENT_3D('',#20165,#11199,#11200);
#10207=AXIS2_PLACEMENT_3D('',#20172,#11201,#11202);
#10208=AXIS2_PLACEMENT_3D('',#20176,#11204,#11205);
#10209=AXIS2_PLACEMENT_3D('',#20200,#11207,#11208);
#10210=AXIS2_PLACEMENT_3D('',#20207,#11209,#11210);
#10211=AXIS2_PLACEMENT_3D('',#20238,#11211,#11212);
#10212=AXIS2_PLACEMENT_3D('',#20265,#11213,#11214);
#10213=AXIS2_PLACEMENT_3D('',#20381,#11215,#11216);
#10214=AXIS2_PLACEMENT_3D('',#20431,#11217,#11218);
#10215=AXIS2_PLACEMENT_3D('',#20462,#11220,#11221);
#10216=AXIS2_PLACEMENT_3D('',#20585,#11222,#11223);
#10217=AXIS2_PLACEMENT_3D('',#20758,#11224,#11225);
#10218=AXIS2_PLACEMENT_3D('',#20761,#11227,#11228);
#10219=AXIS2_PLACEMENT_3D('',#20762,#11229,#11230);
#10220=AXIS2_PLACEMENT_3D('',#20811,#11232,#11233);
#10221=AXIS2_PLACEMENT_3D('',#20922,#11234,#11235);
#10222=AXIS2_PLACEMENT_3D('',#20945,#11236,#11237);
#10223=AXIS2_PLACEMENT_3D('',#20994,#11238,#11239);
#10224=AXIS2_PLACEMENT_3D('',#21019,#11240,#11241);
#10225=AXIS2_PLACEMENT_3D('',#21028,#11243,#11244);
#10226=AXIS2_PLACEMENT_3D('',#21034,#11247,#11248);
#10227=AXIS2_PLACEMENT_3D('',#21040,#11249,#11250);
#10228=AXIS2_PLACEMENT_3D('',#21051,#11253,#11254);
#10229=AXIS2_PLACEMENT_3D('',#21053,#11255,#11256);
#10230=AXIS2_PLACEMENT_3D('',#21055,#11257,#11258);
#10231=AXIS2_PLACEMENT_3D('',#21057,#11259,#11260);
#10232=AXIS2_PLACEMENT_3D('',#21058,#11261,#11262);
#10233=AXIS2_PLACEMENT_3D('',#21061,#11264,#11265);
#10234=AXIS2_PLACEMENT_3D('',#21062,#11266,#11267);
#10235=AXIS2_PLACEMENT_3D('',#21064,#11268,#11269);
#10236=AXIS2_PLACEMENT_3D('',#21068,#11271,#11272);
#10237=AXIS2_PLACEMENT_3D('',#21070,#11274,#11275);
#10238=AXIS2_PLACEMENT_3D('',#21073,#11277,#11278);
#10239=AXIS2_PLACEMENT_3D('',#21075,#11280,#11281);
#10240=AXIS2_PLACEMENT_3D('',#21076,#11282,#11283);
#10241=AXIS2_PLACEMENT_3D('',#21077,#11284,#11285);
#10242=AXIS2_PLACEMENT_3D('',#21078,#11286,#11287);
#10243=AXIS2_PLACEMENT_3D('',#21079,#11288,#11289);
#10244=AXIS2_PLACEMENT_3D('',#21082,#11291,#11292);
#10245=AXIS2_PLACEMENT_3D('',#21083,#11293,#11294);
#10246=AXIS2_PLACEMENT_3D('',#21096,#11297,#11298);
#10247=AXIS2_PLACEMENT_3D('',#21112,#11300,#11301);
#10248=AXIS2_PLACEMENT_3D('',#21192,#11309,#11310);
#10249=AXIS2_PLACEMENT_3D('',#21194,#11311,#11312);
#10250=AXIS2_PLACEMENT_3D('',#21196,#11313,#11314);
#10251=AXIS2_PLACEMENT_3D('',#21198,#11315,#11316);
#10252=AXIS2_PLACEMENT_3D('',#21220,#11317,#11318);
#10253=AXIS2_PLACEMENT_3D('',#21221,#11319,#11320);
#10254=AXIS2_PLACEMENT_3D('',#21243,#11321,#11322);
#10255=AXIS2_PLACEMENT_3D('',#21279,#11323,#11324);
#10256=AXIS2_PLACEMENT_3D('',#21287,#11325,#11326);
#10257=AXIS2_PLACEMENT_3D('',#21308,#11327,#11328);
#10258=AXIS2_PLACEMENT_3D('',#21326,#11329,#11330);
#10259=AXIS2_PLACEMENT_3D('',#21327,#11331,#11332);
#10260=AXIS2_PLACEMENT_3D('',#21328,#11333,#11334);
#10261=AXIS2_PLACEMENT_3D('',#21329,#11335,#11336);
#10262=AXIS2_PLACEMENT_3D('',#21857,#11338,#11339);
#10263=AXIS2_PLACEMENT_3D('',#21858,#11340,#11341);
#10264=AXIS2_PLACEMENT_3D('',#21859,#11342,#11343);
#10265=AXIS2_PLACEMENT_3D('',#21976,#11344,#11345);
#10266=AXIS2_PLACEMENT_3D('',#21978,#11346,#11347);
#10267=AXIS2_PLACEMENT_3D('',#22007,#11348,#11349);
#10268=AXIS2_PLACEMENT_3D('',#22008,#11350,#11351);
#10269=AXIS2_PLACEMENT_3D('',#22100,#11355,#11356);
#10270=AXIS2_PLACEMENT_3D('',#22101,#11357,#11358);
#10271=AXIS2_PLACEMENT_3D('',#22102,#11359,#11360);
#10272=AXIS2_PLACEMENT_3D('',#22103,#11361,#11362);
#10273=AXIS2_PLACEMENT_3D('',#22104,#11363,#11364);
#10274=AXIS2_PLACEMENT_3D('',#22117,#11366,#11367);
#10275=AXIS2_PLACEMENT_3D('',#22180,#11368,#11369);
#10276=AXIS2_PLACEMENT_3D('',#22181,#11370,#11371);
#10277=AXIS2_PLACEMENT_3D('',#22203,#11372,#11373);
#10278=AXIS2_PLACEMENT_3D('',#22205,#11374,#11375);
#10279=AXIS2_PLACEMENT_3D('',#22206,#11376,#11377);
#10280=AXIS2_PLACEMENT_3D('',#22480,#11378,#11379);
#10281=AXIS2_PLACEMENT_3D('',#22502,#11380,#11381);
#10282=AXIS2_PLACEMENT_3D('',#22523,#11382,#11383);
#10283=AXIS2_PLACEMENT_3D('',#22525,#11384,#11385);
#10284=AXIS2_PLACEMENT_3D('',#22526,#11386,#11387);
#10285=AXIS2_PLACEMENT_3D('',#22547,#11388,#11389);
#10286=AXIS2_PLACEMENT_3D('',#22548,#11390,#11391);
#10287=AXIS2_PLACEMENT_3D('',#22570,#11392,#11393);
#10288=AXIS2_PLACEMENT_3D('',#22676,#11396,#11397);
#10289=AXIS2_PLACEMENT_3D('',#22698,#11398,#11399);
#10290=AXIS2_PLACEMENT_3D('',#22723,#11400,#11401);
#10291=AXIS2_PLACEMENT_3D('',#22724,#11402,#11403);
#10292=AXIS2_PLACEMENT_3D('',#22725,#11404,#11405);
#10293=AXIS2_PLACEMENT_3D('',#22794,#11406,#11407);
#10294=AXIS2_PLACEMENT_3D('',#22796,#11409,#11410);
#10295=AXIS2_PLACEMENT_3D('',#22797,#11411,#11412);
#10296=AXIS2_PLACEMENT_3D('',#23319,#11414,#11415);
#10297=AXIS2_PLACEMENT_3D('',#23321,#11417,#11418);
#10298=AXIS2_PLACEMENT_3D('',#23323,#11420,#11421);
#10299=AXIS2_PLACEMENT_3D('',#23325,#11423,#11424);
#10300=AXIS2_PLACEMENT_3D('',#23327,#11426,#11427);
#10301=AXIS2_PLACEMENT_3D('',#23328,#11428,#11429);
#10302=AXIS2_PLACEMENT_3D('',#23329,#11430,#11431);
#10961=DIRECTION('axis',(0.,0.,1.));
#10962=DIRECTION('refdir',(1.,0.,0.));
#10963=DIRECTION('center_axis',(0.258819045102521,-0.965925826289068,0.));
#10964=DIRECTION('ref_axis',(0.,0.,-1.));
#10965=DIRECTION('center_axis',(-0.258819045102521,0.965925826289068,0.));
#10966=DIRECTION('ref_axis',(0.965925826289068,0.258819045102521,0.));
#10967=DIRECTION('center_axis',(-0.965925826289068,-0.258819045102521,0.));
#10968=DIRECTION('ref_axis',(0.,0.,1.));
#10969=DIRECTION('center_axis',(0.258819045102521,-0.965925826289068,0.));
#10970=DIRECTION('ref_axis',(0.965925826289068,0.258819045102521,0.));
#10971=DIRECTION('center_axis',(-0.258819045102521,0.965925826289068,0.));
#10972=DIRECTION('ref_axis',(0.965925826289068,0.258819045102521,0.));
#10973=DIRECTION('center_axis',(-0.258819045102521,0.965925826289068,0.));
#10974=DIRECTION('ref_axis',(0.965925826289068,0.258819045102521,0.));
#10975=DIRECTION('',(-0.258819045102521,0.965925826289068,0.));
#10976=DIRECTION('center_axis',(0.258819045102521,-0.965925826289068,0.));
#10977=DIRECTION('ref_axis',(0.965925826289068,0.258819045102521,0.));
#10978=DIRECTION('center_axis',(0.258819045102521,-0.965925826289068,0.));
#10979=DIRECTION('ref_axis',(0.965925826289068,0.258819045102521,0.));
#10980=DIRECTION('center_axis',(-0.258819045102521,0.965925826289068,0.));
#10981=DIRECTION('ref_axis',(0.965925826289068,0.258819045102521,0.));
#10982=DIRECTION('',(0.,0.,1.));
#10983=DIRECTION('',(0.,0.,1.));
#10984=DIRECTION('',(0.,0.,1.));
#10985=DIRECTION('center_axis',(0.258819045102337,-0.965925826289118,-1.46071306349284E-13));
#10986=DIRECTION('ref_axis',(0.177402769042635,0.0475349287001315,-0.982989668353375));
#10987=DIRECTION('center_axis',(0.258819045102521,-0.965925826289068,0.));
#10988=DIRECTION('ref_axis',(0.,0.,-1.));
#10989=DIRECTION('center_axis',(-0.258819045102521,0.965925826289068,0.));
#10990=DIRECTION('ref_axis',(0.965925826289068,0.258819045102521,0.));
#10991=DIRECTION('center_axis',(-0.965925826289068,-0.258819045102521,0.));
#10992=DIRECTION('ref_axis',(0.,0.,1.));
#10993=DIRECTION('center_axis',(-0.258819045102521,0.965925826289068,0.));
#10994=DIRECTION('ref_axis',(0.965925826289068,0.258819045102521,0.));
#10995=DIRECTION('',(0.,0.,-1.));
#10996=DIRECTION('center_axis',(-0.258819045102521,-0.965925826289068,0.));
#10997=DIRECTION('ref_axis',(0.,0.,-1.));
#10998=DIRECTION('center_axis',(0.258819045102521,0.965925826289068,0.));
#10999=DIRECTION('ref_axis',(0.965925826289068,-0.258819045102521,0.));
#11000=DIRECTION('center_axis',(-0.965925826289068,0.258819045102521,0.));
#11001=DIRECTION('ref_axis',(0.,0.,1.));
#11002=DIRECTION('center_axis',(-0.258819045102521,-0.965925826289068,0.));
#11003=DIRECTION('ref_axis',(0.965925826289068,-0.258819045102521,0.));
#11004=DIRECTION('center_axis',(0.258819045102521,0.965925826289068,0.));
#11005=DIRECTION('ref_axis',(0.965925826289068,-0.258819045102521,0.));
#11006=DIRECTION('center_axis',(0.258819045102521,0.965925826289068,0.));
#11007=DIRECTION('ref_axis',(0.965925826289068,-0.258819045102521,0.));
#11008=DIRECTION('',(0.258819045102521,0.965925826289068,0.));
#11009=DIRECTION('center_axis',(-0.258819045102521,-0.965925826289068,0.));
#11010=DIRECTION('ref_axis',(0.965925826289068,-0.258819045102521,0.));
#11011=DIRECTION('center_axis',(-0.258819045102521,-0.965925826289068,0.));
#11012=DIRECTION('ref_axis',(0.965925826289068,-0.258819045102521,0.));
#11013=DIRECTION('center_axis',(0.258819045102521,0.965925826289068,0.));
#11014=DIRECTION('ref_axis',(0.965925826289068,-0.258819045102521,0.));
#11015=DIRECTION('',(0.,0.,-1.));
#11016=DIRECTION('',(0.,0.,1.));
#11017=DIRECTION('center_axis',(-0.258819045102521,-0.965925826289068,0.));
#11018=DIRECTION('ref_axis',(0.,0.,-1.));
#11019=DIRECTION('center_axis',(0.258819045102521,0.965925826289068,0.));
#11020=DIRECTION('ref_axis',(0.965925826289068,-0.258819045102521,0.));
#11021=DIRECTION('center_axis',(-0.965925826289068,0.258819045102521,0.));
#11022=DIRECTION('ref_axis',(0.,0.,1.));
#11023=DIRECTION('center_axis',(0.258819045102521,0.965925826289068,0.));
#11024=DIRECTION('ref_axis',(0.965925826289068,-0.258819045102521,0.));
#11025=DIRECTION('',(0.,0.,-1.));
#11026=DIRECTION('',(-0.258819045102558,-0.965925826289058,0.));
#11027=DIRECTION('center_axis',(0.258819045102522,0.965925826289068,-8.7140221628902E-16));
#11028=DIRECTION('ref_axis',(0.965925826289068,-0.258819045102522,-5.55111512312583E-15));
#11029=DIRECTION('',(0.258819045102527,0.965925826289067,0.));
#11030=DIRECTION('center_axis',(0.,0.,1.));
#11031=DIRECTION('ref_axis',(0.500000000000001,-0.866025403784438,0.));
#11032=DIRECTION('center_axis',(0.,0.,1.));
#11033=DIRECTION('ref_axis',(-0.258819045102521,-0.965925826289068,0.));
#11034=DIRECTION('',(0.,0.,1.));
#11035=DIRECTION('center_axis',(-0.982489324426665,0.175514354454109,0.0625255049415299));
#11036=DIRECTION('ref_axis',(-0.186318886288095,-0.925515297832794,-0.329707000365231));
#11037=DIRECTION('center_axis',(0.338008733858616,-0.0905691672720826,-0.936774957914086));
#11038=DIRECTION('ref_axis',(-0.904855125270071,0.242455200083276,-0.349932390934396));
#11039=DIRECTION('center_axis',(-0.683496777669841,0.180523094083204,0.70727898838971));
#11040=DIRECTION('ref_axis',(-0.620872426437645,0.365761626196878,-0.693351182945011));
#11041=DIRECTION('center_axis',(-0.65831400371426,0.163876138290105,0.734688562462234));
#11042=DIRECTION('ref_axis',(-0.621487514031739,0.432351222926567,-0.653318980235957));
#11043=DIRECTION('center_axis',(-0.653921618105276,0.160745012694953,0.739288548719833));
#11044=DIRECTION('ref_axis',(-0.621897278706049,0.442272360574022,-0.646249900433488));
#11045=DIRECTION('center_axis',(-0.674075235079952,0.180617914877493,-0.716240006057476));
#11046=DIRECTION('ref_axis',(-0.258819045102521,-0.965925826289068,-3.01308868140017E-16));
#11047=DIRECTION('center_axis',(0.617002360972857,-0.165325284213947,-0.769399530123003));
#11048=DIRECTION('ref_axis',(0.286245910019278,-0.863567369973914,0.415108029931454));
#11049=DIRECTION('center_axis',(0.561902904510146,-0.150561429488195,-0.813385752182526));
#11050=DIRECTION('ref_axis',(0.558276694555572,-0.656562293339674,0.507201229573285));
#11051=DIRECTION('center_axis',(0.,0.,1.));
#11052=DIRECTION('ref_axis',(-0.534539664670774,-0.845143388362979,0.));
#11053=DIRECTION('center_axis',(-0.558874237830334,-0.749434485268718,-0.354975405598154));
#11054=DIRECTION('ref_axis',(0.558276694555565,-0.656562293339652,0.50720122957332));
#11055=DIRECTION('center_axis',(0.383424581050413,0.913295599568985,0.137392643377451));
#11056=DIRECTION('ref_axis',(-0.691543692210921,0.185298573858753,0.698163133006319));
#11057=DIRECTION('center_axis',(-0.250167531395729,-0.933637937572942,-0.256391122623056));
#11058=DIRECTION('ref_axis',(-0.965925826289068,0.258819045102521,-2.91742555544839E-17));
#11059=DIRECTION('center_axis',(-0.423012585798295,-0.887904844679767,-0.180790871037337));
#11060=DIRECTION('ref_axis',(0.273913532304164,-0.315488700307649,0.908536326625879));
#11061=DIRECTION('center_axis',(0.395037810900925,0.906269528225027,0.150401696032296));
#11062=DIRECTION('ref_axis',(-0.690739881421107,0.185083193406755,0.699015470310002));
#11063=DIRECTION('center_axis',(-0.428903026584179,-0.883790713143465,-0.186965689762311));
#11064=DIRECTION('ref_axis',(0.226054040298604,-0.305388776659452,0.925006630222249));
#11065=DIRECTION('center_axis',(0.694220983393908,-0.0865158721857753,-0.714543371724579));
#11066=DIRECTION('ref_axis',(-0.642354017365834,0.373397016182184,-0.669295140188703));
#11067=DIRECTION('center_axis',(-0.919731174770121,0.145681409008706,0.364515422479229));
#11068=DIRECTION('ref_axis',(0.303860786783007,-0.323674532104422,0.896048781887792));
#11069=DIRECTION('center_axis',(0.250253996385053,0.933960629306173,0.25512836024113));
#11070=DIRECTION('ref_axis',(0.713893553669226,-4.20541699587671E-15,-0.700254235281389));
#11071=DIRECTION('center_axis',(0.,0.,-1.));
#11072=DIRECTION('ref_axis',(0.,-1.,0.));
#11073=DIRECTION('center_axis',(-0.000608438188569021,-0.999999814768134,
-1.63299973368426E-5));
#11074=DIRECTION('ref_axis',(0.992173749069427,-0.000605715530870061,0.124863464497081));
#11075=DIRECTION('',(0.,0.,1.));
#11076=DIRECTION('center_axis',(0.250649702632458,0.935437425126364,0.249262011231594));
#11077=DIRECTION('ref_axis',(0.705141225886937,-3.98084930332909E-15,-0.709066887927131));
#11078=DIRECTION('center_axis',(0.250754597488213,0.935828898057517,0.247682065154054));
#11079=DIRECTION('ref_axis',(0.702734584093084,-1.83378449178784E-14,-0.711452109645843));
#11080=DIRECTION('center_axis',(0.140540951555781,0.524505971750252,-0.839727173869061));
#11081=DIRECTION('ref_axis',(0.424955852641996,-0.798002955152438,-0.427321666749171));
#11082=DIRECTION('center_axis',(-0.70009646922517,7.77263219592561E-15,
-0.71404827132236));
#11083=DIRECTION('ref_axis',(-0.71404827132236,2.32197393513232E-31,0.70009646922517));
#11084=DIRECTION('center_axis',(0.709066887926615,0.,0.705141225887457));
#11085=DIRECTION('ref_axis',(0.,1.,0.));
#11086=DIRECTION('center_axis',(-0.709066887926423,0.,0.70514122588765));
#11087=DIRECTION('ref_axis',(0.70514122588765,0.,0.709066887926423));
#11088=DIRECTION('',(0.,1.,0.));
#11089=DIRECTION('',(0.,1.,0.));
#11090=DIRECTION('center_axis',(0.709331039883401,-0.115502907144025,-0.695347793768854));
#11091=DIRECTION('ref_axis',(-0.0956309206562688,-0.993131507969492,0.0674131655737816));
#11092=DIRECTION('center_axis',(0.498818539794665,0.780955571567493,0.375883571860768));
#11093=DIRECTION('ref_axis',(-0.769313473215832,0.59870001961531,-0.222968756648148));
#11094=DIRECTION('center_axis',(-0.901161256199291,-0.00205051766332954,
-0.43347916409284));
#11095=DIRECTION('ref_axis',(-0.184974693085487,0.906194417947414,0.380257859614865));
#11096=DIRECTION('center_axis',(0.0190701713654315,0.92873814597838,0.37024557359776));
#11097=DIRECTION('ref_axis',(-0.88093921041517,0.1907406383142,-0.433086730861832));
#11098=DIRECTION('center_axis',(0.000264490323223583,0.341857053068283,
-0.939751927538506));
#11099=DIRECTION('ref_axis',(0.461132353426908,0.833829687993734,0.303455110425305));
#11100=DIRECTION('center_axis',(0.948694400412647,0.154852037999341,-0.275680577758279));
#11101=DIRECTION('ref_axis',(0.31381938810396,-0.354458336717562,0.88083862266676));
#11102=DIRECTION('center_axis',(1.06290398916907E-6,-0.342123200362749,
0.939655104691302));
#11103=DIRECTION('ref_axis',(0.120372757713139,-0.932822607049188,-0.339635662112345));
#11104=DIRECTION('center_axis',(-0.00180337743760444,0.342018865460073,
-0.939691355445617));
#11105=DIRECTION('ref_axis',(0.725796015895035,0.646870608951044,0.234048197143666));
#11106=DIRECTION('center_axis',(0.0160746645957318,0.949410867921572,0.313624949630195));
#11107=DIRECTION('ref_axis',(-0.881483570808126,0.16150693629599,-0.443736660558533));
#11108=DIRECTION('center_axis',(0.998612730749673,0.000484041380214348,
-0.0526533919954209));
#11109=DIRECTION('ref_axis',(0.0174203520886516,0.940611518756013,0.339037611654835));
#11110=DIRECTION('',(0.,0.939692620785908,0.342020143325669));
#11111=DIRECTION('center_axis',(0.08636525163809,0.995922297288841,0.0260733786151215));
#11112=DIRECTION('ref_axis',(0.978828013818433,-0.0799498801240489,-0.188424350953936));
#11113=DIRECTION('',(0.,1.,0.));
#11114=DIRECTION('center_axis',(0.998654787118421,0.0419942023103323,-0.0304155081788857));
#11115=DIRECTION('ref_axis',(0.0410790612416008,-0.998702024996989,-0.0301127214715466));
#11116=DIRECTION('center_axis',(0.0558943316700949,0.341485459772416,-0.93822358979679));
#11117=DIRECTION('ref_axis',(3.15158408626148E-17,-0.939692620785908,-0.34202014332567));
#11118=DIRECTION('center_axis',(-0.999999997425425,-6.29602249007253E-8,
7.1757557210404E-5));
#11119=DIRECTION('ref_axis',(6.29599482845205E-8,-0.999999999999998,-3.87634923658253E-9));
#11120=DIRECTION('center_axis',(0.,-1.,0.));
#11121=DIRECTION('ref_axis',(0.998606857012289,0.,0.0527668942428699));
#11122=DIRECTION('center_axis',(-0.499999999999997,2.40370335797946E-15,
0.866025403784441));
#11123=DIRECTION('ref_axis',(-0.86602540378444,-1.97523375096352E-30,-0.499999999999997));
#11124=DIRECTION('center_axis',(0.052566152876564,0.0871443475070821,-0.994807851933891));
#11125=DIRECTION('ref_axis',(-1.20857617498309E-18,-0.99618513361228,-0.0872649962463973));
#11126=DIRECTION('center_axis',(-0.0468293174424863,-0.283748024629802,
0.957754704267516));
#11127=DIRECTION('ref_axis',(-0.998806810296615,1.84862994057718E-6,-0.0488360082488711));
#11128=DIRECTION('center_axis',(0.26678747535128,-0.329623886957063,0.905633775950857));
#11129=DIRECTION('ref_axis',(-0.963721144476179,-0.0991646056426279,0.247806248261148));
#11130=DIRECTION('center_axis',(0.368750856924727,-0.317917392275649,0.873470856529244));
#11131=DIRECTION('ref_axis',(-0.929514851454483,-0.131167657818318,0.344669677325997));
#11132=DIRECTION('center_axis',(4.77253183189936E-13,-0.939692620785859,
-0.342020143325803));
#11133=DIRECTION('ref_axis',(0.96375164351186,0.0912513137134674,-0.250710923921866));
#11134=DIRECTION('center_axis',(0.0157117490853046,0.93086474670346,0.365025977548701));
#11135=DIRECTION('ref_axis',(0.320465643538016,-0.35050049031928,0.880029077700112));
#11136=DIRECTION('center_axis',(0.,0.,1.));
#11137=DIRECTION('ref_axis',(-0.713843353559374,-0.700305409502959,0.));
#11138=DIRECTION('center_axis',(0.000714845692164799,-0.935248614150113,
-0.353990845539725));
#11139=DIRECTION('ref_axis',(-0.929514851454482,-0.13116765781832,0.344669677325998));
#11140=DIRECTION('center_axis',(0.,0.939692620785908,0.342020143325669));
#11141=DIRECTION('ref_axis',(1.,0.,0.));
#11142=DIRECTION('',(1.,0.,0.));
#11143=DIRECTION('center_axis',(0.185962802483799,-0.914984054098916,-0.358081019934152));
#11144=DIRECTION('ref_axis',(-0.974399049469672,-0.218600131341872,0.0525402224007016));
#11145=DIRECTION('',(0.,-1.,0.));
#11146=DIRECTION('center_axis',(0.998286319297904,0.0169798943930786,0.0560009632867498));
#11147=DIRECTION('ref_axis',(0.0309996601200789,-0.96511714384739,-0.259976767662606));
#11148=DIRECTION('center_axis',(1.,0.,0.));
#11149=DIRECTION('ref_axis',(0.,-1.,0.));
#11150=DIRECTION('',(1.,0.,0.));
#11151=DIRECTION('',(0.,1.,0.));
#11152=DIRECTION('center_axis',(0.,1.,0.));
#11153=DIRECTION('ref_axis',(0.998040925216739,0.,0.0625644594999036));
#11154=DIRECTION('center_axis',(0.00136898756525043,0.999999062261074,3.67426066888223E-5));
#11155=DIRECTION('ref_axis',(0.999999062724686,-0.00136898831953958,2.0511696959745E-5));
#11156=DIRECTION('',(0.,-1.,0.));
#11157=DIRECTION('',(0.,1.,0.));
#11158=DIRECTION('center_axis',(0.0769992342443215,5.53463470572542E-15,
0.997031151933473));
#11159=DIRECTION('ref_axis',(0.372507740406449,0.927583081399946,-0.0287682192334328));
#11160=DIRECTION('center_axis',(-0.108282317724695,0.,-0.994120183714307));
#11161=DIRECTION('ref_axis',(0.,1.,0.));
#11162=DIRECTION('center_axis',(-0.147910770333402,0.,-0.98900070981743));
#11163=DIRECTION('ref_axis',(0.,1.,0.));
#11164=DIRECTION('center_axis',(0.179815697907154,0.,0.983700317569413));
#11165=DIRECTION('ref_axis',(0.191730437229931,0.980821655000061,-0.0350474039346959));
#11166=DIRECTION('center_axis',(-0.0593029104409559,-0.0158901669614693,
-0.998113554365017));
#11167=DIRECTION('ref_axis',(0.25881904510252,-0.965925826289068,2.91618690438022E-17));
#11168=DIRECTION('center_axis',(0.0698168329514292,0.0187073640074283,0.997384401506523));
#11169=DIRECTION('ref_axis',(-0.323156373260713,-0.945484767603846,0.0403548342839344));
#11170=DIRECTION('center_axis',(-0.0660314821081422,0.995510404849706,0.0678150219831547));
#11171=DIRECTION('ref_axis',(0.318920483681049,0.0854544860520815,-0.943921212762072));
#11172=DIRECTION('center_axis',(0.120185456360085,-0.985054343375952,-0.1233831296235));
#11173=DIRECTION('ref_axis',(-0.716328254484438,5.16215345872698E-16,-0.697763449764516));
#11174=DIRECTION('center_axis',(-0.626869024663385,0.756269149073557,-0.187329122341225));
#11175=DIRECTION('ref_axis',(0.401601466608204,0.107608788656578,-0.909470511133815));
#11176=DIRECTION('center_axis',(0.197508325342163,-0.959113442520952,-0.202711286800078));
#11177=DIRECTION('ref_axis',(-0.716238835403652,1.06988830219121E-14,-0.697855236176974));
#11178=DIRECTION('center_axis',(-0.716109385358714,5.87931396607782E-5,
-0.697988069199275));
#11179=DIRECTION('ref_axis',(-0.68756150283332,-0.172259653507989,0.705397612410826));
#11180=DIRECTION('center_axis',(0.716109496908384,-5.89002338248414E-5,
0.697987954744481));
#11181=DIRECTION('ref_axis',(-0.669323575897851,-0.283691166714552,0.686676978407934));
#11182=DIRECTION('center_axis',(0.452203132506872,-0.164412726418077,-0.876630356731243));
#11183=DIRECTION('ref_axis',(-0.554785176563544,0.717736695451074,-0.42079382584388));
#11184=DIRECTION('center_axis',(-0.258819045102521,0.965925826289068,-3.93157553907421E-15));
#11185=DIRECTION('ref_axis',(-0.965925826289068,-0.258819045102521,2.22044604925036E-14));
#11186=DIRECTION('',(-0.258819045102524,0.965925826289068,0.));
#11187=DIRECTION('center_axis',(-0.999923926773649,0.0102397286101005,-0.00687667241892065));
#11188=DIRECTION('ref_axis',(-0.0123345314287038,-0.830104467290876,0.557471463590887));
#11189=DIRECTION('center_axis',(0.,0.,-1.));
#11190=DIRECTION('ref_axis',(0.258819045325331,-0.965925826229366,0.));
#11191=DIRECTION('center_axis',(-0.674252347930799,-0.180665372122846,0.716061306471393));
#11192=DIRECTION('ref_axis',(0.691662109127011,0.185330303575785,0.698037395398328));
#11193=DIRECTION('center_axis',(0.,0.,1.));
#11194=DIRECTION('ref_axis',(-0.500000000000001,-0.866025403784438,0.));
#11195=DIRECTION('center_axis',(-0.695628388101101,0.0314971703251269,-0.717710996104542));
#11196=DIRECTION('ref_axis',(0.716946879324803,-0.03311269790395,-0.696340952022749));
#11197=DIRECTION('center_axis',(0.258111243842629,0.0691606993450251,0.96363654116483));
#11198=DIRECTION('ref_axis',(0.258819045102521,-0.965925826289068,-2.93972626113222E-17));
#11199=DIRECTION('center_axis',(-0.965925826289068,-0.258819045102521,0.));
#11200=DIRECTION('ref_axis',(0.,0.,1.));
#11201=DIRECTION('center_axis',(1.,0.,0.));
#11202=DIRECTION('ref_axis',(0.,-0.707106781186547,-0.707106781186548));
#11203=DIRECTION('',(-1.,0.,0.));
#11204=DIRECTION('center_axis',(1.,0.,0.));
#11205=DIRECTION('ref_axis',(0.,-1.,0.));
#11206=DIRECTION('',(1.,0.,0.));
#11207=DIRECTION('center_axis',(0.0468234603154239,-0.283756854133083,0.95775237472772));
#11208=DIRECTION('ref_axis',(3.26081672821954E-17,-0.958804009877884,-0.284068425985871));
#11209=DIRECTION('center_axis',(-0.0525661528831979,0.0871443475057628,
-0.994807851933656));
#11210=DIRECTION('ref_axis',(0.998606857012238,-6.04578193157126E-18,-0.0527668942438301));
#11211=DIRECTION('center_axis',(-0.499999999999829,-1.34607388046865E-13,
-0.866025403784538));
#11212=DIRECTION('ref_axis',(0.866025403784538,1.92284846106144E-30,-0.499999999999829));
#11213=DIRECTION('center_axis',(-0.266795615085176,-0.329622984395579,0.905631706561489));
#11214=DIRECTION('ref_axis',(-1.17693390083123E-12,-0.939692620785966,-0.342020143325511));
#11215=DIRECTION('center_axis',(-3.84846287078961E-13,-0.939692620785867,
-0.342020143325782));
#11216=DIRECTION('ref_axis',(-0.929470733634111,0.126169814813646,-0.346648717216086));
#11217=DIRECTION('center_axis',(0.998804703166064,1.69786870596043E-5,-0.0488790818763427));
#11218=DIRECTION('ref_axis',(0.0170818764593461,0.936825466105722,0.349379815605343));
#11219=DIRECTION('',(0.,1.,0.));
#11220=DIRECTION('center_axis',(0.0155776059735878,0.947746103906714,0.318645038752805));
#11221=DIRECTION('ref_axis',(-0.846028382887146,0.182343886514573,-0.50098571077439));
#11222=DIRECTION('center_axis',(0.0312572139148635,0.341853023360818,-0.93923346245614));
#11223=DIRECTION('ref_axis',(-4.36812986433843E-19,-0.939692620785908,-0.342020143325669));
#11224=DIRECTION('center_axis',(0.,0.939692620785908,0.342020143325669));
#11225=DIRECTION('ref_axis',(1.,0.,0.));
#11226=DIRECTION('',(1.,0.,0.));
#11227=DIRECTION('center_axis',(4.78283496086397E-13,-0.939692620785863,
-0.342020143325795));
#11228=DIRECTION('ref_axis',(0.971659954583462,0.0808477547528646,-0.222127380595651));
#11229=DIRECTION('center_axis',(1.,0.,0.));
#11230=DIRECTION('ref_axis',(0.,-1.,0.));
#11231=DIRECTION('',(1.,0.,0.));
#11232=DIRECTION('center_axis',(0.700096469223959,-7.77263219591216E-15,
-0.714048271323547));
#11233=DIRECTION('ref_axis',(0.714048271323547,8.33364844194403E-32,0.700096469223959));
#11234=DIRECTION('center_axis',(0.709066887927214,0.,0.705141225886854));
#11235=DIRECTION('ref_axis',(-0.705141225886854,0.,0.709066887927214));
#11236=DIRECTION('center_axis',(-0.709066887925823,0.,0.705141225888253));
#11237=DIRECTION('ref_axis',(0.,-1.,0.));
#11238=DIRECTION('center_axis',(-0.70009646922517,-2.33178965877769E-14,
-0.71404827132236));
#11239=DIRECTION('ref_axis',(3.33066907387548E-14,-1.,4.30601063609922E-29));
#11240=DIRECTION('center_axis',(0.,0.,1.));
#11241=DIRECTION('ref_axis',(0.,-1.,0.));
#11242=DIRECTION('',(0.,0.,1.));
#11243=DIRECTION('center_axis',(0.,1.,0.));
#11244=DIRECTION('ref_axis',(1.,0.,0.));
#11245=DIRECTION('',(-1.,0.,0.));
#11246=DIRECTION('',(0.,0.,-1.));
#11247=DIRECTION('center_axis',(-1.50215510448877E-15,-1.,2.30138252825371E-14));
#11248=DIRECTION('ref_axis',(-0.999999999791142,1.50262546286449E-15,2.04380924802295E-5));
#11249=DIRECTION('center_axis',(-5.46390275282226E-14,-1.,9.03906656443215E-15));
#11250=DIRECTION('ref_axis',(0.410021673945177,-3.0647499209318E-14,-0.912075779140744));
#11251=DIRECTION('',(0.,0.,1.));
#11252=DIRECTION('',(1.,0.,0.));
#11253=DIRECTION('center_axis',(0.,-1.,0.));
#11254=DIRECTION('ref_axis',(1.,0.,0.));
#11255=DIRECTION('center_axis',(0.,-1.,0.));
#11256=DIRECTION('ref_axis',(1.,0.,0.));
#11257=DIRECTION('center_axis',(0.,-1.,0.));
#11258=DIRECTION('ref_axis',(1.,0.,0.));
#11259=DIRECTION('center_axis',(0.,-1.,0.));
#11260=DIRECTION('ref_axis',(1.,0.,0.));
#11261=DIRECTION('center_axis',(1.,0.,0.));
#11262=DIRECTION('ref_axis',(0.,-0.707106781186547,-0.707106781186548));
#11263=DIRECTION('',(1.,0.,0.));
#11264=DIRECTION('center_axis',(-1.,0.,0.));
#11265=DIRECTION('ref_axis',(0.,0.,-1.));
#11266=DIRECTION('center_axis',(0.,1.,0.));
#11267=DIRECTION('ref_axis',(0.707106781186547,0.,-0.707106781186547));
#11268=DIRECTION('center_axis',(0.,1.,0.));
#11269=DIRECTION('ref_axis',(1.,0.,-1.11022302462516E-14));
#11270=DIRECTION('',(0.,1.,0.));
#11271=DIRECTION('center_axis',(0.,-1.,0.));
#11272=DIRECTION('ref_axis',(0.,0.,-1.));
#11273=DIRECTION('',(0.,-1.,0.));
#11274=DIRECTION('center_axis',(-1.,0.,0.));
#11275=DIRECTION('ref_axis',(0.,0.707106781186547,-0.707106781186548));
#11276=DIRECTION('',(1.,0.,0.));
#11277=DIRECTION('center_axis',(-1.,0.,0.));
#11278=DIRECTION('ref_axis',(0.,1.,-1.11022302462516E-14));
#11279=DIRECTION('',(-1.,0.,0.));
#11280=DIRECTION('center_axis',(-0.408248290463859,-0.408248290463862,-0.816496580927729));
#11281=DIRECTION('ref_axis',(0.577350269189625,0.57735026918963,-0.577350269189623));
#11282=DIRECTION('center_axis',(0.,0.,-1.));
#11283=DIRECTION('ref_axis',(0.707106781186549,0.707106781186546,0.));
#11284=DIRECTION('center_axis',(-0.408248290463859,0.408248290463861,-0.816496580927729));
#11285=DIRECTION('ref_axis',(0.577350269189625,-0.577350269189629,-0.577350269189623));
#11286=DIRECTION('center_axis',(0.,0.,-1.));
#11287=DIRECTION('ref_axis',(0.707106781186549,-0.707106781186546,0.));
#11288=DIRECTION('center_axis',(0.,0.,1.));
#11289=DIRECTION('ref_axis',(0.707106781186548,-0.707106781186547,0.));
#11290=DIRECTION('',(0.,0.,1.));
#11291=DIRECTION('center_axis',(0.,0.,-1.));
#11292=DIRECTION('ref_axis',(1.,0.,0.));
#11293=DIRECTION('center_axis',(1.,0.,0.));
#11294=DIRECTION('ref_axis',(0.,0.,-1.));
#11295=DIRECTION('',(0.,0.,-1.));
#11296=DIRECTION('',(0.,1.,0.));
#11297=DIRECTION('center_axis',(0.,0.,-1.));
#11298=DIRECTION('ref_axis',(0.707106781186548,0.707106781186547,0.));
#11299=DIRECTION('',(0.,0.,1.));
#11300=DIRECTION('center_axis',(0.,1.,0.));
#11301=DIRECTION('ref_axis',(1.,0.,0.));
#11302=DIRECTION('',(-1.,0.,0.));
#11303=DIRECTION('',(-1.,0.,0.));
#11304=DIRECTION('',(0.,0.,1.));
#11305=DIRECTION('',(0.,0.,1.));
#11306=DIRECTION('',(0.,0.,-1.));
#11307=DIRECTION('',(-1.,0.,0.));
#11308=DIRECTION('',(-1.,0.,0.));
#11309=DIRECTION('center_axis',(0.,-1.,0.));
#11310=DIRECTION('ref_axis',(1.,0.,0.));
#11311=DIRECTION('center_axis',(0.,-1.,0.));
#11312=DIRECTION('ref_axis',(1.,0.,0.));
#11313=DIRECTION('center_axis',(0.,-1.,0.));
#11314=DIRECTION('ref_axis',(1.,0.,0.));
#11315=DIRECTION('center_axis',(0.,-1.,0.));
#11316=DIRECTION('ref_axis',(1.,0.,0.));
#11317=DIRECTION('center_axis',(-0.124883782089936,0.,-0.99217137681497));
#11318=DIRECTION('ref_axis',(0.99217137681497,0.,-0.124883782089936));
#11319=DIRECTION('center_axis',(0.,1.,0.));
#11320=DIRECTION('ref_axis',(-0.992173928994009,0.,0.124863503973705));
#11321=DIRECTION('center_axis',(-0.215465317990859,0.,-0.97651149340041));
#11322=DIRECTION('ref_axis',(0.97651149340041,-5.55111512312577E-15,-0.215465317990859));
#11323=DIRECTION('center_axis',(0.384746145047863,4.23953194639129E-13,
0.923022428693262));
#11324=DIRECTION('ref_axis',(-3.05311331771915E-12,-1.,1.73194791841523E-12));
#11325=DIRECTION('center_axis',(-0.74869039128462,-0.200610985725532,0.631836949223701));
#11326=DIRECTION('ref_axis',(-0.324728217067871,-0.719949447827078,-0.613371321153351));
#11327=DIRECTION('center_axis',(0.0982582777590185,0.957717020306253,0.270413423978069));
#11328=DIRECTION('ref_axis',(0.127909569660762,-0.281628557964879,0.950959776924251));
#11329=DIRECTION('center_axis',(-0.65684684485648,-0.176001581630224,0.733195516670518));
#11330=DIRECTION('ref_axis',(-0.437553251543722,-0.702943249076073,-0.560729828564426));
#11331=DIRECTION('center_axis',(-0.264383392923062,0.919236580826271,0.291728521089929));
#11332=DIRECTION('ref_axis',(0.07007383801871,-0.283382405581138,0.95644344810991));
#11333=DIRECTION('center_axis',(0.,0.,1.));
#11334=DIRECTION('ref_axis',(1.,0.,0.));
#11335=DIRECTION('center_axis',(0.363488148886145,-0.708643875710738,0.604731529719585));
#11336=DIRECTION('ref_axis',(-0.437553251543735,-0.702943249076031,-0.560729828564468));
#11337=DIRECTION('',(0.,-1.,0.));
#11338=DIRECTION('center_axis',(0.,-1.,0.));
#11339=DIRECTION('ref_axis',(-0.998040925216754,0.,0.0625644594996687));
#11340=DIRECTION('center_axis',(0.163972207190969,0.540732729492925,0.82505831946842));
#11341=DIRECTION('ref_axis',(-0.984161974111908,0.0325543710521824,0.174256769273245));
#11342=DIRECTION('center_axis',(0.,0.,-1.));
#11343=DIRECTION('ref_axis',(-1.,0.,0.));
#11344=DIRECTION('center_axis',(-0.771919959919765,-0.0808086527971774,
-0.630562873241499));
#11345=DIRECTION('ref_axis',(0.0625870122150387,-0.99672963314136,0.0511165757840384));
#11346=DIRECTION('center_axis',(0.700096469223959,1.55452643918243E-14,
-0.714048271323547));
#11347=DIRECTION('ref_axis',(-2.22044604925031E-14,1.,-3.53183321097136E-30));
#11348=DIRECTION('center_axis',(0.,0.,-1.));
#11349=DIRECTION('ref_axis',(0.,-1.,0.));
#11350=DIRECTION('center_axis',(0.,0.,1.));
#11351=DIRECTION('ref_axis',(0.,-1.,0.));
#11352=DIRECTION('',(0.,-1.,-6.48452891646315E-16));
#11353=DIRECTION('',(0.,1.,0.));
#11354=DIRECTION('',(0.447898727755213,0.894084296738994,0.));
#11355=DIRECTION('center_axis',(-1.13908027475977E-11,1.,1.26463314793467E-25));
#11356=DIRECTION('ref_axis',(1.11022302462518E-14,3.05100033046494E-40,
1.));
#11357=DIRECTION('center_axis',(0.,0.,-1.));
#11358=DIRECTION('ref_axis',(-1.,0.,0.));
#11359=DIRECTION('center_axis',(1.76229903791608E-12,9.84552143939818E-13,
-1.));
#11360=DIRECTION('ref_axis',(-0.890482609600958,-0.455017276593172,-2.01698753190003E-12));
#11361=DIRECTION('center_axis',(0.,0.,-1.));
#11362=DIRECTION('ref_axis',(-1.,0.,0.));
#11363=DIRECTION('center_axis',(-1.,0.,0.));
#11364=DIRECTION('ref_axis',(0.,0.,1.));
#11365=DIRECTION('',(0.,-1.,0.));
#11366=DIRECTION('center_axis',(-5.20040241961378E-7,-0.999999999999865,
5.77360650357171E-21));
#11367=DIRECTION('ref_axis',(0.999398340012359,-5.19727354555897E-7,0.0346836846409219));
#11368=DIRECTION('center_axis',(0.0377485314798384,0.276390855786013,-0.960303672391703));
#11369=DIRECTION('ref_axis',(-0.999228297332728,-4.13963359097666E-15,-0.0392786177141947));
#11370=DIRECTION('center_axis',(-0.998948438150501,0.0354752832048574,-0.0290434536205597));
#11371=DIRECTION('ref_axis',(-0.0305542913919211,-0.98741517219653,-0.155169948745348));
#11372=DIRECTION('center_axis',(0.263764010584037,0.923513515076835,0.278480401807835));
#11373=DIRECTION('ref_axis',(0.891000137487118,-0.343866627487043,0.296436329586345));
#11374=DIRECTION('center_axis',(0.169401090369437,-0.337076992361637,0.926111425154705));
#11375=DIRECTION('ref_axis',(4.54657600793298E-17,0.939692620788689,0.342020143318028));
#11376=DIRECTION('center_axis',(-0.554161596073854,-0.802096420655957,-0.222589886130932));
#11377=DIRECTION('ref_axis',(0.831536970603906,-0.545659536114231,-0.103932368232812));
#11378=DIRECTION('center_axis',(0.0310203232622331,0.341855547490705,-0.939240397446009));
#11379=DIRECTION('ref_axis',(-0.999518753973484,0.0106095754081624,-0.0291495688639121));
#11380=DIRECTION('center_axis',(-0.0569607767181947,0.341464845217121,-0.938166951771649));
#11381=DIRECTION('ref_axis',(2.16317518465542E-9,0.939692620828124,0.342020143209682));
#11382=DIRECTION('center_axis',(0.,0.,1.));
#11383=DIRECTION('ref_axis',(-0.736625730662687,0.676300623188876,0.));
#11384=DIRECTION('center_axis',(-0.000471408636173,0.934389008169434,0.356254065501068));
#11385=DIRECTION('ref_axis',(-0.972631522480859,-0.0832049765466535,0.216944355433455));
#11386=DIRECTION('center_axis',(-0.232320635143996,0.332662217771895,-0.913981931633976));
#11387=DIRECTION('ref_axis',(-0.972631522480859,-0.0832049765466558,0.216944355433454));
#11388=DIRECTION('center_axis',(-0.0123951381577513,-0.927528497526217,
-0.373546846897158));
#11389=DIRECTION('ref_axis',(-0.203183137824287,0.368118154650563,-0.907306804074863));
#11390=DIRECTION('center_axis',(8.47652041731572E-13,0.939692620785858,
0.342020143325808));
#11391=DIRECTION('ref_axis',(0.201508985660445,-0.335004169860873,0.920416392114963));
#11392=DIRECTION('center_axis',(0.000457813874219378,-0.9345848157438,-0.355740091341395));
#11393=DIRECTION('ref_axis',(-0.943802615278056,-0.117979263083487,0.308735350869606));
#11394=DIRECTION('',(0.,0.939692620785908,0.342020143325669));
#11395=DIRECTION('',(0.,-1.,0.));
#11396=DIRECTION('center_axis',(-0.0490673383431336,-0.288968791309725,
0.956080244517644));
#11397=DIRECTION('ref_axis',(-0.998685654811338,1.09394001838749E-14,-0.0512539059394343));
#11398=DIRECTION('center_axis',(0.236372695682419,-0.332328136044342,0.913064049631306));
#11399=DIRECTION('ref_axis',(-0.971626941679023,-0.0888766187212934,0.21918492842378));
#11400=DIRECTION('center_axis',(0.33047220550483,-0.322803989289558,0.886896671482941));
#11401=DIRECTION('ref_axis',(-0.943802615278055,-0.117979263083488,0.308735350869608));
#11402=DIRECTION('center_axis',(0.0160970752919315,0.928887250896035,0.370012647472829));
#11403=DIRECTION('ref_axis',(0.286399133952083,-0.358838253610397,0.888375283209375));
#11404=DIRECTION('center_axis',(0.,0.,1.));
#11405=DIRECTION('ref_axis',(-0.710878052583325,-0.703315288014799,0.));
#11406=DIRECTION('center_axis',(1.,0.,0.));
#11407=DIRECTION('ref_axis',(0.,-1.,0.));
#11408=DIRECTION('',(1.,0.,0.));
#11409=DIRECTION('center_axis',(0.,0.,-1.));
#11410=DIRECTION('ref_axis',(-1.,0.,0.));
#11411=DIRECTION('center_axis',(1.,0.,0.));
#11412=DIRECTION('ref_axis',(0.,-1.,0.));
#11413=DIRECTION('',(1.,0.,0.));
#11414=DIRECTION('center_axis',(0.,1.,0.));
#11415=DIRECTION('ref_axis',(1.,0.,0.));
#11416=DIRECTION('',(0.,1.,0.));
#11417=DIRECTION('center_axis',(0.,1.,0.));
#11418=DIRECTION('ref_axis',(1.,0.,0.));
#11419=DIRECTION('',(0.,1.,0.));
#11420=DIRECTION('center_axis',(0.,1.,0.));
#11421=DIRECTION('ref_axis',(1.,0.,0.));
#11422=DIRECTION('',(0.,1.,0.));
#11423=DIRECTION('center_axis',(0.,1.,0.));
#11424=DIRECTION('ref_axis',(1.,0.,0.));
#11425=DIRECTION('',(0.,1.,0.));
#11426=DIRECTION('center_axis',(0.,0.939692620785908,0.342020143325669));
#11427=DIRECTION('ref_axis',(1.,0.,0.));
#11428=DIRECTION('center_axis',(0.965925826289068,-0.258819045102521,0.));
#11429=DIRECTION('ref_axis',(0.,0.,-1.));
#11430=DIRECTION('center_axis',(0.,0.939692620785908,0.342020143325669));
#11431=DIRECTION('ref_axis',(1.,0.,0.));
#13218=CARTESIAN_POINT('',(0.,0.,0.));
#13219=CARTESIAN_POINT('Origin',(5.91049210772187,0.55689895383893,8.58));
#13220=CARTESIAN_POINT('',(4.60649224223163,0.207493242950527,8.58));
#13221=CARTESIAN_POINT('',(5.91049210772187,0.55689895383893,9.93));
#13222=CARTESIAN_POINT('Origin',(5.91049210772187,0.55689895383893,8.58));
#13223=CARTESIAN_POINT('',(5.93637401223212,0.460306371210023,10.03));
#13224=CARTESIAN_POINT('Origin',(5.91049210772187,0.55689895383893,10.03));
#13225=CARTESIAN_POINT('Origin',(5.93637401223212,0.460306371210023,8.58));
#13226=CARTESIAN_POINT('Origin',(5.91049210772187,0.55689895383893,8.58));
#13227=CARTESIAN_POINT('Origin',(5.93637401223212,0.460306371210023,8.58));
#13228=CARTESIAN_POINT('',(4.52884652870087,0.497270990837247,8.58));
#13229=CARTESIAN_POINT('',(4.63237414674188,0.110900660321619,8.58));
#13230=CARTESIAN_POINT('',(5.83284639419111,0.84667670172565,9.93));
#13231=CARTESIAN_POINT('Origin',(5.83284639419111,0.84667670172565,8.58));
#13232=CARTESIAN_POINT('Origin',(5.83284639419111,0.84667670172565,8.58));
#13233=CARTESIAN_POINT('Origin',(6.30001167592482,0.557742789534021,7.49483504398303));
#13234=CARTESIAN_POINT('',(4.41021120669539,0.05137227994804,11.5901922029304));
#13235=CARTESIAN_POINT('',(4.41021120671322,0.0513722799528162,11.7069738861252));
#13236=CARTESIAN_POINT('',(4.41021120669539,0.05137227994804,5.29092677993983));
#13237=CARTESIAN_POINT('',(4.33293714059227,0.0306667563398384,11.6657994729934));
#13238=CARTESIAN_POINT('Ctrl Pts',(4.33293714059226,0.0306667563398384,
11.6657994729934));
#13239=CARTESIAN_POINT('Ctrl Pts',(4.35772155918772,0.0373077212873651,
11.6410754279018));
#13240=CARTESIAN_POINT('Ctrl Pts',(4.38339811720808,0.044187734273338,11.6158676377922));
#13241=CARTESIAN_POINT('Ctrl Pts',(4.41021120669538,0.0513722799480404,
11.5901922029304));
#13242=CARTESIAN_POINT('',(4.33293714061332,0.0306667563454775,11.573751331703));
#13243=CARTESIAN_POINT('',(4.33293714059227,0.0306667563398384,-0.5));
#13244=CARTESIAN_POINT('',(4.33293714059219,0.0306667563398168,3.61523506307464));
#13245=CARTESIAN_POINT('',(4.33293714059227,0.0306667563398384,-0.5));
#13246=CARTESIAN_POINT('',(4.34909964308327,0.0349974858299681,3.59949138964752));
#13247=CARTESIAN_POINT('Origin',(4.27445292104672,0.0149959569426778,3.46653399560907));
#13248=CARTESIAN_POINT('Ctrl Pts',(4.4102112066954,0.0513722799480404,11.706973886163));
#13249=CARTESIAN_POINT('Ctrl Pts',(4.50817751566127,0.0776222733209033,
11.6029328940868));
#13250=CARTESIAN_POINT('Ctrl Pts',(4.70981258666106,0.131650227761089,11.3959302972882));
#13251=CARTESIAN_POINT('Ctrl Pts',(5.04656750998174,0.22188343751207,11.1281422470874));
#13252=CARTESIAN_POINT('Ctrl Pts',(5.37607158806058,0.310173789136056,10.9130750253569));
#13253=CARTESIAN_POINT('Ctrl Pts',(5.62759741836264,0.377569932241062,10.7756758097979));
#13254=CARTESIAN_POINT('Ctrl Pts',(5.92870322026153,0.458250988696196,10.6347886165848));
#13255=CARTESIAN_POINT('Ctrl Pts',(6.23443464884433,0.540171478085771,10.5447321686106));
#13256=CARTESIAN_POINT('Ctrl Pts',(6.60142713036405,0.638506817137273,10.4592774903079));
#13257=CARTESIAN_POINT('Ctrl Pts',(6.86887110582377,0.710168214382273,10.3610377706145));
#13258=CARTESIAN_POINT('Ctrl Pts',(7.10758729640882,0.774132024869772,10.2019978237482));
#13259=CARTESIAN_POINT('Ctrl Pts',(7.37469139866462,0.845702353364252,9.92445780127518));
#13260=CARTESIAN_POINT('Ctrl Pts',(7.64695093531355,0.918654076341007,9.5279070047071));
#13261=CARTESIAN_POINT('Ctrl Pts',(7.87171191954179,0.978878600554987,9.09615331026656));
#13262=CARTESIAN_POINT('Ctrl Pts',(7.97590410013386,1.00679681120227,8.72233320794333));
#13263=CARTESIAN_POINT('Ctrl Pts',(8.02445425036305,1.01980578474859,8.33910068047419));
#13264=CARTESIAN_POINT('Ctrl Pts',(8.03003514943051,1.02130118214676,7.84937648135502));
#13265=CARTESIAN_POINT('Ctrl Pts',(8.10334949970651,1.04094570309683,7.36854474797747));
#13266=CARTESIAN_POINT('Ctrl Pts',(8.17397369844545,1.05986940011502,6.98613553279737));
#13267=CARTESIAN_POINT('Ctrl Pts',(8.19086884853079,1.06439644193639,6.74182415651423));
#13268=CARTESIAN_POINT('Ctrl Pts',(8.15926186591506,1.05592737646932,6.54872190268123));
#13269=CARTESIAN_POINT('Ctrl Pts',(8.08863405403125,1.03700271131187,6.36645372110484));
#13270=CARTESIAN_POINT('Ctrl Pts',(7.8697531842168,0.978353759006469,6.10374129848354));
#13271=CARTESIAN_POINT('Ctrl Pts',(7.59271262743873,0.904120965547118,5.95839742644866));
#13272=CARTESIAN_POINT('Ctrl Pts',(7.24661705601864,0.811384936681117,5.80579085268058));
#13273=CARTESIAN_POINT('Ctrl Pts',(6.8046210773698,0.692952471144354,5.63860904148901));
#13274=CARTESIAN_POINT('Ctrl Pts',(6.26783169213932,0.54912018886625,5.39183749253912));
#13275=CARTESIAN_POINT('Ctrl Pts',(5.76242378203297,0.413696547504953,5.13078873237884));
#13276=CARTESIAN_POINT('Ctrl Pts',(5.39028650561027,0.313982664813972,4.92283216185341));
#13277=CARTESIAN_POINT('Ctrl Pts',(5.0354367362137,0.21890095566979,4.68193520114933));
#13278=CARTESIAN_POINT('Ctrl Pts',(4.72268568825884,0.135099564938299,4.38319469956436));
#13279=CARTESIAN_POINT('Ctrl Pts',(4.48560194249773,0.071573166723062,4.01568874810612));
#13280=CARTESIAN_POINT('Ctrl Pts',(4.38680976101687,0.0451018814767583,
3.74027893176065));
#13281=CARTESIAN_POINT('Ctrl Pts',(4.34909964308327,0.0349974858299679,
3.59949138964752));
#13282=CARTESIAN_POINT('Origin',(5.83284639419111,0.84667670172565,8.58));
#13283=CARTESIAN_POINT('',(5.80696448968086,0.943269284354557,10.03));
#13284=CARTESIAN_POINT('Origin',(5.80696448968086,0.943269284354557,8.58));
#13285=CARTESIAN_POINT('Origin',(5.83284639419111,0.84667670172565,10.03));
#13286=CARTESIAN_POINT('Origin',(6.17060215337356,1.04070570267856,7.49483504398303));
#13287=CARTESIAN_POINT('',(4.13385008609474,0.494959631068776,2.88827625586697));
#13288=CARTESIAN_POINT('',(4.12726177229555,0.493194297692335,2.77093943708514));
#13289=CARTESIAN_POINT('Ctrl Pts',(4.13385008609474,0.494959631068776,2.88827625586696));
#13290=CARTESIAN_POINT('Ctrl Pts',(4.13152685057893,0.49433712198849,2.84917441683306));
#13291=CARTESIAN_POINT('Ctrl Pts',(4.1293392907043,0.493750967086684,2.8100639744616));
#13292=CARTESIAN_POINT('Ctrl Pts',(4.1272652896216,0.493195240171477,2.77094676616559));
#13293=CARTESIAN_POINT('',(4.14655803346906,0.498364715305182,3.0837901291539));
#13294=CARTESIAN_POINT('Ctrl Pts',(4.14655803346906,0.498364715305182,3.0837901291539));
#13295=CARTESIAN_POINT('Ctrl Pts',(4.14199767141828,0.497142769976483,3.01864202972875));
#13296=CARTESIAN_POINT('Ctrl Pts',(4.13772368979234,0.495997560051348,2.95347198278946));
#13297=CARTESIAN_POINT('Ctrl Pts',(4.13385008609474,0.494959631068777,2.88827625586697));
#13298=CARTESIAN_POINT('',(4.20352761804101,0.513629669484373,3.61216526483892));
#13299=CARTESIAN_POINT('Ctrl Pts',(4.20352761804101,0.513629669484373,3.61216526483892));
#13300=CARTESIAN_POINT('Ctrl Pts',(4.20348225943688,0.513617515683026,3.61188189200445));
#13301=CARTESIAN_POINT('Ctrl Pts',(4.20343686017451,0.513605350987338,3.61159855052174));
#13302=CARTESIAN_POINT('Ctrl Pts',(4.17554861335302,0.506132717773207,3.43668170480236));
#13303=CARTESIAN_POINT('Ctrl Pts',(4.15891388414094,0.501675455514513,3.26030247161513));
#13304=CARTESIAN_POINT('Ctrl Pts',(4.14655803346906,0.498364715305183,3.0837901291539));
#13305=CARTESIAN_POINT('',(4.20352736956267,0.513629602904919,11.769453644722));
#13306=CARTESIAN_POINT('',(4.20352761804101,0.513629669484373,6.5));
#13307=CARTESIAN_POINT('',(4.24867452199362,0.525724687915784,11.7797317356146));
#13308=CARTESIAN_POINT('Ctrl Pts',(4.24867356681531,0.525726489999986,11.7797315270537));
#13309=CARTESIAN_POINT('Ctrl Pts',(4.24163096531645,0.523839430615753,11.7763983972512));
#13310=CARTESIAN_POINT('Ctrl Pts',(4.23419172931546,0.521846093338737,11.7739226030364));
#13311=CARTESIAN_POINT('Ctrl Pts',(4.21900017669025,0.517775529081036,11.770542186514));
#13312=CARTESIAN_POINT('Ctrl Pts',(4.21127795560258,0.515706366175067,11.7696614596113));
#13313=CARTESIAN_POINT('Ctrl Pts',(4.2035273694791,0.513629602882414,11.7694536480639));
#13314=CARTESIAN_POINT('',(4.33613465287435,0.549161617378652,11.7628168777948));
#13315=CARTESIAN_POINT('Ctrl Pts',(4.33613465287435,0.549161617378653,11.7628168777948));
#13316=CARTESIAN_POINT('Ctrl Pts',(4.32047051975656,0.544964425559608,11.7794523105961));
#13317=CARTESIAN_POINT('Ctrl Pts',(4.28812302309206,0.536296939951185,11.7920460899797));
#13318=CARTESIAN_POINT('Ctrl Pts',(4.25705519011612,0.527972339194697,11.7836561768042));
#13319=CARTESIAN_POINT('Ctrl Pts',(4.24870939485228,0.525736090093557,11.7797108569314));
#13320=CARTESIAN_POINT('',(4.20352761804101,0.513629669484372,3.08701851589662));
#13321=CARTESIAN_POINT('Ctrl Pts',(4.33613465287435,0.549161617378653,11.7628168777948));
#13322=CARTESIAN_POINT('Ctrl Pts',(4.35205479627536,0.55342740694634,11.7459095600555));
#13323=CARTESIAN_POINT('Ctrl Pts',(4.39438451441832,0.564769620738584,11.7010611784437));
#13324=CARTESIAN_POINT('Ctrl Pts',(4.46445801430387,0.583545758443739,11.6277377103039));
#13325=CARTESIAN_POINT('Ctrl Pts',(4.56524008224957,0.610550232161327,11.5268404604711));
#13326=CARTESIAN_POINT('Ctrl Pts',(4.70129424855043,0.647005836148533,11.4029224160728));
#13327=CARTESIAN_POINT('Ctrl Pts',(4.85646075505348,0.688582576258383,11.2768795166233));
#13328=CARTESIAN_POINT('Ctrl Pts',(5.01695088441627,0.731585776814311,11.1598106424589));
#13329=CARTESIAN_POINT('Ctrl Pts',(5.18020418201412,0.775329366067371,11.051370419133));
#13330=CARTESIAN_POINT('Ctrl Pts',(5.34412061714924,0.819250642488016,10.9511663773825));
#13331=CARTESIAN_POINT('Ctrl Pts',(5.50802499472635,0.863168688095727,10.8599381259735));
#13332=CARTESIAN_POINT('Ctrl Pts',(5.67271528816759,0.907297319224552,10.7795199127532));
#13333=CARTESIAN_POINT('Ctrl Pts',(5.8394939294453,0.951985521469674,10.7114411549111));
#13334=CARTESIAN_POINT('Ctrl Pts',(6.00944121138842,0.997522758422198,10.6558377434042));
#13335=CARTESIAN_POINT('Ctrl Pts',(6.18264944336441,1.04393376430259,10.6103475969888));
#13336=CARTESIAN_POINT('Ctrl Pts',(6.35731808181363,1.0907360849181,10.5687216653907));
#13337=CARTESIAN_POINT('Ctrl Pts',(6.53037102597449,1.13710548155383,10.5222908830264));
#13338=CARTESIAN_POINT('Ctrl Pts',(6.69840611695161,1.18213034848124,10.462050267878));
#13339=CARTESIAN_POINT('Ctrl Pts',(6.85846176969156,1.22501713137695,10.3804015453596));
#13340=CARTESIAN_POINT('Ctrl Pts',(7.00901521774594,1.26535780620084,10.2733319413005));
#13341=CARTESIAN_POINT('Ctrl Pts',(7.15038910771078,1.30323882584776,10.1414720974144));
#13342=CARTESIAN_POINT('Ctrl Pts',(7.2837085682718,1.33896166764044,9.98835756998534));
#13343=CARTESIAN_POINT('Ctrl Pts',(7.4100830632121,1.37282361150359,9.81917361987377));
#13344=CARTESIAN_POINT('Ctrl Pts',(7.52979533329094,1.40490041759531,9.63939026966049));
#13345=CARTESIAN_POINT('Ctrl Pts',(7.64125800723788,1.4347667510656,9.45324999450471));
#13346=CARTESIAN_POINT('Ctrl Pts',(7.7408376555659,1.46144903741767,9.26297089919836));
#13347=CARTESIAN_POINT('Ctrl Pts',(7.82441721291024,1.48384411231184,9.06945407017055));
#13348=CARTESIAN_POINT('Ctrl Pts',(7.88861442185322,1.50104570260444,8.87266947141857));
#13349=CARTESIAN_POINT('Ctrl Pts',(7.93207481020654,1.51269087856646,8.67216210283894));
#13350=CARTESIAN_POINT('Ctrl Pts',(7.9568818673599,1.51933790949729,8.46752658699496));
#13351=CARTESIAN_POINT('Ctrl Pts',(7.96947772195623,1.52271295856436,8.25883677791438));
#13352=CARTESIAN_POINT('Ctrl Pts',(7.97819085477051,1.52504763546549,8.04662057355209));
#13353=CARTESIAN_POINT('Ctrl Pts',(7.99115812626861,1.52852220539144,7.8318867323277));
#13354=CARTESIAN_POINT('Ctrl Pts',(8.01405316627263,1.5346569128712,7.61613341658679));
#13355=CARTESIAN_POINT('Ctrl Pts',(8.04799304870936,1.54375107696133,7.40136016279815));
#13356=CARTESIAN_POINT('Ctrl Pts',(8.08710913224301,1.55423219995524,7.19009032473197));
#13357=CARTESIAN_POINT('Ctrl Pts',(8.12102374647152,1.56331959344938,6.98516923427904));
#13358=CARTESIAN_POINT('Ctrl Pts',(8.13767668870611,1.56778173587274,6.78954489191915));
#13359=CARTESIAN_POINT('Ctrl Pts',(8.12605341309117,1.56466728855831,6.60605451948904));
#13360=CARTESIAN_POINT('Ctrl Pts',(8.07889077726024,1.55203009837449,6.43720976255638));
#13361=CARTESIAN_POINT('Ctrl Pts',(7.99556800549189,1.52970382896804,6.28498018271691));
#13362=CARTESIAN_POINT('Ctrl Pts',(7.88027463155873,1.49881106252999,6.15052660592943));
#13363=CARTESIAN_POINT('Ctrl Pts',(7.73984733045563,1.46118368060413,6.03389995867286));
#13364=CARTESIAN_POINT('Ctrl Pts',(7.58187158370519,1.41885420683865,5.93381436957244));
#13365=CARTESIAN_POINT('Ctrl Pts',(7.41231922357235,1.37342278886626,5.84723737025948));
#13366=CARTESIAN_POINT('Ctrl Pts',(7.23512222452275,1.3259429960697,5.76979878895671));
#13367=CARTESIAN_POINT('Ctrl Pts',(7.05278517393707,1.277085930615,5.69662713609756));
#13368=CARTESIAN_POINT('Ctrl Pts',(6.86668148224273,1.22721959671705,5.62308582598972));
#13369=CARTESIAN_POINT('Ctrl Pts',(6.6774713630728,1.17652089808567,5.54547963906641));
#13370=CARTESIAN_POINT('Ctrl Pts',(6.4854907752383,1.12507985461296,5.46195513100458));
#13371=CARTESIAN_POINT('Ctrl Pts',(6.29101491648524,1.07297020531273,5.37226655127806));
#13372=CARTESIAN_POINT('Ctrl Pts',(6.09444768929516,1.02030017552872,5.27709955371581));
#13373=CARTESIAN_POINT('Ctrl Pts',(5.89654491782883,0.967272287734439,5.17752467829117));
#13374=CARTESIAN_POINT('Ctrl Pts',(5.69860439377644,0.914234284165208,5.07442896098936));
#13375=CARTESIAN_POINT('Ctrl Pts',(5.50271582364677,0.861746099992474,4.96787993373722));
#13376=CARTESIAN_POINT('Ctrl Pts',(5.31184140107964,0.810601452609855,4.85676111532844));
#13377=CARTESIAN_POINT('Ctrl Pts',(5.12937361465137,0.761709356591708,4.73929437247794));
#13378=CARTESIAN_POINT('Ctrl Pts',(4.95878680959194,0.716000759936628,4.61340315498245));
#13379=CARTESIAN_POINT('Ctrl Pts',(4.80324392104458,0.674323168561959,4.47714872481864));
#13380=CARTESIAN_POINT('Ctrl Pts',(4.66524062494947,0.637345296820439,4.32911151507775));
#13381=CARTESIAN_POINT('Ctrl Pts',(4.54618516499875,0.60544448247213,4.16885849319143));
#13382=CARTESIAN_POINT('Ctrl Pts',(4.446442617986,0.578718547549039,3.99681013615577));
#13383=CARTESIAN_POINT('Ctrl Pts',(4.3654670825206,0.557021218214407,3.81399668859083));
#13384=CARTESIAN_POINT('Ctrl Pts',(4.30190073863269,0.539988667703842,3.62185203209172));
#13385=CARTESIAN_POINT('Ctrl Pts',(4.25745603462795,0.528079745157933,3.43759550531468));
#13386=CARTESIAN_POINT('Ctrl Pts',(4.23093262286488,0.520972818395501,3.28931577678263));
#13387=CARTESIAN_POINT('Ctrl Pts',(4.21521358817958,0.516760915745777,3.18044435652352));
#13388=CARTESIAN_POINT('Ctrl Pts',(4.20662995714442,0.514460938741779,3.11273802327794));
#13389=CARTESIAN_POINT('Ctrl Pts',(4.20352761804101,0.513629669484372,3.08701851589662));
#13390=CARTESIAN_POINT('',(4.19355650923267,0.510830172248245,2.99707929452952));
#13391=CARTESIAN_POINT('Ctrl Pts',(4.20352761804066,0.51362966948428,3.0870185158938));
#13392=CARTESIAN_POINT('Ctrl Pts',(4.20154142505499,0.513097470677755,3.07055226141507));
#13393=CARTESIAN_POINT('Ctrl Pts',(4.19944545032181,0.512535855940644,3.05259191451735));
#13394=CARTESIAN_POINT('Ctrl Pts',(4.19741839741691,0.51199270875176,3.03459621555749));
#13395=CARTESIAN_POINT('Ctrl Pts',(4.1954566774867,0.511467067480684,3.01656643638677));
#13396=CARTESIAN_POINT('Ctrl Pts',(4.19355679933009,0.510957996662904,2.99850373251447));
#13397=CARTESIAN_POINT('Ctrl Pts',(4.19340242707872,0.510916632742816,2.99703196752542));
#13398=CARTESIAN_POINT('Ctrl Pts',(4.1272652896216,0.493195240171478,2.77094676616559));
#13399=CARTESIAN_POINT('Ctrl Pts',(4.14396588850096,0.49767015215432,2.79475655535354));
#13400=CARTESIAN_POINT('Ctrl Pts',(4.15972316042568,0.501892300390747,2.83474868902384));
#13401=CARTESIAN_POINT('Ctrl Pts',(4.18183336047469,0.507816710638371,2.91779295323766));
#13402=CARTESIAN_POINT('Ctrl Pts',(4.18947454830694,0.509864160797954,2.95856894798348));
#13403=CARTESIAN_POINT('Ctrl Pts',(4.19349145124426,0.510940486696084,2.99676457959157));
#13404=CARTESIAN_POINT('Origin',(-5.91049210772187,0.556898953838929,8.58));
#13405=CARTESIAN_POINT('',(-7.21449197321211,0.906304664727332,8.58));
#13406=CARTESIAN_POINT('',(-5.91049210772187,0.556898953838929,9.93));
#13407=CARTESIAN_POINT('Origin',(-5.91049210772187,0.556898953838929,8.58));
#13408=CARTESIAN_POINT('',(-5.93637401223212,0.460306371210023,10.03));
#13409=CARTESIAN_POINT('Origin',(-5.91049210772187,0.556898953838929,10.03));
#13410=CARTESIAN_POINT('Origin',(-5.93637401223212,0.460306371210023,8.58));
#13411=CARTESIAN_POINT('Origin',(-5.91049210772187,0.556898953838929,8.58));
#13412=CARTESIAN_POINT('Origin',(-5.93637401223212,0.460306371210023,8.58));
#13413=CARTESIAN_POINT('',(-7.13684625968135,1.19608241261405,8.58));
#13414=CARTESIAN_POINT('',(-7.24037387772236,0.809712082098426,8.58));
#13415=CARTESIAN_POINT('',(-5.83284639419111,0.84667670172565,9.93));
#13416=CARTESIAN_POINT('Origin',(-5.83284639419111,0.84667670172565,8.58));
#13417=CARTESIAN_POINT('Origin',(-5.83284639419111,0.84667670172565,8.58));
#13418=CARTESIAN_POINT('Origin',(-6.30001167592471,0.557742789533991,7.49483504398145));
#13419=CARTESIAN_POINT('',(-4.41021120669539,0.0513722799480398,4.08908175574846));
#13420=CARTESIAN_POINT('',(-4.41021120669539,0.0513722799480399,3.79515655425572));
#13421=CARTESIAN_POINT('',(-4.41021120669539,0.0513722799480398,9.69874330802488));
#13422=CARTESIAN_POINT('',(-4.33293714059227,0.0306667563398384,3.94826261099145));
#13423=CARTESIAN_POINT('Ctrl Pts',(-4.33293714059227,0.0306667563398375,
3.94826261099145));
#13424=CARTESIAN_POINT('Ctrl Pts',(-4.33856564926069,0.0321749106921323,
3.95968497399622));
#13425=CARTESIAN_POINT('Ctrl Pts',(-4.34431878377979,0.0337164584404719,
3.97106471407484));
#13426=CARTESIAN_POINT('Ctrl Pts',(-4.35019991655898,0.0352923032192356,
3.98240125579818));
#13427=CARTESIAN_POINT('Ctrl Pts',(-4.36917645914159,0.0403770524793794,
4.01898066572307));
#13428=CARTESIAN_POINT('Ctrl Pts',(-4.3891749803178,0.0457356400783655,
4.05451189417237));
#13429=CARTESIAN_POINT('Ctrl Pts',(-4.41021120669539,0.0513722799480392,
4.08908175574845));
#13430=CARTESIAN_POINT('',(-4.33293714050842,0.0306667563173706,11.7119910933489));
#13431=CARTESIAN_POINT('',(-4.33293714059227,0.0306667563398384,-0.5));
#13432=CARTESIAN_POINT('',(-4.36526624577324,0.039329313965101,11.7547577775405));
#13433=CARTESIAN_POINT('Ctrl Pts',(-4.36526624577325,0.0393293139651038,
11.7547577775405));
#13434=CARTESIAN_POINT('Ctrl Pts',(-4.35509026165876,0.0366026672394349,
11.7400274737341));
#13435=CARTESIAN_POINT('Ctrl Pts',(-4.34410968865593,0.0336604315708949,
11.7259232172676));
#13436=CARTESIAN_POINT('Ctrl Pts',(-4.33293714047413,0.0306667563081824,
11.7119910933921));
#13437=CARTESIAN_POINT('Ctrl Pts',(-4.41021120669539,0.0513722799480397,
3.79515655425571));
#13438=CARTESIAN_POINT('Ctrl Pts',(-4.45903808887791,0.0644554035977742,
3.93047791113146));
#13439=CARTESIAN_POINT('Ctrl Pts',(-4.582867212341,0.0976353172291641,4.19123490599198));
#13440=CARTESIAN_POINT('Ctrl Pts',(-4.94740819214276,0.195313778375095,
4.6367821770228));
#13441=CARTESIAN_POINT('Ctrl Pts',(-5.46260381387957,0.333360029163525,
4.97227704636915));
#13442=CARTESIAN_POINT('Ctrl Pts',(-6.04190293430869,0.488582760658567,
5.27702023853286));
#13443=CARTESIAN_POINT('Ctrl Pts',(-6.54703332936491,0.623932042086293,
5.5237763509783));
#13444=CARTESIAN_POINT('Ctrl Pts',(-7.06475153359634,0.762654216816996,
5.73854350352349));
#13445=CARTESIAN_POINT('Ctrl Pts',(-7.50199905569102,0.879814337254775,
5.90674273368555));
#13446=CARTESIAN_POINT('Ctrl Pts',(-7.78652969114894,0.956054091247638,
6.07256733032961));
#13447=CARTESIAN_POINT('Ctrl Pts',(-7.93300439915508,0.995301870969469,
6.19198615507442));
#13448=CARTESIAN_POINT('Ctrl Pts',(-8.03020970920239,1.02134795529666,6.29626516002264));
#13449=CARTESIAN_POINT('Ctrl Pts',(-8.10816249423483,1.04223534109386,6.41672618659136));
#13450=CARTESIAN_POINT('Ctrl Pts',(-8.17753074630009,1.06082250821511,6.59727787804477));
#13451=CARTESIAN_POINT('Ctrl Pts',(-8.19098371232079,1.06442721959616,6.8408696776684));
#13452=CARTESIAN_POINT('Ctrl Pts',(-8.14971164745181,1.05336840314455,7.12565705017148));
#13453=CARTESIAN_POINT('Ctrl Pts',(-8.09711272128414,1.03927456335518,7.40937238436613));
#13454=CARTESIAN_POINT('Ctrl Pts',(-8.05552374714506,1.02813083132057,7.6951718595586));
#13455=CARTESIAN_POINT('Ctrl Pts',(-8.02521849097772,1.02001056240412,8.07845955750479));
#13456=CARTESIAN_POINT('Ctrl Pts',(-8.01790604838202,1.0180511993159,8.46573709363457));
#13457=CARTESIAN_POINT('Ctrl Pts',(-7.94784659338026,0.999278824926013,
8.84438522402643));
#13458=CARTESIAN_POINT('Ctrl Pts',(-7.81984691825478,0.964981415344694,
9.20903949392042));
#13459=CARTESIAN_POINT('Ctrl Pts',(-7.58470305177623,0.901974806216633,
9.62563358808958));
#13460=CARTESIAN_POINT('Ctrl Pts',(-7.3194406724111,0.830897965883391,9.99304501740382));
#13461=CARTESIAN_POINT('Ctrl Pts',(-7.07733743840935,0.766026599847657,
10.2205558508687));
#13462=CARTESIAN_POINT('Ctrl Pts',(-6.8418306113212,0.702922735717372,10.3784329123269));
#13463=CARTESIAN_POINT('Ctrl Pts',(-6.60664228072597,0.639904212465156,
10.4553494743371));
#13464=CARTESIAN_POINT('Ctrl Pts',(-6.33491900485657,0.567096180131211,
10.5234765064095));
#13465=CARTESIAN_POINT('Ctrl Pts',(-6.06384344546407,0.494461702904175,
10.5898397099152));
#13466=CARTESIAN_POINT('Ctrl Pts',(-5.70632931912773,0.398666081469635,
10.7280695887413));
#13467=CARTESIAN_POINT('Ctrl Pts',(-5.33566097788268,0.29934579877324,10.9374674705902));
#13468=CARTESIAN_POINT('Ctrl Pts',(-4.98550528234724,0.205521862929361,
11.1722294927876));
#13469=CARTESIAN_POINT('Ctrl Pts',(-4.65974554183767,0.118234803533251,
11.442738806744));
#13470=CARTESIAN_POINT('Ctrl Pts',(-4.462637168512,0.0654197740792256,11.6512961064053));
#13471=CARTESIAN_POINT('Ctrl Pts',(-4.36526624577324,0.0393293139651011,
11.7547577775405));
#13472=CARTESIAN_POINT('Origin',(-5.83284639419111,0.84667670172565,8.58));
#13473=CARTESIAN_POINT('',(-5.80696448968086,0.943269284354557,10.03));
#13474=CARTESIAN_POINT('Origin',(-5.80696448968086,0.943269284354557,8.58));
#13475=CARTESIAN_POINT('Origin',(-5.83284639419111,0.84667670172565,10.03));
#13476=CARTESIAN_POINT('Origin',(-6.17060215337345,1.04070570267853,7.49483504398145));
#13477=CARTESIAN_POINT('',(-4.24038550259138,0.523505709884365,3.72695850307423));
#13478=CARTESIAN_POINT('',(-4.20352761804101,0.513629669484373,3.61216526483895));
#13479=CARTESIAN_POINT('Ctrl Pts',(-4.24038388893983,0.523505277507739,
3.72695930646786));
#13480=CARTESIAN_POINT('Ctrl Pts',(-4.22951847389614,0.520593898321352,
3.6959946199449));
#13481=CARTESIAN_POINT('Ctrl Pts',(-4.21930406783922,0.517856956467237,
3.66463907541042));
#13482=CARTESIAN_POINT('Ctrl Pts',(-4.20969621562989,0.515282540226749,
3.63288801911005));
#13483=CARTESIAN_POINT('Ctrl Pts',(-4.20760920009148,0.514723326098641,
3.62599106166146));
#13484=CARTESIAN_POINT('Ctrl Pts',(-4.20555351635821,0.514172507302417,
3.6190845391588));
#13485=CARTESIAN_POINT('Ctrl Pts',(-4.203527618041,0.513629669484373,3.61216526483892));
#13486=CARTESIAN_POINT('',(-4.35319009416574,0.553731609099237,3.76716196298096));
#13487=CARTESIAN_POINT('Ctrl Pts',(-4.35319009416574,0.553731609099236,
3.76716196298096));
#13488=CARTESIAN_POINT('Ctrl Pts',(-4.34602020468552,0.551810443003191,
3.7472909589409));
#13489=CARTESIAN_POINT('Ctrl Pts',(-4.31557469838348,0.543652594176403,
3.71389681896982));
#13490=CARTESIAN_POINT('Ctrl Pts',(-4.26651510466209,0.530507115657757,
3.71290855827619));
#13491=CARTESIAN_POINT('Ctrl Pts',(-4.24417455750459,0.524520984088436,
3.72454107717024));
#13492=CARTESIAN_POINT('Ctrl Pts',(-4.24038711624293,0.523506142260992,
3.7269576996806));
#13493=CARTESIAN_POINT('',(-4.21983606380434,0.517999504581966,11.8857786587691));
#13494=CARTESIAN_POINT('Ctrl Pts',(-4.35319009416574,0.553731609099237,
3.76716196298096));
#13495=CARTESIAN_POINT('Ctrl Pts',(-4.35641988647835,0.55459702934112,3.77611317712024));
#13496=CARTESIAN_POINT('Ctrl Pts',(-4.37357151210268,0.559192793576042,
3.82283506370591));
#13497=CARTESIAN_POINT('Ctrl Pts',(-4.40695017775135,0.56813658008103,3.9061004919638));
#13498=CARTESIAN_POINT('Ctrl Pts',(-4.46167983075915,0.582801346406506,
4.02309317686375));
#13499=CARTESIAN_POINT('Ctrl Pts',(-4.54618516499859,0.605444482472087,
4.16885849319142));
#13500=CARTESIAN_POINT('Ctrl Pts',(-4.66524062494938,0.637345296820415,
4.32911151507774));
#13501=CARTESIAN_POINT('Ctrl Pts',(-4.80324392104458,0.674323168561958,
4.47714872481861));
#13502=CARTESIAN_POINT('Ctrl Pts',(-4.958786809592,0.716000759936643,4.61340315498244));
#13503=CARTESIAN_POINT('Ctrl Pts',(-5.12937361465147,0.761709356591734,
4.73929437247796));
#13504=CARTESIAN_POINT('Ctrl Pts',(-5.31184140107974,0.810601452609883,
4.8567611153285));
#13505=CARTESIAN_POINT('Ctrl Pts',(-5.50271582364683,0.861746099992491,
4.96787993373728));
#13506=CARTESIAN_POINT('Ctrl Pts',(-5.69860439377643,0.914234284165206,
5.07442896098937));
#13507=CARTESIAN_POINT('Ctrl Pts',(-5.89654491782873,0.967272287734412,
5.17752467829109));
#13508=CARTESIAN_POINT('Ctrl Pts',(-6.09444768929498,1.02030017552868,5.27709955371564));
#13509=CARTESIAN_POINT('Ctrl Pts',(-6.29101491648506,1.07297020531268,5.37226655127787));
#13510=CARTESIAN_POINT('Ctrl Pts',(-6.4854907752382,1.12507985461293,5.46195513100446));
#13511=CARTESIAN_POINT('Ctrl Pts',(-6.67747136307279,1.17652089808567,5.54547963906637));
#13512=CARTESIAN_POINT('Ctrl Pts',(-6.86668148224272,1.22721959671704,5.62308582598972));
#13513=CARTESIAN_POINT('Ctrl Pts',(-7.05278517393693,1.27708593061496,5.69662713609756));
#13514=CARTESIAN_POINT('Ctrl Pts',(-7.23512222452253,1.32594299606964,5.76979878895672));
#13515=CARTESIAN_POINT('Ctrl Pts',(-7.4123192235721,1.37342278886619,5.84723737025949));
#13516=CARTESIAN_POINT('Ctrl Pts',(-7.58187158370505,1.41885420683861,5.93381436957244));
#13517=CARTESIAN_POINT('Ctrl Pts',(-7.73984733045567,1.46118368060414,6.03389995867283));
#13518=CARTESIAN_POINT('Ctrl Pts',(-7.88027463155893,1.49881106253004,6.15052660592937));
#13519=CARTESIAN_POINT('Ctrl Pts',(-7.99556800549214,1.5297038289681,6.28498018271686));
#13520=CARTESIAN_POINT('Ctrl Pts',(-8.0788907772604,1.55203009837453,6.43720976255636));
#13521=CARTESIAN_POINT('Ctrl Pts',(-8.12605341309117,1.56466728855831,6.60605451948903));
#13522=CARTESIAN_POINT('Ctrl Pts',(-8.13767668870588,1.56778173587268,6.78954489191904));
#13523=CARTESIAN_POINT('Ctrl Pts',(-8.12102374647115,1.56331959344928,6.9851692342788));
#13524=CARTESIAN_POINT('Ctrl Pts',(-8.08710913224264,1.55423219995514,7.19009032473164));
#13525=CARTESIAN_POINT('Ctrl Pts',(-8.04799304870916,1.54375107696127,7.40136016279791));
#13526=CARTESIAN_POINT('Ctrl Pts',(-8.01405316627267,1.53465691287121,7.61613341658677));
#13527=CARTESIAN_POINT('Ctrl Pts',(-7.99115812626882,1.5285222053915,7.83188673232793));
#13528=CARTESIAN_POINT('Ctrl Pts',(-7.97819085477082,1.52504763546557,8.04662057355248));
#13529=CARTESIAN_POINT('Ctrl Pts',(-7.96947772195652,1.52271295856444,8.25883677791483));
#13530=CARTESIAN_POINT('Ctrl Pts',(-7.95688186736008,1.51933790949734,8.46752658699528));
#13531=CARTESIAN_POINT('Ctrl Pts',(-7.93207481020656,1.51269087856646,8.67216210283896));
#13532=CARTESIAN_POINT('Ctrl Pts',(-7.88861442185311,1.50104570260441,8.87266947141823));
#13533=CARTESIAN_POINT('Ctrl Pts',(-7.82441721291003,1.48384411231178,9.06945407016992));
#13534=CARTESIAN_POINT('Ctrl Pts',(-7.74083765556568,1.46144903741761,9.26297089919765));
#13535=CARTESIAN_POINT('Ctrl Pts',(-7.6412580072377,1.43476675106555,9.4532499945042));
#13536=CARTESIAN_POINT('Ctrl Pts',(-7.52979533329092,1.4049004175953,9.63939026966035));
#13537=CARTESIAN_POINT('Ctrl Pts',(-7.41008306321222,1.37282361150362,9.81917361987397));
#13538=CARTESIAN_POINT('Ctrl Pts',(-7.28370856827199,1.33896166764049,9.98835756998572));
#13539=CARTESIAN_POINT('Ctrl Pts',(-7.15038910771094,1.30323882584781,10.1414720974148));
#13540=CARTESIAN_POINT('Ctrl Pts',(-7.00901521774607,1.26535780620087,10.2733319413008));
#13541=CARTESIAN_POINT('Ctrl Pts',(-6.85846176969162,1.22501713137696,10.3804015453596));
#13542=CARTESIAN_POINT('Ctrl Pts',(-6.69840611695159,1.18213034848123,10.4620502678778));
#13543=CARTESIAN_POINT('Ctrl Pts',(-6.5303710259744,1.13710548155381,10.522290883026));
#13544=CARTESIAN_POINT('Ctrl Pts',(-6.35731808181357,1.09073608491808,10.5687216653902));
#13545=CARTESIAN_POINT('Ctrl Pts',(-6.18264944336438,1.04393376430258,10.6103475969885));
#13546=CARTESIAN_POINT('Ctrl Pts',(-6.00944121138848,0.997522758422214,
10.6558377434043));
#13547=CARTESIAN_POINT('Ctrl Pts',(-5.83949392944539,0.9519855214697,10.7114411549114));
#13548=CARTESIAN_POINT('Ctrl Pts',(-5.67271528816766,0.907297319224571,
10.7795199127535));
#13549=CARTESIAN_POINT('Ctrl Pts',(-5.5080249947264,0.86316868809574,10.8599381259737));
#13550=CARTESIAN_POINT('Ctrl Pts',(-5.34412061714928,0.819250642488025,
10.9511663773826));
#13551=CARTESIAN_POINT('Ctrl Pts',(-5.18020418201415,0.77532936606738,11.0513704191329));
#13552=CARTESIAN_POINT('Ctrl Pts',(-5.01695088441632,0.731585776814323,
11.1598106424589));
#13553=CARTESIAN_POINT('Ctrl Pts',(-4.85646075505354,0.6885825762584,11.2768795166235));
#13554=CARTESIAN_POINT('Ctrl Pts',(-4.70129424855049,0.64700583614855,11.4029224160731));
#13555=CARTESIAN_POINT('Ctrl Pts',(-4.55372957684968,0.607466001534954,
11.5373242211527));
#13556=CARTESIAN_POINT('Ctrl Pts',(-4.42837559321091,0.573877502850922,
11.6641229448127));
#13557=CARTESIAN_POINT('Ctrl Pts',(-4.33577812365105,0.549066085661191,
11.7630935610003));
#13558=CARTESIAN_POINT('Ctrl Pts',(-4.27132531937695,0.531796008806026,
11.8319171323704));
#13559=CARTESIAN_POINT('Ctrl Pts',(-4.23290575435463,0.52150151738474,11.8721941731916));
#13560=CARTESIAN_POINT('Ctrl Pts',(-4.21983606290434,0.517999504115311,
11.8857786577829));
#13561=CARTESIAN_POINT('',(-4.1874280189678,0.50930672791011,11.9066032159468));
#13562=CARTESIAN_POINT('Ctrl Pts',(-4.18742959608618,0.509316217501841,
11.9066111158145));
#13563=CARTESIAN_POINT('Ctrl Pts',(-4.19350514643691,0.510944156311893,
11.90450243125));
#13564=CARTESIAN_POINT('Ctrl Pts',(-4.19934410120603,0.512508699526892,
11.901643125283));
#13565=CARTESIAN_POINT('Ctrl Pts',(-4.21023945601472,0.515428101049129,
11.8946395116115));
#13566=CARTESIAN_POINT('Ctrl Pts',(-4.21530831280245,0.516786297131982,
11.8904852125323));
#13567=CARTESIAN_POINT('Ctrl Pts',(-4.21983606433895,0.517999504499715,
11.8857786592622));
#13568=CARTESIAN_POINT('',(-4.16769131691124,0.504008073901423,11.877637340138));
#13569=CARTESIAN_POINT('Ctrl Pts',(-4.16763707611828,0.504012827760267,
11.8776857726864));
#13570=CARTESIAN_POINT('Ctrl Pts',(-4.17121106796204,0.504970475988557,
11.8820075339236));
#13571=CARTESIAN_POINT('Ctrl Pts',(-4.17467687370206,0.505899135837717,
11.886562635604));
#13572=CARTESIAN_POINT('Ctrl Pts',(-4.18131563754359,0.507677987247797,
11.8961437713168));
#13573=CARTESIAN_POINT('Ctrl Pts',(-4.18453611370009,0.508540911233175,
11.9012960415207));
#13574=CARTESIAN_POINT('Ctrl Pts',(-4.18742622136955,0.509315313249245,
11.9065959606927));
#13575=CARTESIAN_POINT('',(-4.08479144096579,0.481813289987988,11.8776398161281));
#13576=CARTESIAN_POINT('Ctrl Pts',(-4.08479023695801,0.481814084111799,
11.8776392691564));
#13577=CARTESIAN_POINT('Ctrl Pts',(-4.08706116705159,0.482422577996443,
11.8748861572519));
#13578=CARTESIAN_POINT('Ctrl Pts',(-4.08944735162265,0.48306195422525,11.8721644698882));
#13579=CARTESIAN_POINT('Ctrl Pts',(-4.09704796925229,0.485098533581088,
11.8641214958086));
#13580=CARTESIAN_POINT('Ctrl Pts',(-4.10372042299868,0.486886412173969,
11.8578732851267));
#13581=CARTESIAN_POINT('Ctrl Pts',(-4.11372524923515,0.489567197284444,
11.8523156024532));
#13582=CARTESIAN_POINT('Ctrl Pts',(-4.1165662789659,0.490328448906532,11.8510857204423));
#13583=CARTESIAN_POINT('Ctrl Pts',(-4.12093513745218,0.491499081009779,
11.8499489173249));
#13584=CARTESIAN_POINT('Ctrl Pts',(-4.12235572296345,0.491879725750239,
11.8496888852406));
#13585=CARTESIAN_POINT('Ctrl Pts',(-4.12495943119795,0.492577387269001,
11.8494326147479));
#13586=CARTESIAN_POINT('Ctrl Pts',(-4.12612349683335,0.492889297715944,
11.84939639251));
#13587=CARTESIAN_POINT('Ctrl Pts',(-4.12867719428593,0.493573558886076,
11.8494923231472));
#13588=CARTESIAN_POINT('Ctrl Pts',(-4.1300494846765,0.493941262988009,11.849656558201));
#13589=CARTESIAN_POINT('Ctrl Pts',(-4.13413098098875,0.495034896628787,
11.8504660257216));
#13590=CARTESIAN_POINT('Ctrl Pts',(-4.13674238668242,0.495734620675518,
11.8514172338417));
#13591=CARTESIAN_POINT('Ctrl Pts',(-4.14602007144597,0.498220568815541,
11.8559209100288));
#13592=CARTESIAN_POINT('Ctrl Pts',(-4.15225831333328,0.499892100691434,
11.8612576457903));
#13593=CARTESIAN_POINT('Ctrl Pts',(-4.16089398054571,0.502206020747108,
11.8697337781851));
#13594=CARTESIAN_POINT('Ctrl Pts',(-4.16443685648729,0.503155331494539,
11.8736636802312));
#13595=CARTESIAN_POINT('Ctrl Pts',(-4.16770535281746,0.504031122446673,
11.8776253118062));
#13596=CARTESIAN_POINT('',(-4.07626606489887,0.479531832015509,11.8887931799445));
#13597=CARTESIAN_POINT('Ctrl Pts',(-4.07627028629145,0.479531170211144,
11.8887900280456));
#13598=CARTESIAN_POINT('Ctrl Pts',(-4.0776217174446,0.479893285097256,11.8868801280725));
#13599=CARTESIAN_POINT('Ctrl Pts',(-4.07901087220012,0.480265508002298,
11.8849921870643));
#13600=CARTESIAN_POINT('Ctrl Pts',(-4.08185066713631,0.481026428762121,
11.8812787398917));
#13601=CARTESIAN_POINT('Ctrl Pts',(-4.0833083652902,0.481417017795125,11.8794441008497));
#13602=CARTESIAN_POINT('Ctrl Pts',(-4.08479586226042,0.481815591407038,
11.8776442482011));
#13603=CARTESIAN_POINT('',(-4.08038520490284,0.480637587265309,11.8829275774895));
#13604=CARTESIAN_POINT('Ctrl Pts',(-4.08037603631363,0.48063130261391,11.8829200406371));
#13605=CARTESIAN_POINT('Ctrl Pts',(-4.07969798014178,0.480449618010238,
11.8838896584534));
#13606=CARTESIAN_POINT('Ctrl Pts',(-4.07901808066457,0.480267439494496,
11.88485801079));
#13607=CARTESIAN_POINT('Ctrl Pts',(-4.0776425844075,0.479898876383224,11.8868093475648));
#13608=CARTESIAN_POINT('Ctrl Pts',(-4.07694681683877,0.479712446024951,
11.8877924353392));
#13609=CARTESIAN_POINT('Ctrl Pts',(-4.07624931525263,0.479525551038226,
11.8887740875086));
#13610=CARTESIAN_POINT('',(-4.12427480026047,0.492417973766977,11.8128235778692));
#13611=CARTESIAN_POINT('Ctrl Pts',(-4.12423812645742,0.492384114246278,
11.8127998597806));
#13612=CARTESIAN_POINT('Ctrl Pts',(-4.11801102587266,0.490715567673405,
11.8242536640082));
#13613=CARTESIAN_POINT('Ctrl Pts',(-4.11123809259506,0.488900765674664,
11.8357141226374));
#13614=CARTESIAN_POINT('Ctrl Pts',(-4.0966932732167,0.485003493068176,11.8589805842168));
#13615=CARTESIAN_POINT('Ctrl Pts',(-4.08862759438386,0.482842300935126,
11.8711181616458));
#13616=CARTESIAN_POINT('Ctrl Pts',(-4.0803883880346,0.480634612247568,11.8829292871397));
#13617=CARTESIAN_POINT('',(-4.20352761804114,0.513629669484408,11.6617726299258));
#13618=CARTESIAN_POINT('Ctrl Pts',(-4.20352761804102,0.513629669484374,
11.6617726299262));
#13619=CARTESIAN_POINT('Ctrl Pts',(-4.20343490116772,0.51360482607305,11.6619472559298));
#13620=CARTESIAN_POINT('Ctrl Pts',(-4.20334221118164,0.513579989866137,
11.6621218699999));
#13621=CARTESIAN_POINT('Ctrl Pts',(-4.19007529654029,0.510025130801935,
11.687120248245));
#13622=CARTESIAN_POINT('Ctrl Pts',(-4.17722348491259,0.506581497959521,
11.7121079587146));
#13623=CARTESIAN_POINT('Ctrl Pts',(-4.15123059201542,0.499616723298776,
11.7623137554701));
#13624=CARTESIAN_POINT('Ctrl Pts',(-4.13789818430393,0.496044315714815,
11.7879024491707));
#13625=CARTESIAN_POINT('Ctrl Pts',(-4.12430337644551,0.492401597927895,
11.8128379265828));
#13626=CARTESIAN_POINT('',(-4.20352761804101,0.513629669484372,-0.5));
#13627=CARTESIAN_POINT('Ctrl Pts',(-4.4618940931088,0.148042762057828,3.76716196298096));
#13628=CARTESIAN_POINT('Ctrl Pts',(-4.33144929437701,0.63486937850796,3.76716196298096));
#13629=CARTESIAN_POINT('Ctrl Pts',(-4.45472420362858,0.146121595961783,
3.7472909589409));
#13630=CARTESIAN_POINT('Ctrl Pts',(-4.32427940489679,0.632948212411915,
3.7472909589409));
#13631=CARTESIAN_POINT('Ctrl Pts',(-4.42427869732654,0.137963747134995,
3.71389681896982));
#13632=CARTESIAN_POINT('Ctrl Pts',(-4.29383389859475,0.624790363585127,
3.71389681896982));
#13633=CARTESIAN_POINT('Ctrl Pts',(-4.36342914970185,0.121659159989159,
3.71267106042637));
#13634=CARTESIAN_POINT('Ctrl Pts',(-4.23298435097006,0.608485776439291,
3.71267106042637));
#13635=CARTESIAN_POINT('Ctrl Pts',(-4.32167171841416,0.110470289997625,
3.74751057050733));
#13636=CARTESIAN_POINT('Ctrl Pts',(-4.19122691968237,0.597296906447757,
3.74751057050733));
#13637=CARTESIAN_POINT('Ctrl Pts',(-4.31223161698407,0.107940822442964,
3.77924744726674));
#13638=CARTESIAN_POINT('Ctrl Pts',(-4.18178681825228,0.594767438893096,
3.77924744726674));
#13639=CARTESIAN_POINT('Ctrl Pts',(-4.31223161698407,0.107940822442964,
3.79515655425571));
#13640=CARTESIAN_POINT('Ctrl Pts',(-4.18178681825228,0.594767438893096,
3.79515655425571));
#13641=CARTESIAN_POINT('',(-4.2656293489477,0.281862854502613,3.79515655425571));
#13642=CARTESIAN_POINT('Ctrl Pts',(-4.26562934894771,0.281862854502614,
3.79515655425571));
#13643=CARTESIAN_POINT('Ctrl Pts',(-4.26147271281242,0.297375631748062,
3.78450087317412));
#13644=CARTESIAN_POINT('Ctrl Pts',(-4.25740948502131,0.321025382479211,
3.77380857087543));
#13645=CARTESIAN_POINT('Ctrl Pts',(-4.25373528372325,0.35087999479231,3.76392332459328));
#13646=CARTESIAN_POINT('Ctrl Pts',(-4.25264800923526,0.359714610994202,
3.76099806949206));
#13647=CARTESIAN_POINT('Ctrl Pts',(-4.25159449798474,0.36909250201679,3.75814367226683));
#13648=CARTESIAN_POINT('Ctrl Pts',(-4.25058168579739,0.378963405580522,
3.75538231946777));
#13649=CARTESIAN_POINT('Ctrl Pts',(-4.24992566575775,0.385357000195711,
3.75359373240755));
#13650=CARTESIAN_POINT('Ctrl Pts',(-4.24929705290578,0.391856366095762,
3.75187242351791));
#13651=CARTESIAN_POINT('Ctrl Pts',(-4.2486954070829,0.398435948977368,3.75021886318504));
#13652=CARTESIAN_POINT('Ctrl Pts',(-4.24703988692003,0.416540673899359,
3.74566883995297));
#13653=CARTESIAN_POINT('Ctrl Pts',(-4.24559783322402,0.435254084284691,
3.7416155679197));
#13654=CARTESIAN_POINT('Ctrl Pts',(-4.24432835230835,0.454028466761707,
3.73805391289932));
#13655=CARTESIAN_POINT('Ctrl Pts',(-4.24300172172098,0.473648037048853,
3.73433191878866));
#13656=CARTESIAN_POINT('Ctrl Pts',(-4.24186364941875,0.493334218942247,
3.73114657008713));
#13657=CARTESIAN_POINT('Ctrl Pts',(-4.24091335650253,0.512474244136979,
3.72846116461617));
#13658=CARTESIAN_POINT('Ctrl Pts',(-4.24072970279613,0.516173247368188,
3.72794218287957));
#13659=CARTESIAN_POINT('Ctrl Pts',(-4.24055319140698,0.519851886464871,
3.72744179167473));
#13660=CARTESIAN_POINT('Ctrl Pts',(-4.2403839967245,0.523505786600193,3.72695961362351));
#13661=CARTESIAN_POINT('',(-4.31223161698407,0.107940822442964,3.79515655425571));
#13662=CARTESIAN_POINT('',(-4.2656293489477,0.281862854502613,3.79515655425571));
#13663=CARTESIAN_POINT('',(-4.4618940931088,0.148042762057828,3.76716196298096));
#13664=CARTESIAN_POINT('Origin',(-4.38950568308719,0.128646346051165,3.79515655425571));
#13665=CARTESIAN_POINT('',(-4.4618940931088,0.148042762057828,3.76716196298096));
#13666=CARTESIAN_POINT('Origin',(-4.38950568308719,0.128646346051165,9.69874330802488));
#13667=CARTESIAN_POINT('',(-4.31223161698407,0.107940822442963,3.90484829258838));
#13668=CARTESIAN_POINT('Ctrl Pts',(-4.4102112066954,0.0513722799480405,
4.08908175574846));
#13669=CARTESIAN_POINT('Ctrl Pts',(-4.40715780817639,0.0505541242807026,
4.08406395634642));
#13670=CARTESIAN_POINT('Ctrl Pts',(-4.40410949393389,0.0499312335671429,
4.07899808604622));
#13671=CARTESIAN_POINT('Ctrl Pts',(-4.40108550168694,0.0494888587161251,
4.07391511943208));
#13672=CARTESIAN_POINT('Ctrl Pts',(-4.39811787660674,0.0490547297252024,
4.06892689923374));
#13673=CARTESIAN_POINT('Ctrl Pts',(-4.39516354057751,0.048792963118744,
4.06390522474203));
#13674=CARTESIAN_POINT('Ctrl Pts',(-4.39223708843253,0.0486929882427565,
4.05887466023701));
#13675=CARTESIAN_POINT('Ctrl Pts',(-4.38915212776929,0.0485875983219737,
4.05357161995375));
#13676=CARTESIAN_POINT('Ctrl Pts',(-4.38608814252384,0.0486616553190951,
4.04824149366342));
#13677=CARTESIAN_POINT('Ctrl Pts',(-4.38305987368437,0.0489064467463467,
4.04291033102921));
#13678=CARTESIAN_POINT('Ctrl Pts',(-4.37901299723057,0.0492335777626303,
4.03578594489329));
#13679=CARTESIAN_POINT('Ctrl Pts',(-4.37500939219102,0.0498672890372918,
4.02862330711841));
#13680=CARTESIAN_POINT('Ctrl Pts',(-4.37108271550167,0.0507965273914985,
4.02148538683094));
#13681=CARTESIAN_POINT('Ctrl Pts',(-4.36407440648063,0.0524550264368009,
4.0087456694822));
#13682=CARTESIAN_POINT('Ctrl Pts',(-4.35719229690955,0.0550831201777107,
3.99586222022605));
#13683=CARTESIAN_POINT('Ctrl Pts',(-4.35066738468329,0.0587064677477982,
3.98330174291168));
#13684=CARTESIAN_POINT('Ctrl Pts',(-4.3452914594315,0.0616917716143653,
3.97295306927019));
#13685=CARTESIAN_POINT('Ctrl Pts',(-4.33994121668507,0.0654745878228202,
3.96240228466924));
#13686=CARTESIAN_POINT('Ctrl Pts',(-4.33493714468306,0.0701435073148899,
3.95230898650671));
#13687=CARTESIAN_POINT('Ctrl Pts',(-4.33267033431069,0.0722584958938203,
3.9477367915109));
#13688=CARTESIAN_POINT('Ctrl Pts',(-4.33047389394378,0.0745553153476243,
3.9432588379003));
#13689=CARTESIAN_POINT('Ctrl Pts',(-4.32837457659156,0.0770422006884091,
3.93893808366001));
#13690=CARTESIAN_POINT('Ctrl Pts',(-4.32476766398669,0.0813150077859595,
3.931514440486));
#13691=CARTESIAN_POINT('Ctrl Pts',(-4.32123459484289,0.0864133300397851,
3.9241081537622));
#13692=CARTESIAN_POINT('Ctrl Pts',(-4.31820676396266,0.0923632352188068,
3.91767246460418));
#13693=CARTESIAN_POINT('Ctrl Pts',(-4.31592387475179,0.0968492765058371,
3.91282015748251));
#13694=CARTESIAN_POINT('Ctrl Pts',(-4.31380785765501,0.102058212174025,
3.90826444070493));
#13695=CARTESIAN_POINT('Ctrl Pts',(-4.31223161698407,0.107940822442957,
3.90484829258837));
#13696=CARTESIAN_POINT('Origin',(-4.38950568308719,0.128646346051165,3.79515655425572));
#13697=CARTESIAN_POINT('',(-4.31223161698407,0.107940822442964,9.69874330802488));
#13698=CARTESIAN_POINT('Origin',(-4.38950568308719,0.128646346051165,3.79515655425571));
#13699=CARTESIAN_POINT('Origin',(-4.38950568308719,0.128646346051165,3.79515655425571));
#13700=CARTESIAN_POINT('Ctrl Pts',(-4.48256963531681,-0.527769316435443,
3.08701851589457));
#13701=CARTESIAN_POINT('Ctrl Pts',(-3.91894481913026,1.57570713397942,3.08701851589457));
#13702=CARTESIAN_POINT('Ctrl Pts',(-4.48567197442026,-0.526938047178027,
3.11273802327628));
#13703=CARTESIAN_POINT('Ctrl Pts',(-3.92204715823371,1.57653840323684,3.11273802327628));
#13704=CARTESIAN_POINT('Ctrl Pts',(-4.49425560545544,-0.524638070174025,
3.18044435652227));
#13705=CARTESIAN_POINT('Ctrl Pts',(-3.93063078926889,1.57883838024084,3.18044435652227));
#13706=CARTESIAN_POINT('Ctrl Pts',(-4.50997464014073,-0.520426167524303,
3.28931577678178));
#13707=CARTESIAN_POINT('Ctrl Pts',(-3.94634982395418,1.58305028289056,3.28931577678178));
#13708=CARTESIAN_POINT('Ctrl Pts',(-4.53649805190377,-0.51331924076188,
3.43759550531425));
#13709=CARTESIAN_POINT('Ctrl Pts',(-3.97287323571722,1.59015720965299,3.43759550531425));
#13710=CARTESIAN_POINT('Ctrl Pts',(-4.58094275590847,-0.50141031821598,
3.62185203209171));
#13711=CARTESIAN_POINT('Ctrl Pts',(-4.01731793972192,1.60206613219889,3.62185203209171));
#13712=CARTESIAN_POINT('Ctrl Pts',(-4.64450909979627,-0.484377767705444,
3.81399668859083));
#13713=CARTESIAN_POINT('Ctrl Pts',(-4.08088428360972,1.61909868270942,3.81399668859083));
#13714=CARTESIAN_POINT('Ctrl Pts',(-4.72548463526162,-0.462680438370826,
3.99681013615577));
#13715=CARTESIAN_POINT('Ctrl Pts',(-4.16185981907507,1.64079601204404,3.99681013615577));
#13716=CARTESIAN_POINT('Ctrl Pts',(-4.8252271822744,-0.435954503447729,
4.16885849319142));
#13717=CARTESIAN_POINT('Ctrl Pts',(-4.26160236608785,1.66752194696714,4.16885849319142));
#13718=CARTESIAN_POINT('Ctrl Pts',(-4.94428264222518,-0.404053689099401,
4.32911151507774));
#13719=CARTESIAN_POINT('Ctrl Pts',(-4.38065782603863,1.69942276131547,4.32911151507774));
#13720=CARTESIAN_POINT('Ctrl Pts',(-5.08228593832039,-0.367075817357858,
4.47714872481861));
#13721=CARTESIAN_POINT('Ctrl Pts',(-4.51866112213384,1.73640063305701,4.47714872481861));
#13722=CARTESIAN_POINT('Ctrl Pts',(-5.2378288268678,-0.325398225983173,
4.61340315498244));
#13723=CARTESIAN_POINT('Ctrl Pts',(-4.67420401068125,1.77807822443169,4.61340315498244));
#13724=CARTESIAN_POINT('Ctrl Pts',(-5.40841563192727,-0.279689629328082,
4.73929437247796));
#13725=CARTESIAN_POINT('Ctrl Pts',(-4.84479081574072,1.82378682108679,4.73929437247796));
#13726=CARTESIAN_POINT('Ctrl Pts',(-5.59088341835554,-0.230797533309933,
4.8567611153285));
#13727=CARTESIAN_POINT('Ctrl Pts',(-5.02725860216899,1.87267891710493,4.8567611153285));
#13728=CARTESIAN_POINT('Ctrl Pts',(-5.78175784092263,-0.179652885927325,
4.96787993373728));
#13729=CARTESIAN_POINT('Ctrl Pts',(-5.21813302473608,1.92382356448754,4.96787993373728));
#13730=CARTESIAN_POINT('Ctrl Pts',(-5.97764641105224,-0.127164701754609,
5.07442896098937));
#13731=CARTESIAN_POINT('Ctrl Pts',(-5.41402159486569,1.97631174866026,5.07442896098937));
#13732=CARTESIAN_POINT('Ctrl Pts',(-6.17558693510453,-0.0741266981854037,
5.17752467829109));
#13733=CARTESIAN_POINT('Ctrl Pts',(-5.61196211891798,2.02934975222946,5.17752467829109));
#13734=CARTESIAN_POINT('Ctrl Pts',(-6.37348970657079,-0.0210988103911397,
5.27709955371564));
#13735=CARTESIAN_POINT('Ctrl Pts',(-5.80986489038424,2.08237764002373,5.27709955371564));
#13736=CARTESIAN_POINT('Ctrl Pts',(-6.57005693376087,0.0315712193928662,
5.37226655127787));
#13737=CARTESIAN_POINT('Ctrl Pts',(-6.00643211757432,2.13504766980773,5.37226655127787));
#13738=CARTESIAN_POINT('Ctrl Pts',(-6.764532792514,0.0836808686931177,5.46195513100446));
#13739=CARTESIAN_POINT('Ctrl Pts',(-6.20090797632745,2.18715731910799,5.46195513100446));
#13740=CARTESIAN_POINT('Ctrl Pts',(-6.9565133803486,0.135121912165851,5.54547963906637));
#13741=CARTESIAN_POINT('Ctrl Pts',(-6.39288856416205,2.23859836258072,5.54547963906637));
#13742=CARTESIAN_POINT('Ctrl Pts',(-7.14572349951852,0.185820610797228,
5.62308582598972));
#13743=CARTESIAN_POINT('Ctrl Pts',(-6.58209868333197,2.2892970612121,5.62308582598972));
#13744=CARTESIAN_POINT('Ctrl Pts',(-7.33182719121273,0.235686944695142,
5.69662713609756));
#13745=CARTESIAN_POINT('Ctrl Pts',(-6.76820237502618,2.33916339511001,5.69662713609756));
#13746=CARTESIAN_POINT('Ctrl Pts',(-7.51416424179833,0.284544010149827,
5.76979878895672));
#13747=CARTESIAN_POINT('Ctrl Pts',(-6.95053942561178,2.38802046056469,5.76979878895672));
#13748=CARTESIAN_POINT('Ctrl Pts',(-7.69136124084791,0.332023802946379,
5.84723737025949));
#13749=CARTESIAN_POINT('Ctrl Pts',(-7.12773642466136,2.43550025336125,5.84723737025949));
#13750=CARTESIAN_POINT('Ctrl Pts',(-7.86091360098085,0.377455220918793,
5.93381436957244));
#13751=CARTESIAN_POINT('Ctrl Pts',(-7.2972887847943,2.48093167133366,5.93381436957244));
#13752=CARTESIAN_POINT('Ctrl Pts',(-8.01888934773147,0.419784694684325,
6.03389995867283));
#13753=CARTESIAN_POINT('Ctrl Pts',(-7.45526453154492,2.52326114509919,6.03389995867283));
#13754=CARTESIAN_POINT('Ctrl Pts',(-8.15931664883473,0.457412076610226,
6.15052660592937));
#13755=CARTESIAN_POINT('Ctrl Pts',(-7.59569183264818,2.56088852702509,6.15052660592937));
#13756=CARTESIAN_POINT('Ctrl Pts',(-8.27461002276794,0.488304843048287,
6.28498018271686));
#13757=CARTESIAN_POINT('Ctrl Pts',(-7.71098520658139,2.59178129346315,6.28498018271686));
#13758=CARTESIAN_POINT('Ctrl Pts',(-8.35793279453621,0.510631112454717,
6.43720976255636));
#13759=CARTESIAN_POINT('Ctrl Pts',(-7.79430797834966,2.61410756286958,6.43720976255636));
#13760=CARTESIAN_POINT('Ctrl Pts',(-8.40509543036698,0.523268302638496,
6.60605451948903));
#13761=CARTESIAN_POINT('Ctrl Pts',(-7.84147061418043,2.62674475305336,6.60605451948903));
#13762=CARTESIAN_POINT('Ctrl Pts',(-8.41671870598169,0.526382749952862,
6.78954489191904));
#13763=CARTESIAN_POINT('Ctrl Pts',(-7.85309388979514,2.62985920036773,6.78954489191904));
#13764=CARTESIAN_POINT('Ctrl Pts',(-8.40006576374695,0.521920607529461,
6.9851692342788));
#13765=CARTESIAN_POINT('Ctrl Pts',(-7.8364409475604,2.62539705794433,6.9851692342788));
#13766=CARTESIAN_POINT('Ctrl Pts',(-8.36615114951844,0.512833214035319,
7.19009032473164));
#13767=CARTESIAN_POINT('Ctrl Pts',(-7.80252633333189,2.61630966445019,7.19009032473164));
#13768=CARTESIAN_POINT('Ctrl Pts',(-8.32703506598497,0.502352091041457,
7.40136016279791));
#13769=CARTESIAN_POINT('Ctrl Pts',(-7.76341024979842,2.60582854145632,7.40136016279791));
#13770=CARTESIAN_POINT('Ctrl Pts',(-8.29309518354847,0.49325792695139,7.61613341658677));
#13771=CARTESIAN_POINT('Ctrl Pts',(-7.72947036736192,2.59673437736626,7.61613341658677));
#13772=CARTESIAN_POINT('Ctrl Pts',(-8.27020014354463,0.487123219471682,
7.83188673232793));
#13773=CARTESIAN_POINT('Ctrl Pts',(-7.70657532735808,2.59059966988655,7.83188673232793));
#13774=CARTESIAN_POINT('Ctrl Pts',(-8.25723287204663,0.483648649545758,
8.04662057355248));
#13775=CARTESIAN_POINT('Ctrl Pts',(-7.69360805586008,2.58712509996063,8.04662057355248));
#13776=CARTESIAN_POINT('Ctrl Pts',(-8.24851973923233,0.481313972644621,
8.25883677791483));
#13777=CARTESIAN_POINT('Ctrl Pts',(-7.68489492304578,2.58479042305949,8.25883677791483));
#13778=CARTESIAN_POINT('Ctrl Pts',(-8.23592388463589,0.477938923577525,
8.46752658699528));
#13779=CARTESIAN_POINT('Ctrl Pts',(-7.67229906844934,2.58141537399239,8.46752658699528));
#13780=CARTESIAN_POINT('Ctrl Pts',(-8.21111682748236,0.471291892646646,
8.67216210283896));
#13781=CARTESIAN_POINT('Ctrl Pts',(-7.64749201129581,2.57476834306151,8.67216210283896));
#13782=CARTESIAN_POINT('Ctrl Pts',(-8.16765643912891,0.459646716684596,
8.87266947141823));
#13783=CARTESIAN_POINT('Ctrl Pts',(-7.60403162294236,2.56312316709946,8.87266947141823));
#13784=CARTESIAN_POINT('Ctrl Pts',(-8.10345923018583,0.442445126391965,
9.06945407016992));
#13785=CARTESIAN_POINT('Ctrl Pts',(-7.53983441399928,2.54592157680683,9.06945407016992));
#13786=CARTESIAN_POINT('Ctrl Pts',(-8.01987967284149,0.420050051497798,
9.26297089919765));
#13787=CARTESIAN_POINT('Ctrl Pts',(-7.45625485665494,2.52352650191267,9.26297089919765));
#13788=CARTESIAN_POINT('Ctrl Pts',(-7.9203000245135,0.393367765145738,9.4532499945042));
#13789=CARTESIAN_POINT('Ctrl Pts',(-7.35667520832695,2.49684421556061,9.4532499945042));
#13790=CARTESIAN_POINT('Ctrl Pts',(-7.80883735056672,0.363501431675485,
9.63939026966035));
#13791=CARTESIAN_POINT('Ctrl Pts',(-7.24521253438017,2.46697788209035,9.63939026966035));
#13792=CARTESIAN_POINT('Ctrl Pts',(-7.68912508048803,0.331424625583803,
9.81917361987397));
#13793=CARTESIAN_POINT('Ctrl Pts',(-7.12550026430148,2.43490107599867,9.81917361987397));
#13794=CARTESIAN_POINT('Ctrl Pts',(-7.56275058554779,0.297562681720675,
9.98835756998572));
#13795=CARTESIAN_POINT('Ctrl Pts',(-6.99912576936124,2.40103913213554,9.98835756998572));
#13796=CARTESIAN_POINT('Ctrl Pts',(-7.42943112498675,0.26183983992799,10.1414720974148));
#13797=CARTESIAN_POINT('Ctrl Pts',(-6.8658063088002,2.36531629034286,10.1414720974148));
#13798=CARTESIAN_POINT('Ctrl Pts',(-7.28805723502187,0.223958820281056,
10.2733319413008));
#13799=CARTESIAN_POINT('Ctrl Pts',(-6.72443241883532,2.32743527069592,10.2733319413008));
#13800=CARTESIAN_POINT('Ctrl Pts',(-7.13750378696743,0.183618145457146,
10.3804015453596));
#13801=CARTESIAN_POINT('Ctrl Pts',(-6.57387897078088,2.28709459587201,10.3804015453596));
#13802=CARTESIAN_POINT('Ctrl Pts',(-6.97744813422739,0.140731362561417,
10.4620502678778));
#13803=CARTESIAN_POINT('Ctrl Pts',(-6.41382331804084,2.24420781297628,10.4620502678778));
#13804=CARTESIAN_POINT('Ctrl Pts',(-6.8094130432502,0.0957064956339898,
10.522290883026));
#13805=CARTESIAN_POINT('Ctrl Pts',(-6.24578822706365,2.19918294604886,10.522290883026));
#13806=CARTESIAN_POINT('Ctrl Pts',(-6.63636009908937,0.0493370989982661,
10.5687216653902));
#13807=CARTESIAN_POINT('Ctrl Pts',(-6.07273528290282,2.15281354941313,10.5687216653902));
#13808=CARTESIAN_POINT('Ctrl Pts',(-6.46169146064018,0.00253477838276239,
10.6103475969885));
#13809=CARTESIAN_POINT('Ctrl Pts',(-5.89806664445363,2.10601122879763,10.6103475969885));
#13810=CARTESIAN_POINT('Ctrl Pts',(-6.28848322866428,-0.0438762274976022,
10.6558377434043));
#13811=CARTESIAN_POINT('Ctrl Pts',(-5.72485841247773,2.05960022291727,10.6558377434043));
#13812=CARTESIAN_POINT('Ctrl Pts',(-6.1185359467212,-0.0894134644501156,
10.7114411549114));
#13813=CARTESIAN_POINT('Ctrl Pts',(-5.55491113053465,2.01406298596475,10.7114411549114));
#13814=CARTESIAN_POINT('Ctrl Pts',(-5.95175730544346,-0.134101666695245,
10.7795199127535));
#13815=CARTESIAN_POINT('Ctrl Pts',(-5.38813248925691,1.96937478371962,10.7795199127535));
#13816=CARTESIAN_POINT('Ctrl Pts',(-5.7870670120022,-0.178230297824076,
10.8599381259737));
#13817=CARTESIAN_POINT('Ctrl Pts',(-5.22344219581565,1.92524615259079,10.8599381259737));
#13818=CARTESIAN_POINT('Ctrl Pts',(-5.62316263442508,-0.22214834343179,
10.9511663773826));
#13819=CARTESIAN_POINT('Ctrl Pts',(-5.05953781823853,1.88132810698308,10.9511663773826));
#13820=CARTESIAN_POINT('Ctrl Pts',(-5.45924619928996,-0.266069619852436,
11.0513704191329));
#13821=CARTESIAN_POINT('Ctrl Pts',(-4.89562138310341,1.83740683056243,11.0513704191329));
#13822=CARTESIAN_POINT('Ctrl Pts',(-5.29599290169212,-0.309813209105493,
11.1598106424589));
#13823=CARTESIAN_POINT('Ctrl Pts',(-4.73236808550557,1.79366324130937,11.1598106424589));
#13824=CARTESIAN_POINT('Ctrl Pts',(-5.13550277232935,-0.352816409661416,
11.2768795166235));
#13825=CARTESIAN_POINT('Ctrl Pts',(-4.5718779561428,1.75066004075345,11.2768795166235));
#13826=CARTESIAN_POINT('Ctrl Pts',(-4.9803362658263,-0.394393149771265,
11.4029224160731));
#13827=CARTESIAN_POINT('Ctrl Pts',(-4.41671144963975,1.7090833006436,11.4029224160731));
#13828=CARTESIAN_POINT('Ctrl Pts',(-4.83277159412549,-0.433932984384862,
11.5373242211527));
#13829=CARTESIAN_POINT('Ctrl Pts',(-4.26914677793894,1.66954346603001,11.5373242211527));
#13830=CARTESIAN_POINT('Ctrl Pts',(-4.69404542712503,-0.471104548801699,
11.6776492463597));
#13831=CARTESIAN_POINT('Ctrl Pts',(-4.13042061093848,1.63237190161317,11.6776492463597));
#13832=CARTESIAN_POINT('Ctrl Pts',(-4.5634172640769,-0.506106259599206,
11.8183570873721));
#13833=CARTESIAN_POINT('Ctrl Pts',(-3.99979244789035,1.59737019081566,11.8183570873721));
#13834=CARTESIAN_POINT('Ctrl Pts',(-4.438093400719,-0.539686687578305,11.9514202619522));
#13835=CARTESIAN_POINT('Ctrl Pts',(-3.87446858453245,1.56378976283656,11.9514202619522));
#13836=CARTESIAN_POINT('Ctrl Pts',(-4.31385169054842,-0.572977153484772,
12.0684942936867));
#13837=CARTESIAN_POINT('Ctrl Pts',(-3.75022687436187,1.5304992969301,12.0684942936867));
#13838=CARTESIAN_POINT('Ctrl Pts',(-4.18546338657022,-0.607378695853334,
12.1626050652586));
#13839=CARTESIAN_POINT('Ctrl Pts',(-3.62183857038367,1.49609775456153,12.1626050652586));
#13840=CARTESIAN_POINT('Ctrl Pts',(-4.04719835432938,-0.64442669958373,
12.2301117722809));
#13841=CARTESIAN_POINT('Ctrl Pts',(-3.48357353814283,1.45904975083114,12.2301117722809));
#13842=CARTESIAN_POINT('Ctrl Pts',(-3.89329384649782,-0.685665288168704,
12.2723364229645));
#13843=CARTESIAN_POINT('Ctrl Pts',(-3.32966903031127,1.41781116224616,12.2723364229645));
#13844=CARTESIAN_POINT('Ctrl Pts',(-3.71837239798516,-0.732535349036556,
12.2938762651139));
#13845=CARTESIAN_POINT('Ctrl Pts',(-3.15474758179861,1.37094110137831,12.2938762651139));
#13846=CARTESIAN_POINT('Ctrl Pts',(-3.51787595240156,-0.786258209715991,
12.3010487961981));
#13847=CARTESIAN_POINT('Ctrl Pts',(-2.95425113621501,1.31721824069888,12.3010487961981));
#13848=CARTESIAN_POINT('Ctrl Pts',(-3.28845641826505,-0.847730988615793,
12.300400839059));
#13849=CARTESIAN_POINT('Ctrl Pts',(-2.7248316020785,1.25574546179907,12.300400839059));
#13850=CARTESIAN_POINT('Ctrl Pts',(-3.02847742875917,-0.917392148902953,
12.2969132923574));
#13851=CARTESIAN_POINT('Ctrl Pts',(-2.46485261257262,1.18608430151191,12.2969132923574));
#13852=CARTESIAN_POINT('Ctrl Pts',(-2.7380515440356,-0.995211530175729,
12.2935845551224));
#13853=CARTESIAN_POINT('Ctrl Pts',(-2.17442672784905,1.10826492023914,12.2935845551224));
#13854=CARTESIAN_POINT('Ctrl Pts',(-2.41876039944478,-1.08076533451925,
12.2919684497906));
#13855=CARTESIAN_POINT('Ctrl Pts',(-1.85513558325823,1.02271111589562,12.2919684497906));
#13856=CARTESIAN_POINT('Ctrl Pts',(-2.07346909055444,-1.1732858618899,12.2924280531798));
#13857=CARTESIAN_POINT('Ctrl Pts',(-1.50984427436789,0.930190588524968,
12.2924280531798));
#13858=CARTESIAN_POINT('Ctrl Pts',(-1.70610182774042,-1.27172162328655,
12.2945066442122));
#13859=CARTESIAN_POINT('Ctrl Pts',(-1.14247701155387,0.831754827128318,
12.2945066442122));
#13860=CARTESIAN_POINT('Ctrl Pts',(-1.32143431837074,-1.37479297177665,
12.2972483292773));
#13861=CARTESIAN_POINT('Ctrl Pts',(-0.757809502184194,0.728683478638218,
12.2972483292773));
#13862=CARTESIAN_POINT('Ctrl Pts',(-1.00419011146164,-1.45979830082139,
12.299081889758));
#13863=CARTESIAN_POINT('Ctrl Pts',(-0.440565295275094,0.643678149593478,
12.299081889758));
#13864=CARTESIAN_POINT('Ctrl Pts',(-0.763534432174986,-1.52428179574021,
12.2998330708668));
#13865=CARTESIAN_POINT('Ctrl Pts',(-0.19990961598844,0.579194654674658,
12.2998330708668));
#13866=CARTESIAN_POINT('Ctrl Pts',(-0.602693975746076,-1.56737886615059,
12.2999999999989));
#13867=CARTESIAN_POINT('Ctrl Pts',(-0.0390691595595298,0.536097584264278,
12.2999999999989));
#13868=CARTESIAN_POINT('Ctrl Pts',(-0.522273747531633,-1.58892740135578,
12.3));
#13869=CARTESIAN_POINT('Ctrl Pts',(0.0413510686549131,0.514549049059088,
12.3));
#13870=CARTESIAN_POINT('Ctrl Pts',(-0.441853519317205,-1.61047593656096,
12.3000000000011));
#13871=CARTESIAN_POINT('Ctrl Pts',(0.121771296869341,0.493000513853908,
12.3000000000011));
#13872=CARTESIAN_POINT('Ctrl Pts',(-0.281013062888359,-1.65357300697132,
12.2998330708736));
#13873=CARTESIAN_POINT('Ctrl Pts',(0.282611753298187,0.449903443443548,
12.2998330708736));
#13874=CARTESIAN_POINT('Ctrl Pts',(-0.0403573836016633,-1.71805650189016,
12.2990818897713));
#13875=CARTESIAN_POINT('Ctrl Pts',(0.523267432584883,0.385419948524708,
12.2990818897713));
#13876=CARTESIAN_POINT('Ctrl Pts',(0.276886823307267,-1.80306183093486,
12.2972483292974));
#13877=CARTESIAN_POINT('Ctrl Pts',(0.840511639493813,0.300414619480008,
12.2972483292974));
#13878=CARTESIAN_POINT('Ctrl Pts',(0.661554332676866,-1.90613317942493,
12.2945066442369));
#13879=CARTESIAN_POINT('Ctrl Pts',(1.22517914886341,0.197343270989938,12.2945066442369));
#13880=CARTESIAN_POINT('Ctrl Pts',(1.0289215954908,-2.00456894082156,12.2924280532047));
#13881=CARTESIAN_POINT('Ctrl Pts',(1.59254641167735,0.0989075095933076,
12.2924280532047));
#13882=CARTESIAN_POINT('Ctrl Pts',(1.37421290438113,-2.09708946819221,12.291968449812));
#13883=CARTESIAN_POINT('Ctrl Pts',(1.93783772056768,0.00638698222265788,
12.291968449812));
#13884=CARTESIAN_POINT('Ctrl Pts',(1.693504048972,-2.18264327253574,12.2935845551378));
#13885=CARTESIAN_POINT('Ctrl Pts',(2.25712886515855,-0.0791668221208721,
12.2935845551378));
#13886=CARTESIAN_POINT('Ctrl Pts',(1.98392993369567,-2.26046265380854,12.2969132923658));
#13887=CARTESIAN_POINT('Ctrl Pts',(2.54755474988222,-0.156986203393672,
12.2969132923658));
#13888=CARTESIAN_POINT('Ctrl Pts',(2.24390892320168,-2.33012381409574,12.3004008390612));
#13889=CARTESIAN_POINT('Ctrl Pts',(2.80753373938823,-0.226647363680872,
12.3004008390612));
#13890=CARTESIAN_POINT('Ctrl Pts',(2.47332845733829,-2.39159659299556,12.3010487961961));
#13891=CARTESIAN_POINT('Ctrl Pts',(3.03695327352484,-0.288120142580692,
12.3010487961961));
#13892=CARTESIAN_POINT('Ctrl Pts',(2.67382490292192,-2.44531945367501,12.2938762651102));
#13893=CARTESIAN_POINT('Ctrl Pts',(3.23744971910847,-0.341843003260142,
12.2938762651102));
#13894=CARTESIAN_POINT('Ctrl Pts',(2.84874635143459,-2.49218951454286,12.2723364229612));
#13895=CARTESIAN_POINT('Ctrl Pts',(3.41237116762114,-0.388713064127992,
12.2723364229612));
#13896=CARTESIAN_POINT('Ctrl Pts',(3.0026508592661,-2.53342810312782,12.2301117722792));
#13897=CARTESIAN_POINT('Ctrl Pts',(3.56627567545265,-0.429951652712952,
12.2301117722792));
#13898=CARTESIAN_POINT('Ctrl Pts',(3.14091589150692,-2.57047610685821,12.1626050652587));
#13899=CARTESIAN_POINT('Ctrl Pts',(3.70454070769347,-0.466999656443342,
12.1626050652587));
#13900=CARTESIAN_POINT('Ctrl Pts',(3.26930419548512,-2.60487764922678,12.0684942936878));
#13901=CARTESIAN_POINT('Ctrl Pts',(3.83292901167167,-0.501401198811912,
12.0684942936878));
#13902=CARTESIAN_POINT('Ctrl Pts',(3.39354590565573,-2.63816811513325,11.9514202619535));
#13903=CARTESIAN_POINT('Ctrl Pts',(3.95717072184228,-0.534691664718382,
11.9514202619535));
#13904=CARTESIAN_POINT('Ctrl Pts',(3.51886976901364,-2.67174854311235,11.8183570873731));
#13905=CARTESIAN_POINT('Ctrl Pts',(4.08249458520019,-0.568272092697482,
11.8183570873731));
#13906=CARTESIAN_POINT('Ctrl Pts',(3.64949793206175,-2.70675025390985,11.67764924636));
#13907=CARTESIAN_POINT('Ctrl Pts',(4.2131227482483,-0.603273803494982,11.67764924636));
#13908=CARTESIAN_POINT('Ctrl Pts',(3.78822409906218,-2.74392181832668,11.5373242211525));
#13909=CARTESIAN_POINT('Ctrl Pts',(4.35184891524873,-0.640445367911812,
11.5373242211525));
#13910=CARTESIAN_POINT('Ctrl Pts',(3.93578877076297,-2.78346165294027,11.4029224160728));
#13911=CARTESIAN_POINT('Ctrl Pts',(4.49941358694952,-0.679985202525402,
11.4029224160728));
#13912=CARTESIAN_POINT('Ctrl Pts',(4.09095527726601,-2.82503839305012,11.2768795166233));
#13913=CARTESIAN_POINT('Ctrl Pts',(4.65458009345256,-0.721561942635252,
11.2768795166233));
#13914=CARTESIAN_POINT('Ctrl Pts',(4.25144540662881,-2.86804159360605,11.1598106424589));
#13915=CARTESIAN_POINT('Ctrl Pts',(4.81507022281536,-0.764565143191182,
11.1598106424589));
#13916=CARTESIAN_POINT('Ctrl Pts',(4.41469870422666,-2.91178518285911,11.051370419133));
#13917=CARTESIAN_POINT('Ctrl Pts',(4.97832352041321,-0.808308732444242,
11.051370419133));
#13918=CARTESIAN_POINT('Ctrl Pts',(4.57861513936178,-2.95570645927976,10.9511663773825));
#13919=CARTESIAN_POINT('Ctrl Pts',(5.14223995554833,-0.852230008864892,
10.9511663773825));
#13920=CARTESIAN_POINT('Ctrl Pts',(4.74251951693888,-2.99962450488747,10.8599381259735));
#13921=CARTESIAN_POINT('Ctrl Pts',(5.30614433312543,-0.896148054472602,
10.8599381259735));
#13922=CARTESIAN_POINT('Ctrl Pts',(4.90720981038013,-3.04375313601629,10.7795199127532));
#13923=CARTESIAN_POINT('Ctrl Pts',(5.47083462656668,-0.940276685601422,
10.7795199127532));
#13924=CARTESIAN_POINT('Ctrl Pts',(5.07398845165783,-3.08844133826141,10.7114411549111));
#13925=CARTESIAN_POINT('Ctrl Pts',(5.63761326784438,-0.984964887846542,
10.7114411549111));
#13926=CARTESIAN_POINT('Ctrl Pts',(5.24393573360096,-3.13397857521394,10.6558377434042));
#13927=CARTESIAN_POINT('Ctrl Pts',(5.80756054978751,-1.03050212479907,10.6558377434042));
#13928=CARTESIAN_POINT('Ctrl Pts',(5.41714396557695,-3.18038958109433,10.6103475969888));
#13929=CARTESIAN_POINT('Ctrl Pts',(5.9807687817635,-1.07691313067946,10.6103475969888));
#13930=CARTESIAN_POINT('Ctrl Pts',(5.59181260402617,-3.22719190170984,10.5687216653907));
#13931=CARTESIAN_POINT('Ctrl Pts',(6.15543742021272,-1.12371545129497,10.5687216653907));
#13932=CARTESIAN_POINT('Ctrl Pts',(5.76486554818703,-3.27356129834557,10.5222908830264));
#13933=CARTESIAN_POINT('Ctrl Pts',(6.32849036437358,-1.1700848479307,10.5222908830264));
#13934=CARTESIAN_POINT('Ctrl Pts',(5.93290063916415,-3.31858616527298,10.462050267878));
#13935=CARTESIAN_POINT('Ctrl Pts',(6.4965254553507,-1.21510971485811,10.462050267878));
#13936=CARTESIAN_POINT('Ctrl Pts',(6.0929562919041,-3.36147294816869,10.3804015453596));
#13937=CARTESIAN_POINT('Ctrl Pts',(6.65658110809065,-1.25799649775382,10.3804015453596));
#13938=CARTESIAN_POINT('Ctrl Pts',(6.24350973995848,-3.40181362299258,10.2733319413005));
#13939=CARTESIAN_POINT('Ctrl Pts',(6.80713455614503,-1.29833717257771,10.2733319413005));
#13940=CARTESIAN_POINT('Ctrl Pts',(6.38488362992331,-3.4396946426395,10.1414720974144));
#13941=CARTESIAN_POINT('Ctrl Pts',(6.94850844610986,-1.33621819222463,10.1414720974144));
#13942=CARTESIAN_POINT('Ctrl Pts',(6.51820309048434,-3.47541748443218,9.98835756998534));
#13943=CARTESIAN_POINT('Ctrl Pts',(7.08182790667089,-1.37194103401731,9.98835756998534));
#13944=CARTESIAN_POINT('Ctrl Pts',(6.64457758542464,-3.50927942829533,9.81917361987377));
#13945=CARTESIAN_POINT('Ctrl Pts',(7.20820240161119,-1.40580297788046,9.81917361987377));
#13946=CARTESIAN_POINT('Ctrl Pts',(6.76428985550348,-3.54135623438705,9.63939026966049));
#13947=CARTESIAN_POINT('Ctrl Pts',(7.32791467169003,-1.43787978397218,9.63939026966049));
#13948=CARTESIAN_POINT('Ctrl Pts',(6.87575252945042,-3.57122256785734,9.45324999450471));
#13949=CARTESIAN_POINT('Ctrl Pts',(7.43937734563697,-1.46774611744247,9.45324999450471));
#13950=CARTESIAN_POINT('Ctrl Pts',(6.97533217777844,-3.59790485420941,9.26297089919836));
#13951=CARTESIAN_POINT('Ctrl Pts',(7.53895699396499,-1.49442840379454,9.26297089919836));
#13952=CARTESIAN_POINT('Ctrl Pts',(7.05891173512278,-3.62029992910358,9.06945407017055));
#13953=CARTESIAN_POINT('Ctrl Pts',(7.62253655130933,-1.51682347868871,9.06945407017055));
#13954=CARTESIAN_POINT('Ctrl Pts',(7.12310894406576,-3.63750151939618,8.87266947141857));
#13955=CARTESIAN_POINT('Ctrl Pts',(7.68673376025231,-1.53402506898131,8.87266947141857));
#13956=CARTESIAN_POINT('Ctrl Pts',(7.16656933241908,-3.6491466953582,8.67216210283894));
#13957=CARTESIAN_POINT('Ctrl Pts',(7.73019414860563,-1.54567024494333,8.67216210283894));
#13958=CARTESIAN_POINT('Ctrl Pts',(7.19137638957244,-3.65579372628903,8.46752658699496));
#13959=CARTESIAN_POINT('Ctrl Pts',(7.75500120575899,-1.55231727587416,8.46752658699496));
#13960=CARTESIAN_POINT('Ctrl Pts',(7.20397224416876,-3.6591687753561,8.25883677791438));
#13961=CARTESIAN_POINT('Ctrl Pts',(7.76759706035531,-1.55569232494123,8.25883677791438));
#13962=CARTESIAN_POINT('Ctrl Pts',(7.21268537698305,-3.66150345225723,8.04662057355209));
#13963=CARTESIAN_POINT('Ctrl Pts',(7.7763101931696,-1.55802700184236,8.04662057355209));
#13964=CARTESIAN_POINT('Ctrl Pts',(7.22565264848115,-3.66497802218318,7.8318867323277));
#13965=CARTESIAN_POINT('Ctrl Pts',(7.7892774646677,-1.56150157176831,7.8318867323277));
#13966=CARTESIAN_POINT('Ctrl Pts',(7.24854768848517,-3.67111272966294,7.61613341658679));
#13967=CARTESIAN_POINT('Ctrl Pts',(7.81217250467172,-1.56763627924807,7.61613341658679));
#13968=CARTESIAN_POINT('Ctrl Pts',(7.2824875709219,-3.68020689375307,7.40136016279815));
#13969=CARTESIAN_POINT('Ctrl Pts',(7.84611238710845,-1.5767304433382,7.40136016279815));
#13970=CARTESIAN_POINT('Ctrl Pts',(7.32160365445555,-3.69068801674698,7.19009032473197));
#13971=CARTESIAN_POINT('Ctrl Pts',(7.8852284706421,-1.58721156633211,7.19009032473197));
#13972=CARTESIAN_POINT('Ctrl Pts',(7.35551826868406,-3.69977541024112,6.98516923427904));
#13973=CARTESIAN_POINT('Ctrl Pts',(7.91914308487061,-1.59629895982625,6.98516923427904));
#13974=CARTESIAN_POINT('Ctrl Pts',(7.37217121091865,-3.70423755266448,6.78954489191915));
#13975=CARTESIAN_POINT('Ctrl Pts',(7.9357960271052,-1.60076110224961,6.78954489191915));
#13976=CARTESIAN_POINT('Ctrl Pts',(7.36054793530371,-3.70112310535005,6.60605451948904));
#13977=CARTESIAN_POINT('Ctrl Pts',(7.92417275149026,-1.59764665493518,6.60605451948904));
#13978=CARTESIAN_POINT('Ctrl Pts',(7.31338529947278,-3.68848591516623,6.43720976255638));
#13979=CARTESIAN_POINT('Ctrl Pts',(7.87701011565933,-1.58500946475136,6.43720976255638));
#13980=CARTESIAN_POINT('Ctrl Pts',(7.23006252770443,-3.66615964575978,6.28498018271691));
#13981=CARTESIAN_POINT('Ctrl Pts',(7.79368734389098,-1.56268319534491,6.28498018271691));
#13982=CARTESIAN_POINT('Ctrl Pts',(7.11476915377127,-3.63526687932173,6.15052660592943));
#13983=CARTESIAN_POINT('Ctrl Pts',(7.67839396995782,-1.53179042890686,6.15052660592943));
#13984=CARTESIAN_POINT('Ctrl Pts',(6.97434185266817,-3.59763949739587,6.03389995867286));
#13985=CARTESIAN_POINT('Ctrl Pts',(7.53796666885472,-1.494163046981,6.03389995867286));
#13986=CARTESIAN_POINT('Ctrl Pts',(6.81636610591773,-3.55531002363039,5.93381436957244));
#13987=CARTESIAN_POINT('Ctrl Pts',(7.37999092210428,-1.45183357321552,5.93381436957244));
#13988=CARTESIAN_POINT('Ctrl Pts',(6.64681374578489,-3.509878605658,5.84723737025948));
#13989=CARTESIAN_POINT('Ctrl Pts',(7.21043856197144,-1.40640215524313,5.84723737025948));
#13990=CARTESIAN_POINT('Ctrl Pts',(6.46961674673529,-3.46239881286144,5.76979878895671));
#13991=CARTESIAN_POINT('Ctrl Pts',(7.03324156292184,-1.35892236244657,5.76979878895671));
#13992=CARTESIAN_POINT('Ctrl Pts',(6.28727969614961,-3.41354174740674,5.69662713609756));
#13993=CARTESIAN_POINT('Ctrl Pts',(6.85090451233616,-1.31006529699187,5.69662713609756));
#13994=CARTESIAN_POINT('Ctrl Pts',(6.10117600445527,-3.36367541350879,5.62308582598972));
#13995=CARTESIAN_POINT('Ctrl Pts',(6.66480082064182,-1.26019896309392,5.62308582598972));
#13996=CARTESIAN_POINT('Ctrl Pts',(5.91196588528534,-3.31297671487741,5.54547963906641));
#13997=CARTESIAN_POINT('Ctrl Pts',(6.47559070147189,-1.20950026446254,5.54547963906641));
#13998=CARTESIAN_POINT('Ctrl Pts',(5.71998529745084,-3.2615356714047,5.46195513100458));
#13999=CARTESIAN_POINT('Ctrl Pts',(6.28361011363739,-1.15805922098983,5.46195513100458));
#14000=CARTESIAN_POINT('Ctrl Pts',(5.52550943869778,-3.20942602210447,5.37226655127806));
#14001=CARTESIAN_POINT('Ctrl Pts',(6.08913425488433,-1.1059495716896,5.37226655127806));
#14002=CARTESIAN_POINT('Ctrl Pts',(5.3289422115077,-3.15675599232046,5.27709955371581));
#14003=CARTESIAN_POINT('Ctrl Pts',(5.89256702769425,-1.05327954190559,5.27709955371581));
#14004=CARTESIAN_POINT('Ctrl Pts',(5.13103944004137,-3.10372810452618,5.17752467829117));
#14005=CARTESIAN_POINT('Ctrl Pts',(5.69466425622792,-1.00025165411131,5.17752467829117));
#14006=CARTESIAN_POINT('Ctrl Pts',(4.93309891598898,-3.05069010095695,5.07442896098936));
#14007=CARTESIAN_POINT('Ctrl Pts',(5.49672373217553,-0.947213650542082,
5.07442896098936));
#14008=CARTESIAN_POINT('Ctrl Pts',(4.7372103458593,-2.99820191678422,4.96787993373722));
#14009=CARTESIAN_POINT('Ctrl Pts',(5.30083516204585,-0.894725466369352,
4.96787993373722));
#14010=CARTESIAN_POINT('Ctrl Pts',(4.54633592329218,-2.9470572694016,4.85676111532844));
#14011=CARTESIAN_POINT('Ctrl Pts',(5.10996073947873,-0.843580818986732,
4.85676111532844));
#14012=CARTESIAN_POINT('Ctrl Pts',(4.36386813686391,-2.89816517338345,4.73929437247794));
#14013=CARTESIAN_POINT('Ctrl Pts',(4.92749295305046,-0.794688722968582,
4.73929437247794));
#14014=CARTESIAN_POINT('Ctrl Pts',(4.19328133180448,-2.85245657672837,4.61340315498245));
#14015=CARTESIAN_POINT('Ctrl Pts',(4.75690614799103,-0.748980126313502,
4.61340315498245));
#14016=CARTESIAN_POINT('Ctrl Pts',(4.03773844325712,-2.8107789853537,4.47714872481864));
#14017=CARTESIAN_POINT('Ctrl Pts',(4.60136325944367,-0.707302534938832,
4.47714872481864));
#14018=CARTESIAN_POINT('Ctrl Pts',(3.899735147162,-2.77380111361218,4.32911151507775));
#14019=CARTESIAN_POINT('Ctrl Pts',(4.46335996334855,-0.670324663197312,
4.32911151507775));
#14020=CARTESIAN_POINT('Ctrl Pts',(3.78067968721129,-2.74190029926387,4.16885849319143));
#14021=CARTESIAN_POINT('Ctrl Pts',(4.34430450339784,-0.638423848849002,
4.16885849319143));
#14022=CARTESIAN_POINT('Ctrl Pts',(3.68093714019854,-2.71517436434078,3.99681013615577));
#14023=CARTESIAN_POINT('Ctrl Pts',(4.24456195638509,-0.611697913925912,
3.99681013615577));
#14024=CARTESIAN_POINT('Ctrl Pts',(3.59996160473314,-2.69347703500615,3.81399668859083));
#14025=CARTESIAN_POINT('Ctrl Pts',(4.16358642091969,-0.590000584591282,
3.81399668859083));
#14026=CARTESIAN_POINT('Ctrl Pts',(3.53639526084523,-2.67644448449558,3.62185203209172));
#14027=CARTESIAN_POINT('Ctrl Pts',(4.10002007703178,-0.572968034080712,
3.62185203209172));
#14028=CARTESIAN_POINT('Ctrl Pts',(3.48818717006887,-2.66352716550341,3.42199345348454));
#14029=CARTESIAN_POINT('Ctrl Pts',(4.05181198625542,-0.560050715088542,
3.42199345348454));
#14030=CARTESIAN_POINT('Ctrl Pts',(3.45268796832176,-2.65401518306332,3.21600287470933));
#14031=CARTESIAN_POINT('Ctrl Pts',(4.01631278450831,-0.550538732648452,
3.21600287470933));
#14032=CARTESIAN_POINT('Ctrl Pts',(3.42695681706767,-2.64712054186447,3.00529120729351));
#14033=CARTESIAN_POINT('Ctrl Pts',(3.99058163325422,-0.543644091449602,
3.00529120729351));
#14034=CARTESIAN_POINT('Ctrl Pts',(3.40807807946881,-2.64206199937073,2.7909834104826));
#14035=CARTESIAN_POINT('Ctrl Pts',(3.97170289565536,-0.538585548955862,
2.7909834104826));
#14036=CARTESIAN_POINT('Ctrl Pts',(3.39349547439656,-2.63815460211808,2.57377631141663));
#14037=CARTESIAN_POINT('Ctrl Pts',(3.95712029058311,-0.534678151703212,
2.57377631141663));
#14038=CARTESIAN_POINT('Ctrl Pts',(3.3812915164225,-2.63488456143447,2.35385258470204));
#14039=CARTESIAN_POINT('Ctrl Pts',(3.94491633260905,-0.531408111019602,
2.35385258470204));
#14040=CARTESIAN_POINT('Ctrl Pts',(3.37061031638295,-2.63202254250968,2.13065748555701));
#14041=CARTESIAN_POINT('Ctrl Pts',(3.9342351325695,-0.528546092094812,2.13065748555701));
#14042=CARTESIAN_POINT('Ctrl Pts',(3.36139243871498,-2.62955261963262,1.9033255681334));
#14043=CARTESIAN_POINT('Ctrl Pts',(3.92501725490153,-0.526076169217752,
1.9033255681334));
#14044=CARTESIAN_POINT('Ctrl Pts',(3.35377640719761,-2.62751191013801,1.67142113207676));
#14045=CARTESIAN_POINT('Ctrl Pts',(3.91740122338416,-0.524035459723142,
1.67142113207676));
#14046=CARTESIAN_POINT('Ctrl Pts',(3.34760493989187,-2.62585827045732,1.4355810193293));
#14047=CARTESIAN_POINT('Ctrl Pts',(3.91122975607842,-0.522381820042452,
1.4355810193293));
#14048=CARTESIAN_POINT('Ctrl Pts',(3.34188856653398,-2.62432657283244,1.19819542279832));
#14049=CARTESIAN_POINT('Ctrl Pts',(3.90551338272053,-0.520850122417572,
1.19819542279832));
#14050=CARTESIAN_POINT('Ctrl Pts',(3.33428532937914,-2.62228929157694,0.964078729991153));
#14051=CARTESIAN_POINT('Ctrl Pts',(3.89791014556569,-0.518812841162072,
0.964078729991153));
#14052=CARTESIAN_POINT('Ctrl Pts',(3.32057911187183,-2.61861672166457,0.741129277895168));
#14053=CARTESIAN_POINT('Ctrl Pts',(3.88420392805838,-0.515140271249702,
0.741129277895168));
#14054=CARTESIAN_POINT('Ctrl Pts',(3.29563694769388,-2.6119334889156,0.538436816836329));
#14055=CARTESIAN_POINT('Ctrl Pts',(3.85926176388043,-0.508457038500732,
0.538436816836329));
#14056=CARTESIAN_POINT('Ctrl Pts',(3.25436653279393,-2.60087511457186,0.364350357241537));
#14057=CARTESIAN_POINT('Ctrl Pts',(3.81799134898048,-0.497398664156992,
0.364350357241537));
#14058=CARTESIAN_POINT('Ctrl Pts',(3.19265967747922,-2.58434081252282,0.224659532804428));
#14059=CARTESIAN_POINT('Ctrl Pts',(3.75628449366577,-0.480864362107952,
0.224659532804428));
#14060=CARTESIAN_POINT('Ctrl Pts',(3.10837404726043,-2.56175654597215,0.120497232333236));
#14061=CARTESIAN_POINT('Ctrl Pts',(3.67199886344698,-0.458280095557282,
0.120497232333236));
#14062=CARTESIAN_POINT('Ctrl Pts',(3.00221227044612,-2.5333105836077,0.0470540298718229));
#14063=CARTESIAN_POINT('Ctrl Pts',(3.56583708663267,-0.429834133192832,
0.0470540298718229));
#14064=CARTESIAN_POINT('Ctrl Pts',(2.87822299923539,-2.50008775851666,-0.00118366394786523));
#14065=CARTESIAN_POINT('Ctrl Pts',(3.44184781542194,-0.396611308101792,
-0.00118366394786523));
#14066=CARTESIAN_POINT('Ctrl Pts',(2.74414641495931,-2.46416204603596,-0.0263068037111615));
#14067=CARTESIAN_POINT('Ctrl Pts',(3.30777123114586,-0.360685595621092,
-0.0263068037111615));
#14068=CARTESIAN_POINT('Ctrl Pts',(2.61226182052933,-2.42882367546434,-0.0214179570895094));
#14069=CARTESIAN_POINT('Ctrl Pts',(3.17588663671588,-0.325347225049472,
-0.0214179570895094));
#14070=CARTESIAN_POINT('Ctrl Pts',(2.49578790483729,-2.39761458381537,0.0241851999814078));
#14071=CARTESIAN_POINT('Ctrl Pts',(3.05941272102384,-0.294138133400502,
0.0241851999814078));
#14072=CARTESIAN_POINT('Ctrl Pts',(2.40509129270346,-2.37331249983787,0.119017371327004));
#14073=CARTESIAN_POINT('Ctrl Pts',(2.96871610889001,-0.269836049423002,
0.119017371327004));
#14074=CARTESIAN_POINT('Ctrl Pts',(2.34304142033346,-2.35668628664588,0.262319630540593));
#14075=CARTESIAN_POINT('Ctrl Pts',(2.90666623652001,-0.253209836231012,
0.262319630540593));
#14076=CARTESIAN_POINT('Ctrl Pts',(2.3057679034264,-2.34669887789156,0.444963858672424));
#14077=CARTESIAN_POINT('Ctrl Pts',(2.86939271961295,-0.243222427476692,
0.444963858672424));
#14078=CARTESIAN_POINT('Ctrl Pts',(2.28584564406426,-2.34136072458407,0.65402023086958));
#14079=CARTESIAN_POINT('Ctrl Pts',(2.84947046025081,-0.237884274169202,
0.65402023086958));
#14080=CARTESIAN_POINT('Ctrl Pts',(2.27453624485986,-2.33833038020037,0.875890304828918));
#14081=CARTESIAN_POINT('Ctrl Pts',(2.83816106104641,-0.234853929785502,
0.875890304828918));
#14082=CARTESIAN_POINT('Ctrl Pts',(2.26478646139362,-2.33571793359422,1.10060381648398));
#14083=CARTESIAN_POINT('Ctrl Pts',(2.82841127758017,-0.232241483179352,
1.10060381648398));
#14084=CARTESIAN_POINT('Ctrl Pts',(2.25268204108937,-2.33247456394885,1.32371934078733));
#14085=CARTESIAN_POINT('Ctrl Pts',(2.81630685727592,-0.228998113533982,
1.32371934078733));
#14086=CARTESIAN_POINT('Ctrl Pts',(2.23620043629654,-2.32805833125464,1.54401727992264));
#14087=CARTESIAN_POINT('Ctrl Pts',(2.79982525248309,-0.224581880839772,
1.54401727992264));
#14088=CARTESIAN_POINT('Ctrl Pts',(2.21453882104101,-2.32225411894016,1.76209503442146));
#14089=CARTESIAN_POINT('Ctrl Pts',(2.77816363722756,-0.218777668525292,
1.76209503442146));
#14090=CARTESIAN_POINT('Ctrl Pts',(2.187197906392,-2.31492814293964,1.97856787413951));
#14091=CARTESIAN_POINT('Ctrl Pts',(2.75082272257855,-0.211451692524772,
1.97856787413951));
#14092=CARTESIAN_POINT('Ctrl Pts',(2.15320467528109,-2.30581968411534,2.19251877196071));
#14093=CARTESIAN_POINT('Ctrl Pts',(2.71682949146764,-0.202343233700472,
2.19251877196071));
#14094=CARTESIAN_POINT('Ctrl Pts',(2.11018279685234,-2.29429200653349,2.39962532458029));
#14095=CARTESIAN_POINT('Ctrl Pts',(2.67380761303889,-0.190815556118622,
2.39962532458029));
#14096=CARTESIAN_POINT('Ctrl Pts',(2.05479350671064,-2.27945049097069,2.59347738935741));
#14097=CARTESIAN_POINT('Ctrl Pts',(2.61841832289719,-0.175974040555822,
2.59347738935741));
#14098=CARTESIAN_POINT('Ctrl Pts',(1.98331409228925,-2.26029763960102,2.7672283971178));
#14099=CARTESIAN_POINT('Ctrl Pts',(2.5469389084758,-0.156821189186152,2.7672283971178));
#14100=CARTESIAN_POINT('Ctrl Pts',(1.89216285547678,-2.23587373930803,2.91510580081997));
#14101=CARTESIAN_POINT('Ctrl Pts',(2.45578767166333,-0.132397288893162,
2.91510580081997));
#14102=CARTESIAN_POINT('Ctrl Pts',(1.77845779245372,-2.20540655949567,3.03403241435618));
#14103=CARTESIAN_POINT('Ctrl Pts',(2.34208260864027,-0.101930109080802,
3.03403241435618));
#14104=CARTESIAN_POINT('Ctrl Pts',(1.64052927563717,-2.16844872480145,3.12505646843308));
#14105=CARTESIAN_POINT('Ctrl Pts',(2.20415409182372,-0.0649722743865824,
3.12505646843308));
#14106=CARTESIAN_POINT('Ctrl Pts',(1.477782460992,-2.12484084724654,3.19196918412265));
#14107=CARTESIAN_POINT('Ctrl Pts',(2.04140727717855,-0.0213643968316721,
3.19196918412265));
#14108=CARTESIAN_POINT('Ctrl Pts',(1.29059023976394,-2.07468284273909,3.24001322621211));
#14109=CARTESIAN_POINT('Ctrl Pts',(1.85421505595049,0.0287936076757775,
3.24001322621211));
#14110=CARTESIAN_POINT('Ctrl Pts',(1.08017544120182,-2.01830236738882,3.27464765209773));
#14111=CARTESIAN_POINT('Ctrl Pts',(1.64380025738837,0.0851740830260477,
3.27464765209773));
#14112=CARTESIAN_POINT('Ctrl Pts',(0.84849626609417,-1.95622411951561,3.30006519349576));
#14113=CARTESIAN_POINT('Ctrl Pts',(1.41212108228072,0.147252330899258,3.30006519349576));
#14114=CARTESIAN_POINT('Ctrl Pts',(0.598137797989503,-1.88914077016867,
3.31897283641381));
#14115=CARTESIAN_POINT('Ctrl Pts',(1.16176261417605,0.214335680246198,3.31897283641381));
#14116=CARTESIAN_POINT('Ctrl Pts',(0.332208473855475,-1.81788522252321,
3.33300441174764));
#14117=CARTESIAN_POINT('Ctrl Pts',(0.895833290042021,0.285591227891658,
3.33300441174764));
#14118=CARTESIAN_POINT('Ctrl Pts',(0.0542349483243482,-1.74340244083991,
3.34293392264922));
#14119=CARTESIAN_POINT('Ctrl Pts',(0.617859764510894,0.360074009574958,
3.34293392264922));
#14120=CARTESIAN_POINT('Ctrl Pts',(-0.231942319271813,-1.66672147309537,
3.34897162637417));
#14121=CARTESIAN_POINT('Ctrl Pts',(0.331682496914733,0.436754977319498,
3.34897162637417));
#14122=CARTESIAN_POINT('Ctrl Pts',(-0.522273747531617,-1.58892740135578,
3.35102435732185));
#14123=CARTESIAN_POINT('Ctrl Pts',(0.0413510686549291,0.514549049059088,
3.35102435732185));
#14124=CARTESIAN_POINT('Ctrl Pts',(-0.812605175791414,-1.5111333296162,
3.34897162637426));
#14125=CARTESIAN_POINT('Ctrl Pts',(-0.248980359604868,0.592343120798668,
3.34897162637426));
#14126=CARTESIAN_POINT('Ctrl Pts',(-1.09878244338755,-1.43445236187167,
3.34293392264938));
#14127=CARTESIAN_POINT('Ctrl Pts',(-0.535157627201004,0.669024088543198,
3.34293392264938));
#14128=CARTESIAN_POINT('Ctrl Pts',(-1.37675596891866,-1.35996958018837,
3.33300441174785));
#14129=CARTESIAN_POINT('Ctrl Pts',(-0.813131152732114,0.743506870226498,
3.33300441174785));
#14130=CARTESIAN_POINT('Ctrl Pts',(-1.64268529305271,-1.2887140325429,3.31897283641402));
#14131=CARTESIAN_POINT('Ctrl Pts',(-1.07906047686616,0.814762417871968,
3.31897283641402));
#14132=CARTESIAN_POINT('Ctrl Pts',(-1.8930437611574,-1.22163068319595,3.30006519349591));
#14133=CARTESIAN_POINT('Ctrl Pts',(-1.32941894497085,0.881845767218918,
3.30006519349591));
#14134=CARTESIAN_POINT('Ctrl Pts',(-2.12472293626507,-1.15955243532275,
3.27464765209779));
#14135=CARTESIAN_POINT('Ctrl Pts',(-1.56109812007852,0.943924015092118,
3.27464765209779));
#14136=CARTESIAN_POINT('Ctrl Pts',(-2.33513773482719,-1.10317195997247,
3.24001322621208));
#14137=CARTESIAN_POINT('Ctrl Pts',(-1.77151291864064,1.0003044904424,3.24001322621208));
#14138=CARTESIAN_POINT('Ctrl Pts',(-2.52232995605521,-1.05301395546503,
3.19196918412254));
#14139=CARTESIAN_POINT('Ctrl Pts',(-1.95870513986866,1.05046249494984,3.19196918412254));
#14140=CARTESIAN_POINT('Ctrl Pts',(-2.68507677070033,-1.00940607791014,
3.12505646843295));
#14141=CARTESIAN_POINT('Ctrl Pts',(-2.12145195451378,1.09407037250473,3.12505646843295));
#14142=CARTESIAN_POINT('Ctrl Pts',(-2.82300528751688,-0.972448243215919,
3.03403241435609));
#14143=CARTESIAN_POINT('Ctrl Pts',(-2.25938047133033,1.13102820719895,3.03403241435609));
#14144=CARTESIAN_POINT('Ctrl Pts',(-2.93671035054001,-0.94198106340354,
2.91510580081997));
#14145=CARTESIAN_POINT('Ctrl Pts',(-2.37308553435346,1.16149538701133,2.91510580081997));
#14146=CARTESIAN_POINT('Ctrl Pts',(-3.02786158735262,-0.917557163110504,
2.76722839711793));
#14147=CARTESIAN_POINT('Ctrl Pts',(-2.46423677116607,1.18591928730436,2.76722839711793));
#14148=CARTESIAN_POINT('Ctrl Pts',(-3.09934100177414,-0.898404311740807,
2.59347738935767));
#14149=CARTESIAN_POINT('Ctrl Pts',(-2.53571618558759,1.20507213867406,2.59347738935767));
#14150=CARTESIAN_POINT('Ctrl Pts',(-3.15473029191589,-0.883562796177992,
2.39962532458057));
#14151=CARTESIAN_POINT('Ctrl Pts',(-2.59110547572934,1.21991365423688,2.39962532458057));
#14152=CARTESIAN_POINT('Ctrl Pts',(-3.19775217034456,-0.872035118596162,
2.19251877196088));
#14153=CARTESIAN_POINT('Ctrl Pts',(-2.63412735415801,1.23144133181871,2.19251877196088));
#14154=CARTESIAN_POINT('Ctrl Pts',(-3.23174540145526,-0.862926659771925,
1.97856787413951));
#14155=CARTESIAN_POINT('Ctrl Pts',(-2.66812058526871,1.24054979064294,1.97856787413951));
#14156=CARTESIAN_POINT('Ctrl Pts',(-3.25908631610399,-0.855600683771469,
1.76209503442131));
#14157=CARTESIAN_POINT('Ctrl Pts',(-2.69546149991744,1.2478757666434,1.76209503442131));
#14158=CARTESIAN_POINT('Ctrl Pts',(-3.28074793135931,-0.849796471457051,
1.54401727992238));
#14159=CARTESIAN_POINT('Ctrl Pts',(-2.71712311517276,1.25367997895782,1.54401727992238));
#14160=CARTESIAN_POINT('Ctrl Pts',(-3.29722953615212,-0.84538023876285,
1.32371934078708));
#14161=CARTESIAN_POINT('Ctrl Pts',(-2.73360471996557,1.25809621165202,1.32371934078708));
#14162=CARTESIAN_POINT('Ctrl Pts',(-3.30933395645652,-0.842136869117439,
1.10060381648384));
#14163=CARTESIAN_POINT('Ctrl Pts',(-2.74570914026997,1.26133958129743,1.10060381648384));
#14164=CARTESIAN_POINT('Ctrl Pts',(-3.31908373992304,-0.839524422511207,
0.875890304828914));
#14165=CARTESIAN_POINT('Ctrl Pts',(-2.75545892373649,1.26395202790366,0.875890304828914));
#14166=CARTESIAN_POINT('Ctrl Pts',(-3.3303931391277,-0.836494078127436,
0.654020230869684));
#14167=CARTESIAN_POINT('Ctrl Pts',(-2.76676832294115,1.26698237228743,0.654020230869684));
#14168=CARTESIAN_POINT('Ctrl Pts',(-3.35031539848996,-0.831155924819917,
0.444963858672577));
#14169=CARTESIAN_POINT('Ctrl Pts',(-2.78669058230341,1.27232052559495,0.444963858672577));
#14170=CARTESIAN_POINT('Ctrl Pts',(-3.38758891539696,-0.821168516065618,
0.262319630540737));
#14171=CARTESIAN_POINT('Ctrl Pts',(-2.82396409921041,1.28230793434925,0.262319630540737));
#14172=CARTESIAN_POINT('Ctrl Pts',(-3.4496387877668,-0.804542302873664,
0.11901737132707));
#14173=CARTESIAN_POINT('Ctrl Pts',(-2.88601397158025,1.2989341475412,0.11901737132707));
#14174=CARTESIAN_POINT('Ctrl Pts',(-3.54033539990049,-0.780240218896203,
0.0241851999813871));
#14175=CARTESIAN_POINT('Ctrl Pts',(-2.97671058371394,1.32323623151866,0.0241851999813871));
#14176=CARTESIAN_POINT('Ctrl Pts',(-3.65680931559247,-0.749031127247248,
-0.0214179570895714));
#14177=CARTESIAN_POINT('Ctrl Pts',(-3.09318449940592,1.35444532316762,-0.0214179570895714));
#14178=CARTESIAN_POINT('Ctrl Pts',(-3.78869391002249,-0.713692756675616,
-0.0263068037112043));
#14179=CARTESIAN_POINT('Ctrl Pts',(-3.22506909383594,1.38978369373925,-0.0263068037112043));
#14180=CARTESIAN_POINT('Ctrl Pts',(-3.92277049429866,-0.677767044194892,
-0.00118366394785932));
#14181=CARTESIAN_POINT('Ctrl Pts',(-3.35914567811211,1.42570940621998,-0.00118366394785932));
#14182=CARTESIAN_POINT('Ctrl Pts',(-4.04675976550942,-0.644544219103847,
0.0470540298718583));
#14183=CARTESIAN_POINT('Ctrl Pts',(-3.48313494932287,1.45893223131102,0.0470540298718583));
#14184=CARTESIAN_POINT('Ctrl Pts',(-4.15292154232371,-0.616098256739405,
0.120497232333251));
#14185=CARTESIAN_POINT('Ctrl Pts',(-3.58929672613716,1.48737819367546,0.120497232333251));
#14186=CARTESIAN_POINT('Ctrl Pts',(-4.23720717254246,-0.593513990188742,
0.224659532804408));
#14187=CARTESIAN_POINT('Ctrl Pts',(-3.67358235635591,1.50996246022613,0.224659532804408));
#14188=CARTESIAN_POINT('Ctrl Pts',(-4.29891402785718,-0.576979688139698,
0.364350357241515));
#14189=CARTESIAN_POINT('Ctrl Pts',(-3.73528921167063,1.52649676227517,0.364350357241515));
#14190=CARTESIAN_POINT('Ctrl Pts',(-4.34018444275717,-0.565921313795949,
0.538436816836325));
#14191=CARTESIAN_POINT('Ctrl Pts',(-3.77655962657062,1.53755513661892,0.538436816836325));
#14192=CARTESIAN_POINT('Ctrl Pts',(-4.36512660693517,-0.559238081046971,
0.741129277895169));
#14193=CARTESIAN_POINT('Ctrl Pts',(-3.80150179074862,1.5442383693679,0.741129277895169));
#14194=CARTESIAN_POINT('Ctrl Pts',(-4.37883282444249,-0.555565511134598,
0.964078729991154));
#14195=CARTESIAN_POINT('Ctrl Pts',(-3.81520800825594,1.54791093928027,0.964078729991154));
#14196=CARTESIAN_POINT('Ctrl Pts',(-4.38643606159726,-0.553528229879115,
1.1981954227983));
#14197=CARTESIAN_POINT('Ctrl Pts',(-3.82281124541071,1.54994822053575,1.1981954227983));
#14198=CARTESIAN_POINT('Ctrl Pts',(-4.39215243495502,-0.551996532254268,
1.43558101932923));
#14199=CARTESIAN_POINT('Ctrl Pts',(-3.82852761876847,1.5514799181606,1.43558101932923));
#14200=CARTESIAN_POINT('Ctrl Pts',(-4.39832390226062,-0.550342892573617,
1.67142113207667));
#14201=CARTESIAN_POINT('Ctrl Pts',(-3.83469908607407,1.55313355784125,1.67142113207667));
#14202=CARTESIAN_POINT('Ctrl Pts',(-4.40593993377794,-0.548302183079021,
1.90332556813333));
#14203=CARTESIAN_POINT('Ctrl Pts',(-3.84231511759139,1.55517426733585,1.90332556813333));
#14204=CARTESIAN_POINT('Ctrl Pts',(-4.41515781144595,-0.54583226020195,
2.130657485557));
#14205=CARTESIAN_POINT('Ctrl Pts',(-3.8515329952594,1.55764419021292,2.130657485557));
#14206=CARTESIAN_POINT('Ctrl Pts',(-4.42583901148565,-0.542970241277118,
2.35385258470204));
#14207=CARTESIAN_POINT('Ctrl Pts',(-3.8622141952991,1.56050620913775,2.35385258470204));
#14208=CARTESIAN_POINT('Ctrl Pts',(-4.43804296945989,-0.539700200593456,
2.57377631141659));
#14209=CARTESIAN_POINT('Ctrl Pts',(-3.87441815327334,1.56377624982141,2.57377631141659));
#14210=CARTESIAN_POINT('Ctrl Pts',(-4.45084745128755,-0.536269250028235,
2.76449836272519));
#14211=CARTESIAN_POINT('Ctrl Pts',(-3.887222635101,1.56720720038663,2.76449836272519));
#14212=CARTESIAN_POINT('Ctrl Pts',(-4.46320446802865,-0.532958197371602,
2.91011271894269));
#14213=CARTESIAN_POINT('Ctrl Pts',(-3.8995796518421,1.57051825304327,2.91011271894269));
#14214=CARTESIAN_POINT('Ctrl Pts',(-4.47372590670627,-0.530138986374719,
3.01179023688553));
#14215=CARTESIAN_POINT('Ctrl Pts',(-3.91010109051972,1.57333746404015,3.01179023688553));
#14216=CARTESIAN_POINT('Ctrl Pts',(-4.48058344233111,-0.528301515241974,
3.07055226141567));
#14217=CARTESIAN_POINT('Ctrl Pts',(-3.91695862614456,1.57517493517289,3.07055226141567));
#14218=CARTESIAN_POINT('Ctrl Pts',(-4.48256963531681,-0.527769316435443,
3.08701851589457));
#14219=CARTESIAN_POINT('Ctrl Pts',(-3.91894481913026,1.57570713397942,3.08701851589457));
#14220=CARTESIAN_POINT('',(-4.39990749973883,0.13143350442279,11.8105861003151));
#14221=CARTESIAN_POINT('Ctrl Pts',(-4.39990749973883,0.131433504422787,
11.8105861003151));
#14222=CARTESIAN_POINT('Ctrl Pts',(-4.49754913369766,0.157596501389713,
11.7068367844248));
#14223=CARTESIAN_POINT('Ctrl Pts',(-4.69125400852046,0.209499566168453,
11.5019717467543));
#14224=CARTESIAN_POINT('Ctrl Pts',(-5.00967190543604,0.294819384502599,
11.2375756728753));
#14225=CARTESIAN_POINT('Ctrl Pts',(-5.35454459136527,0.38722774218889,11.0061555791443));
#14226=CARTESIAN_POINT('Ctrl Pts',(-5.71913861942256,0.48492041757205,10.8005509999885));
#14227=CARTESIAN_POINT('Ctrl Pts',(-6.06462842910348,0.577494133069235,
10.66692181492));
#14228=CARTESIAN_POINT('Ctrl Pts',(-6.33148581479284,0.648998354058979,
10.6014247262997));
#14229=CARTESIAN_POINT('Ctrl Pts',(-6.60565152217716,0.722460833944915,
10.5327688098564));
#14230=CARTESIAN_POINT('Ctrl Pts',(-6.85297550359782,0.78873109503543,10.4523928827042));
#14231=CARTESIAN_POINT('Ctrl Pts',(-7.10446088941469,0.856116401073289,
10.2839337584245));
#14232=CARTESIAN_POINT('Ctrl Pts',(-7.35838141384484,0.924154200536037,
10.0446906337461));
#14233=CARTESIAN_POINT('Ctrl Pts',(-7.62832379034323,0.996485042321717,
9.6700018953962));
#14234=CARTESIAN_POINT('Ctrl Pts',(-7.86849512871787,1.0608387584843,9.24528298390541));
#14235=CARTESIAN_POINT('Ctrl Pts',(-8.00203202129173,1.09661986100923,8.8659022538591));
#14236=CARTESIAN_POINT('Ctrl Pts',(-8.07463904021301,1.11607485309402,8.47098152553076));
#14237=CARTESIAN_POINT('Ctrl Pts',(-8.08171248804463,1.11797017772821,8.08076694642368));
#14238=CARTESIAN_POINT('Ctrl Pts',(-8.11167522300546,1.12599866836399,7.7043597380442));
#14239=CARTESIAN_POINT('Ctrl Pts',(-8.15245921105438,1.13692670502582,7.42372739456374));
#14240=CARTESIAN_POINT('Ctrl Pts',(-8.20488040179384,1.15097292075073,7.14034281931128));
#14241=CARTESIAN_POINT('Ctrl Pts',(-8.2477646225197,1.16246371306227,6.84786314045739));
#14242=CARTESIAN_POINT('Ctrl Pts',(-8.2340924899642,1.15880027618521,6.58185725748997));
#14243=CARTESIAN_POINT('Ctrl Pts',(-8.15624193537567,1.1379402829529,6.37882425840707));
#14244=CARTESIAN_POINT('Ctrl Pts',(-8.06959783090691,1.11472406513158,6.24539149037989));
#14245=CARTESIAN_POINT('Ctrl Pts',(-7.96390674795061,1.08640422480626,6.13212489925341));
#14246=CARTESIAN_POINT('Ctrl Pts',(-7.80782708725179,1.04458280576709,6.00502448889162));
#14247=CARTESIAN_POINT('Ctrl Pts',(-7.51121080585291,0.965104712704338,
5.83268998867983));
#14248=CARTESIAN_POINT('Ctrl Pts',(-7.07025856977831,0.846951917147452,
5.6633705113799));
#14249=CARTESIAN_POINT('Ctrl Pts',(-6.55772910172197,0.709620060084601,
5.45056821320793));
#14250=CARTESIAN_POINT('Ctrl Pts',(-6.05533862945534,0.575004938755668,
5.20523396509008));
#14251=CARTESIAN_POINT('Ctrl Pts',(-5.47842644000812,0.420421783489613,
4.90183331737205));
#14252=CARTESIAN_POINT('Ctrl Pts',(-4.97546534076346,0.28565376312274,4.5730826167126));
#14253=CARTESIAN_POINT('Ctrl Pts',(-4.62774205069207,0.192481588358615,
4.14707585774942));
#14254=CARTESIAN_POINT('Ctrl Pts',(-4.50892895738859,0.160645715957704,
3.89751682838105));
#14255=CARTESIAN_POINT('Ctrl Pts',(-4.4618940931088,0.148042762057827,3.76716196298096));
#14256=CARTESIAN_POINT('',(-4.38674149674992,0.152249769835312,11.8181058720863));
#14257=CARTESIAN_POINT('Ctrl Pts',(-4.38674149675009,0.152249769834917,
11.8181058720862));
#14258=CARTESIAN_POINT('Ctrl Pts',(-4.3869775568074,0.151688294341147,11.8180210706515));
#14259=CARTESIAN_POINT('Ctrl Pts',(-4.38748854871073,0.150590557851844,
11.8178062692381));
#14260=CARTESIAN_POINT('Ctrl Pts',(-4.38858693511445,0.14845239833212,11.817285750215));
#14261=CARTESIAN_POINT('Ctrl Pts',(-4.39064941066155,0.144825508674648,
11.8162052857216));
#14262=CARTESIAN_POINT('Ctrl Pts',(-4.39446005348131,0.138892971386962,
11.8140046108773));
#14263=CARTESIAN_POINT('Ctrl Pts',(-4.3978421585968,0.134197554896133,11.8118993900741));
#14264=CARTESIAN_POINT('Ctrl Pts',(-4.39990749973883,0.131433504422785,
11.8105861003151));
#14265=CARTESIAN_POINT('',(-4.34854691846782,0.241356558688882,11.8322728954492));
#14266=CARTESIAN_POINT('Origin',(-1.23271387586545,-1.70581675488325,15.3403250734267));
#14267=CARTESIAN_POINT('',(-4.25518135747447,0.44557426920425,11.8702643430631));
#14268=CARTESIAN_POINT('Ctrl Pts',(-4.25518135747447,0.445574269204249,
11.8702643430631));
#14269=CARTESIAN_POINT('Ctrl Pts',(-4.28743714356257,0.378238787953571,
11.8563818704341));
#14270=CARTESIAN_POINT('Ctrl Pts',(-4.31850684021249,0.310110504419452,
11.8437528706395));
#14271=CARTESIAN_POINT('Ctrl Pts',(-4.34854691846782,0.241356558688883,
11.8322728954492));
#14272=CARTESIAN_POINT('',(-4.2368109319615,0.483558887244307,11.8782524024265));
#14273=CARTESIAN_POINT('Origin',(-1.56538794823573,-1.42563865727917,14.6978241049146));
#14274=CARTESIAN_POINT('Origin',(-1.70912501884918,-1.31404604504918,14.5049189366084));
#14275=CARTESIAN_POINT('Ctrl Pts',(-4.39990749973883,0.131433504422787,
11.8105861003151));
#14276=CARTESIAN_POINT('Ctrl Pts',(-4.49754913369766,0.157596501389713,
11.7068367844248));
#14277=CARTESIAN_POINT('Ctrl Pts',(-4.69125400852046,0.209499566168453,
11.5019717467543));
#14278=CARTESIAN_POINT('Ctrl Pts',(-5.00967190543604,0.294819384502599,
11.2375756728753));
#14279=CARTESIAN_POINT('Ctrl Pts',(-5.35454459136527,0.38722774218889,11.0061555791443));
#14280=CARTESIAN_POINT('Ctrl Pts',(-5.71913861942256,0.48492041757205,10.8005509999885));
#14281=CARTESIAN_POINT('Ctrl Pts',(-6.06462842910348,0.577494133069235,
10.66692181492));
#14282=CARTESIAN_POINT('Ctrl Pts',(-6.33148581479284,0.648998354058979,
10.6014247262997));
#14283=CARTESIAN_POINT('Ctrl Pts',(-6.60565152217716,0.722460833944915,
10.5327688098564));
#14284=CARTESIAN_POINT('Ctrl Pts',(-6.85297550359782,0.78873109503543,10.4523928827042));
#14285=CARTESIAN_POINT('Ctrl Pts',(-7.10446088941469,0.856116401073289,
10.2839337584245));
#14286=CARTESIAN_POINT('Ctrl Pts',(-7.35838141384484,0.924154200536037,
10.0446906337461));
#14287=CARTESIAN_POINT('Ctrl Pts',(-7.62832379034323,0.996485042321717,
9.6700018953962));
#14288=CARTESIAN_POINT('Ctrl Pts',(-7.86849512871787,1.0608387584843,9.24528298390541));
#14289=CARTESIAN_POINT('Ctrl Pts',(-8.00203202129173,1.09661986100923,8.8659022538591));
#14290=CARTESIAN_POINT('Ctrl Pts',(-8.07463904021301,1.11607485309402,8.47098152553076));
#14291=CARTESIAN_POINT('Ctrl Pts',(-8.08171248804463,1.11797017772821,8.08076694642368));
#14292=CARTESIAN_POINT('Ctrl Pts',(-8.11167522300546,1.12599866836399,7.7043597380442));
#14293=CARTESIAN_POINT('Ctrl Pts',(-8.15245921105438,1.13692670502582,7.42372739456374));
#14294=CARTESIAN_POINT('Ctrl Pts',(-8.20488040179384,1.15097292075073,7.14034281931128));
#14295=CARTESIAN_POINT('Ctrl Pts',(-8.2477646225197,1.16246371306227,6.84786314045739));
#14296=CARTESIAN_POINT('Ctrl Pts',(-8.2340924899642,1.15880027618521,6.58185725748997));
#14297=CARTESIAN_POINT('Ctrl Pts',(-8.15624193537567,1.1379402829529,6.37882425840707));
#14298=CARTESIAN_POINT('Ctrl Pts',(-8.06959783090691,1.11472406513158,6.24539149037989));
#14299=CARTESIAN_POINT('Ctrl Pts',(-7.96390674795061,1.08640422480626,6.13212489925341));
#14300=CARTESIAN_POINT('Ctrl Pts',(-7.80782708725179,1.04458280576709,6.00502448889162));
#14301=CARTESIAN_POINT('Ctrl Pts',(-7.51121080585291,0.965104712704338,
5.83268998867983));
#14302=CARTESIAN_POINT('Ctrl Pts',(-7.07025856977831,0.846951917147452,
5.6633705113799));
#14303=CARTESIAN_POINT('Ctrl Pts',(-6.55772910172197,0.709620060084601,
5.45056821320793));
#14304=CARTESIAN_POINT('Ctrl Pts',(-6.05533862945534,0.575004938755668,
5.20523396509008));
#14305=CARTESIAN_POINT('Ctrl Pts',(-5.47842644000812,0.420421783489613,
4.90183331737205));
#14306=CARTESIAN_POINT('Ctrl Pts',(-4.97546534076346,0.28565376312274,4.5730826167126));
#14307=CARTESIAN_POINT('Ctrl Pts',(-4.62774205069207,0.192481588358615,
4.14707585774942));
#14308=CARTESIAN_POINT('Ctrl Pts',(-4.50892895738859,0.160645715957704,
3.89751682838105));
#14309=CARTESIAN_POINT('Ctrl Pts',(-4.4618940931088,0.148042762057827,3.76716196298096));
#14310=CARTESIAN_POINT('Ctrl Pts',(-4.40610257791561,0.10831315791016,11.8105861003151));
#14311=CARTESIAN_POINT('Ctrl Pts',(-4.50374507702499,0.134476386693474,
11.7068358651574));
#14312=CARTESIAN_POINT('Ctrl Pts',(-4.69744752408798,0.186378800955935,
11.5019742817009));
#14313=CARTESIAN_POINT('Ctrl Pts',(-5.01586638212965,0.271698876823038,
11.2375781425806));
#14314=CARTESIAN_POINT('Ctrl Pts',(-5.36073964308098,0.364107388586036,
11.0061565233321));
#14315=CARTESIAN_POINT('Ctrl Pts',(-5.72534334415641,0.461802655846596,
10.8005488998531));
#14316=CARTESIAN_POINT('Ctrl Pts',(-6.07081472117805,0.554371432327612,
10.6669268865357));
#14317=CARTESIAN_POINT('Ctrl Pts',(-6.33766369106806,0.62587339831072,10.6014312575901));
#14318=CARTESIAN_POINT('Ctrl Pts',(-6.61182227957146,0.699333970698262,
10.5327811735249));
#14319=CARTESIAN_POINT('Ctrl Pts',(-6.85916868333988,0.765610239838752,
10.4524004053925));
#14320=CARTESIAN_POINT('Ctrl Pts',(-7.11066195746784,0.832997659543196,
10.2839369025062));
#14321=CARTESIAN_POINT('Ctrl Pts',(-7.36459656854927,0.901039233512779,
10.0446770327022));
#14322=CARTESIAN_POINT('Ctrl Pts',(-7.63451688382228,0.973364164010934,
9.67000537128577));
#14323=CARTESIAN_POINT('Ctrl Pts',(-7.87469455084438,1.0377195759295,9.24528421592605));
#14324=CARTESIAN_POINT('Ctrl Pts',(-8.00823128702896,1.07350063655004,8.86590036282094));
#14325=CARTESIAN_POINT('Ctrl Pts',(-8.08083869530086,1.09295573296102,8.47096393307005));
#14326=CARTESIAN_POINT('Ctrl Pts',(-8.08790913116448,1.09485025054081,8.08075207953364));
#14327=CARTESIAN_POINT('Ctrl Pts',(-8.11787189500846,1.10287874891581,7.70436013759456));
#14328=CARTESIAN_POINT('Ctrl Pts',(-8.15865443057292,1.1138063963856,7.42374345640766));
#14329=CARTESIAN_POINT('Ctrl Pts',(-8.21107842618733,1.12785336367449,7.14036999923671));
#14330=CARTESIAN_POINT('Ctrl Pts',(-8.25396944631471,1.13934597788017,6.84789820200929));
#14331=CARTESIAN_POINT('Ctrl Pts',(-8.24031812870394,1.13568811835075,6.58189724851307));
#14332=CARTESIAN_POINT('Ctrl Pts',(-8.16244596760929,1.11482233567257,6.37880997093398));
#14333=CARTESIAN_POINT('Ctrl Pts',(-8.07579191235616,1.09160345154661,6.24536441066714));
#14334=CARTESIAN_POINT('Ctrl Pts',(-7.97009137637762,1.06328107829162,6.13209608067231));
#14335=CARTESIAN_POINT('Ctrl Pts',(-7.81399260224414,1.02145453782307,6.00498322378118));
#14336=CARTESIAN_POINT('Ctrl Pts',(-7.51738480597013,0.941978718342671,
5.83267352057959));
#14337=CARTESIAN_POINT('Ctrl Pts',(-7.07644541070296,0.823829363469767,
5.66336515001065));
#14338=CARTESIAN_POINT('Ctrl Pts',(-6.56392284376063,0.686499355554842,
5.45056727419079));
#14339=CARTESIAN_POINT('Ctrl Pts',(-6.06153370995061,0.551884592864275,
5.20523328921882));
#14340=CARTESIAN_POINT('Ctrl Pts',(-5.48461630527476,0.397300040181924,
4.90183082421786));
#14341=CARTESIAN_POINT('Ctrl Pts',(-4.98165380025924,0.26253164313988,4.57306922084908));
#14342=CARTESIAN_POINT('Ctrl Pts',(-4.63394385126977,0.169363043107885,
4.14707693759231));
#14343=CARTESIAN_POINT('Ctrl Pts',(-4.51511830855761,0.137523834897972,
3.89750095625433));
#14344=CARTESIAN_POINT('Ctrl Pts',(-4.46808917128558,0.124922415545199,
3.76716196298096));
#14345=CARTESIAN_POINT('Ctrl Pts',(-4.40291516435328,0.0645741697282324,
11.796556443628));
#14346=CARTESIAN_POINT('Ctrl Pts',(-4.50048856350348,0.0907188832332889,
11.6928796307718));
#14347=CARTESIAN_POINT('Ctrl Pts',(-4.69504931294762,0.14285127892564,11.4870859088997));
#14348=CARTESIAN_POINT('Ctrl Pts',(-5.0153119872158,0.228665403861629,11.2211535933451));
#14349=CARTESIAN_POINT('Ctrl Pts',(-5.36151215707251,0.321429459794252,
10.9888940346623));
#14350=CARTESIAN_POINT('Ctrl Pts',(-5.72763036696513,0.419530538469309,
10.7823369202495));
#14351=CARTESIAN_POINT('Ctrl Pts',(-6.0761462566863,0.51291508966951,10.6475498808516));
#14352=CARTESIAN_POINT('Ctrl Pts',(-6.3440656643213,0.584703878581932,10.5818347915591));
#14353=CARTESIAN_POINT('Ctrl Pts',(-6.61761927622536,0.658002347978243,
10.5133104011913));
#14354=CARTESIAN_POINT('Ctrl Pts',(-6.861888253579,0.723454023196128,10.4338049599974));
#14355=CARTESIAN_POINT('Ctrl Pts',(-7.10935635790786,0.789762901903506,
10.2680061458923));
#14356=CARTESIAN_POINT('Ctrl Pts',(-7.36030385820222,0.85700408194999,10.0317153152368));
#14357=CARTESIAN_POINT('Ctrl Pts',(-7.62907538108075,0.929021194453772,
9.65885131647057));
#14358=CARTESIAN_POINT('Ctrl Pts',(-7.86798181564301,0.993035980661329,
9.23617470335927));
#14359=CARTESIAN_POINT('Ctrl Pts',(-8.00012724262594,1.02844424110487,8.86049547284917));
#14360=CARTESIAN_POINT('Ctrl Pts',(-8.07209396647679,1.04772766664262,8.46966777014732));
#14361=CARTESIAN_POINT('Ctrl Pts',(-8.07922818767295,1.04963927545076,8.08019062380329));
#14362=CARTESIAN_POINT('Ctrl Pts',(-8.10927699136119,1.05769082813254,7.70205072960373));
#14363=CARTESIAN_POINT('Ctrl Pts',(-8.15026361671259,1.06867316129593,7.42011617327014));
#14364=CARTESIAN_POINT('Ctrl Pts',(-8.20272880746984,1.08273116679008,7.13664584277076));
#14365=CARTESIAN_POINT('Ctrl Pts',(-8.24520628166168,1.0941129716963,6.84609737205768));
#14366=CARTESIAN_POINT('Ctrl Pts',(-8.23158429149218,1.09046297043107,6.58572297937688));
#14367=CARTESIAN_POINT('Ctrl Pts',(-8.15587046120199,1.07017551074895,6.38835239922954));
#14368=CARTESIAN_POINT('Ctrl Pts',(-8.07141284400203,1.04754516042556,6.258182462026));
#14369=CARTESIAN_POINT('Ctrl Pts',(-7.96785647648126,1.01979731537727,6.14717486337006));
#14370=CARTESIAN_POINT('Ctrl Pts',(-7.81419507107175,0.978623865889961,
6.02200778579695));
#14371=CARTESIAN_POINT('Ctrl Pts',(-7.52061390092899,0.899959028437226,
5.85130334614999));
#14372=CARTESIAN_POINT('Ctrl Pts',(-7.08058961552272,0.782054876512532,
5.68226275410023));
#14373=CARTESIAN_POINT('Ctrl Pts',(-6.56675458224047,0.644373194301734,
5.46896563973939));
#14374=CARTESIAN_POINT('Ctrl Pts',(-6.06367525013762,0.509573493535987,
5.2232740147586));
#14375=CARTESIAN_POINT('Ctrl Pts',(-5.48616446123447,0.354829944029128,
4.91953641642625));
#14376=CARTESIAN_POINT('Ctrl Pts',(-4.9801291599051,0.219238193696283,4.58909349075147));
#14377=CARTESIAN_POINT('Ctrl Pts',(-4.62817642216375,0.124932741844566,
4.15817276994372));
#14378=CARTESIAN_POINT('Ctrl Pts',(-4.50810575167473,0.0927599026523696,
3.90580371045959));
#14379=CARTESIAN_POINT('Ctrl Pts',(-4.46061919574128,0.080035918338667,
3.77419700335406));
#14380=CARTESIAN_POINT('Ctrl Pts',(-4.37768603361793,0.0426571860882519,
11.7672856238756));
#14381=CARTESIAN_POINT('Ctrl Pts',(-4.4751175795493,0.0687638901378774,
11.6637595374443));
#14382=CARTESIAN_POINT('Ctrl Pts',(-4.67146255830039,0.121374368632138,
11.4560302833013));
#14383=CARTESIAN_POINT('Ctrl Pts',(-4.99557465491178,0.208219943176319,
11.1868927865811));
#14384=CARTESIAN_POINT('Ctrl Pts',(-5.34454476327236,0.301726201894137,
10.9528809104907));
#14385=CARTESIAN_POINT('Ctrl Pts',(-5.71384864247256,0.400680878087512,
10.7443346810372));
#14386=CARTESIAN_POINT('Ctrl Pts',(-6.06866716597707,0.495754214920148,
10.6071361653846));
#14387=CARTESIAN_POINT('Ctrl Pts',(-6.33879737818042,0.568135387131283,
10.540967107949));
#14388=CARTESIAN_POINT('Ctrl Pts',(-6.61106975689777,0.641090551129898,
10.4727205567864));
#14389=CARTESIAN_POINT('Ctrl Pts',(-6.84897810060804,0.704837899699691,
10.3950284103723));
#14390=CARTESIAN_POINT('Ctrl Pts',(-7.08806937487797,0.768902213557648,
10.234777368477));
#14391=CARTESIAN_POINT('Ctrl Pts',(-7.3328223793598,0.834483583453643,10.0046362201527));
#14392=CARTESIAN_POINT('Ctrl Pts',(-7.59913811631925,0.905842670103627,
9.63558931371895));
#14393=CARTESIAN_POINT('Ctrl Pts',(-7.83540923585815,0.969151325778873,
9.21717233709717));
#14394=CARTESIAN_POINT('Ctrl Pts',(-7.9646514821359,1.00378168129698,8.84921390584317));
#14395=CARTESIAN_POINT('Ctrl Pts',(-8.03528255322126,1.02270721975485,8.46691646823682));
#14396=CARTESIAN_POINT('Ctrl Pts',(-8.04254179813168,1.02465232856626,8.07897946972552));
#14397=CARTESIAN_POINT('Ctrl Pts',(-8.07277018857148,1.03275200137309,7.69723355728135));
#14398=CARTESIAN_POINT('Ctrl Pts',(-8.11417873287728,1.04384738737958,7.41259133413029));
#14399=CARTESIAN_POINT('Ctrl Pts',(-8.16673737243891,1.0579304324054,7.12894862515868));
#14400=CARTESIAN_POINT('Ctrl Pts',(-8.20837022762595,1.06908592233137,6.8424339710948));
#14401=CARTESIAN_POINT('Ctrl Pts',(-8.19486509106195,1.06546723189537,6.59381175490167));
#14402=CARTESIAN_POINT('Ctrl Pts',(-8.12359651814278,1.04637087533596,6.40822306593102));
#14403=CARTESIAN_POINT('Ctrl Pts',(-8.04369483483858,1.02496128382071,6.28485302475822));
#14404=CARTESIAN_POINT('Ctrl Pts',(-7.94458667955791,0.998405333649918,
6.17855745994456));
#14405=CARTESIAN_POINT('Ctrl Pts',(-7.79595937050461,0.958580766215877,
6.05741667913553));
#14406=CARTESIAN_POINT('Ctrl Pts',(-7.50871550370568,0.88161400407631,5.89012770190778));
#14407=CARTESIAN_POINT('Ctrl Pts',(-7.0706348013897,0.764230633671083,5.72167549359611));
#14408=CARTESIAN_POINT('Ctrl Pts',(-6.5540799556138,0.625820179899048,5.50734861815085));
#14409=CARTESIAN_POINT('Ctrl Pts',(-6.04956420554889,0.490635592100373,
5.26091153351829));
#14410=CARTESIAN_POINT('Ctrl Pts',(-5.47080146025223,0.335556581888915,
4.95646986864331));
#14411=CARTESIAN_POINT('Ctrl Pts',(-4.95835146085607,0.198246018389383,
4.62248995318707));
#14412=CARTESIAN_POINT('Ctrl Pts',(-4.59758244560127,0.101578252097688,
4.18132548363876));
#14413=CARTESIAN_POINT('Ctrl Pts',(-4.47488070480479,0.0687004197413792,
3.92308374120045));
#14414=CARTESIAN_POINT('Ctrl Pts',(-4.42645512791889,0.0557248255217898,
3.78887458266364));
#14415=CARTESIAN_POINT('Ctrl Pts',(-4.36526624577324,0.0393293139651011,
11.7547577775405));
#14416=CARTESIAN_POINT('Ctrl Pts',(-4.462637168512,0.0654197740792256,11.6512961064053));
#14417=CARTESIAN_POINT('Ctrl Pts',(-4.65974554183767,0.118234803533251,
11.442738806744));
#14418=CARTESIAN_POINT('Ctrl Pts',(-4.98550528234724,0.205521862929361,
11.1722294927876));
#14419=CARTESIAN_POINT('Ctrl Pts',(-5.33566097788268,0.29934579877324,10.9374674705902));
#14420=CARTESIAN_POINT('Ctrl Pts',(-5.70632931912773,0.398666081469635,
10.7280695887413));
#14421=CARTESIAN_POINT('Ctrl Pts',(-6.06384344546407,0.494461702904175,
10.5898397099152));
#14422=CARTESIAN_POINT('Ctrl Pts',(-6.33491900485657,0.567096180131211,
10.5234765064095));
#14423=CARTESIAN_POINT('Ctrl Pts',(-6.60664228072597,0.639904212465156,
10.4553494743371));
#14424=CARTESIAN_POINT('Ctrl Pts',(-6.8418306113212,0.702922735717372,10.3784329123269));
#14425=CARTESIAN_POINT('Ctrl Pts',(-7.07733743840935,0.766026599847657,
10.2205558508687));
#14426=CARTESIAN_POINT('Ctrl Pts',(-7.3194406724111,0.830897965883391,9.99304501740382));
#14427=CARTESIAN_POINT('Ctrl Pts',(-7.58470305177623,0.901974806216633,
9.62563358808958));
#14428=CARTESIAN_POINT('Ctrl Pts',(-7.81984691825478,0.964981415344694,
9.20903949392042));
#14429=CARTESIAN_POINT('Ctrl Pts',(-7.94784659338026,0.999278824926013,
8.84438522402643));
#14430=CARTESIAN_POINT('Ctrl Pts',(-8.01790604838202,1.0180511993159,8.46573709363457));
#14431=CARTESIAN_POINT('Ctrl Pts',(-8.02521849097772,1.02001056240412,8.07845955750479));
#14432=CARTESIAN_POINT('Ctrl Pts',(-8.05552374714506,1.02813083132057,7.6951718595586));
#14433=CARTESIAN_POINT('Ctrl Pts',(-8.09711272128414,1.03927456335518,7.40937238436613));
#14434=CARTESIAN_POINT('Ctrl Pts',(-8.14971164745181,1.05336840314455,7.12565705017148));
#14435=CARTESIAN_POINT('Ctrl Pts',(-8.19098371232079,1.06442721959616,6.8408696776684));
#14436=CARTESIAN_POINT('Ctrl Pts',(-8.17753074630009,1.06082250821511,6.59727787804477));
#14437=CARTESIAN_POINT('Ctrl Pts',(-8.10816249423483,1.04223534109386,6.41672618659136));
#14438=CARTESIAN_POINT('Ctrl Pts',(-8.03020970920239,1.02134795529666,6.29626516002264));
#14439=CARTESIAN_POINT('Ctrl Pts',(-7.93300439915508,0.995301870969469,
6.19198615507442));
#14440=CARTESIAN_POINT('Ctrl Pts',(-7.78652969114894,0.956054091247638,
6.07256733032961));
#14441=CARTESIAN_POINT('Ctrl Pts',(-7.50199905569102,0.879814337254775,
5.90674273368555));
#14442=CARTESIAN_POINT('Ctrl Pts',(-7.06475153359634,0.762654216816996,
5.73854350352349));
#14443=CARTESIAN_POINT('Ctrl Pts',(-6.54703332936491,0.623932042086293,
5.5237763509783));
#14444=CARTESIAN_POINT('Ctrl Pts',(-6.04190293430869,0.488582760658567,
5.27702023853286));
#14445=CARTESIAN_POINT('Ctrl Pts',(-5.46260381387957,0.333360029163525,
4.97227704636915));
#14446=CARTESIAN_POINT('Ctrl Pts',(-4.94740819214276,0.195313778375095,
4.6367821770228));
#14447=CARTESIAN_POINT('Ctrl Pts',(-4.582867212341,0.0976353172291641,4.19123490599198));
#14448=CARTESIAN_POINT('Ctrl Pts',(-4.45903808887791,0.0644554035977742,
3.93047791113146));
#14449=CARTESIAN_POINT('Ctrl Pts',(-4.41021120669539,0.0513722799480397,
3.79515655425571));
#14450=CARTESIAN_POINT('Origin',(-4.34456072216504,0.116603380068226,11.7547577775405));
#14451=CARTESIAN_POINT('Ctrl Pts',(-4.26119373042795,0.0145528918841498,
11.638842338191));
#14452=CARTESIAN_POINT('Ctrl Pts',(-4.26125236043256,0.0145635653496478,
11.6390494463487));
#14453=CARTESIAN_POINT('Ctrl Pts',(-4.2613108171609,0.0145742781139868,
11.6392564542239));
#14454=CARTESIAN_POINT('Ctrl Pts',(-4.27313475944305,0.0168564057035511,
11.6811561932301));
#14455=CARTESIAN_POINT('Ctrl Pts',(-4.28208612481729,0.0278778097684391,
11.7209829966278));
#14456=CARTESIAN_POINT('Ctrl Pts',(-4.28908755611092,0.0448598329498131,
11.7564896488273));
#14457=CARTESIAN_POINT('Ctrl Pts',(-4.26119373042795,0.0145528918841498,
11.638842338191));
#14458=CARTESIAN_POINT('Ctrl Pts',(-4.26127828911038,0.0145682856093495,
11.6390223367578));
#14459=CARTESIAN_POINT('Ctrl Pts',(-4.26136364251986,0.0145842788598119,
11.639202913148));
#14460=CARTESIAN_POINT('Ctrl Pts',(-4.27851654506032,0.0177444550235382,
11.675650547572));
#14461=CARTESIAN_POINT('Ctrl Pts',(-4.29379674050307,0.0238869170482415,
11.7114368827851));
#14462=CARTESIAN_POINT('Ctrl Pts',(-4.30450945627382,0.0325071787760864,
11.7471124459761));
#14463=CARTESIAN_POINT('Ctrl Pts',(-4.26119373042795,0.0145528918841498,
11.638842338191));
#14464=CARTESIAN_POINT('Ctrl Pts',(-4.26130467158735,0.0145730884822054,
11.6389946828916));
#14465=CARTESIAN_POINT('Ctrl Pts',(-4.2614161729233,0.0145934983333006,
11.639149772681));
#14466=CARTESIAN_POINT('Ctrl Pts',(-4.28389600361695,0.0186893116053435,
11.6701638807614));
#14467=CARTESIAN_POINT('Ctrl Pts',(-4.30492281676891,0.023383483481463,
11.7014497023147));
#14468=CARTESIAN_POINT('Ctrl Pts',(-4.32325512462864,0.0279667529147067,
11.7334386747809));
#14469=CARTESIAN_POINT('Ctrl Pts',(-4.26119373042795,0.0145528918841498,
11.638842338191));
#14470=CARTESIAN_POINT('Ctrl Pts',(-4.26133114891829,0.0145779086230217,
11.6389687144068));
#14471=CARTESIAN_POINT('Ctrl Pts',(-4.26146855208158,0.014602959314705,
11.639095090611));
#14472=CARTESIAN_POINT('Ctrl Pts',(-4.28927567952828,0.0196775034910065,
11.6647148078266));
#14473=CARTESIAN_POINT('Ctrl Pts',(-4.3154573308492,0.0258092392550238,
11.6915792314772));
#14474=CARTESIAN_POINT('Ctrl Pts',(-4.33960641395499,0.0324815600844758,
11.7196558802127));
#14475=CARTESIAN_POINT('',(-4.28933390296185,0.0388612606170688,11.7451969266016));
#14476=CARTESIAN_POINT('Origin',(-4.31223161686593,0.107940822411309,11.7119910933921));
#14477=CARTESIAN_POINT('',(-4.26119373042794,0.0145528918841489,11.638842338191));
#14478=CARTESIAN_POINT('Ctrl Pts',(-4.33293714046261,0.0306667563050961,
11.7119910933921));
#14479=CARTESIAN_POINT('Ctrl Pts',(-4.31066098923177,0.0246978795758798,
11.6866819998201));
#14480=CARTESIAN_POINT('Ctrl Pts',(-4.28674775885131,0.0192161812931609,
11.6623857426252));
#14481=CARTESIAN_POINT('Ctrl Pts',(-4.26146855208158,0.014602959314705,
11.639095090611));
#14482=CARTESIAN_POINT('Ctrl Pts',(-4.26133114891829,0.0145779086230217,
11.6389687144068));
#14483=CARTESIAN_POINT('Ctrl Pts',(-4.26119373042795,0.0145528918841498,
11.638842338191));
#14484=CARTESIAN_POINT('Ctrl Pts',(-4.26119373042795,0.0145528918841497,
11.638842338191));
#14485=CARTESIAN_POINT('Ctrl Pts',(-4.26125633218466,0.0145642883985241,
11.6390452934056));
#14486=CARTESIAN_POINT('Ctrl Pts',(-4.26131888429506,0.0145758879335255,
11.639248262593));
#14487=CARTESIAN_POINT('Ctrl Pts',(-4.2613813161263,0.0145876766504085,
11.6394510185953));
#14488=CARTESIAN_POINT('Ctrl Pts',(-4.265016010492,0.0152739993480501,11.6512551909948));
#14489=CARTESIAN_POINT('Ctrl Pts',(-4.26847153091007,0.0166441818282242,
11.6629691301088));
#14490=CARTESIAN_POINT('Ctrl Pts',(-4.27169388060566,0.0186106171418232,
11.6744752186442));
#14491=CARTESIAN_POINT('Ctrl Pts',(-4.27431552229403,0.0202104710629102,
11.6838363508068));
#14492=CARTESIAN_POINT('Ctrl Pts',(-4.27678305604313,0.0222047860179351,
11.6930581330534));
#14493=CARTESIAN_POINT('Ctrl Pts',(-4.2790962892493,0.0245559887567339,
11.7021068786235));
#14494=CARTESIAN_POINT('Ctrl Pts',(-4.28076743592503,0.0262545657227037,
11.7086439545391));
#14495=CARTESIAN_POINT('Ctrl Pts',(-4.28235877711272,0.0281396923832335,
11.7150914206716));
#14496=CARTESIAN_POINT('Ctrl Pts',(-4.28387859102004,0.0302000190087009,
11.7214511909726));
#14497=CARTESIAN_POINT('Ctrl Pts',(-4.2848378009235,0.0315003661722649,
11.7254650736113));
#14498=CARTESIAN_POINT('Ctrl Pts',(-4.28576868964866,0.032870535179902,
11.7294443738346));
#14499=CARTESIAN_POINT('Ctrl Pts',(-4.28667443781518,0.0343117715877457,
11.733390025982));
#14500=CARTESIAN_POINT('Ctrl Pts',(-4.28758560787174,0.0357616353664485,
11.7373592971583));
#14501=CARTESIAN_POINT('Ctrl Pts',(-4.28847140705044,0.0372834000391179,
11.741294500388));
#14502=CARTESIAN_POINT('Ctrl Pts',(-4.28933737923093,0.0388717353254243,
11.7451918804009));
#14503=CARTESIAN_POINT('Ctrl Pts',(-4.28933194406438,0.0388554328133947,
11.7451997357866));
#14504=CARTESIAN_POINT('Ctrl Pts',(-4.29334608958886,0.0462195341306841,
11.7632876305128));
#14505=CARTESIAN_POINT('Ctrl Pts',(-4.29689723089593,0.0549276403535255,
11.780184802912));
#14506=CARTESIAN_POINT('Ctrl Pts',(-4.2998985866006,0.0640783966010583,
11.7953338759064));
#14507=CARTESIAN_POINT('Ctrl Pts',(-4.29723383551483,0.0337205660463619,
11.7399663528515));
#14508=CARTESIAN_POINT('Ctrl Pts',(-4.30223892661807,0.0391552689494062,
11.7577758392426));
#14509=CARTESIAN_POINT('Ctrl Pts',(-4.30655480288613,0.0454981284300141,
11.7748811862141));
#14510=CARTESIAN_POINT('Ctrl Pts',(-4.3097492473298,0.0521509621179001,
11.7907366681496));
#14511=CARTESIAN_POINT('Ctrl Pts',(-4.31216328890714,0.0280798242089688,
11.7292060775775));
#14512=CARTESIAN_POINT('Ctrl Pts',(-4.31962072705201,0.0310704426480294,
11.7457834264563));
#14513=CARTESIAN_POINT('Ctrl Pts',(-4.32641873804203,0.0341585077796439,
11.7622236442056));
#14514=CARTESIAN_POINT('Ctrl Pts',(-4.33187469076345,0.0371197035570584,
11.7782343306969));
#14515=CARTESIAN_POINT('Ctrl Pts',(-4.32692885226188,0.0290568403338177,
11.7171552346107));
#14516=CARTESIAN_POINT('Ctrl Pts',(-4.3370622021989,0.0317709139581999,
11.7318804084193));
#14517=CARTESIAN_POINT('Ctrl Pts',(-4.34688041119116,0.0344079488305172,
11.7466859910022));
#14518=CARTESIAN_POINT('Ctrl Pts',(-4.35575691289273,0.0367812958992088,
11.7617986618842));
#14519=CARTESIAN_POINT('Ctrl Pts',(-4.33293714047413,0.0306667563081824,
11.7119910933921));
#14520=CARTESIAN_POINT('Ctrl Pts',(-4.34410968865593,0.0336604315708949,
11.7259232172676));
#14521=CARTESIAN_POINT('Ctrl Pts',(-4.35509026165876,0.0366026672394349,
11.7400274737341));
#14522=CARTESIAN_POINT('Ctrl Pts',(-4.36526624577325,0.0393293139651038,
11.7547577775405));
#14523=CARTESIAN_POINT('',(-4.29989857489109,0.0640783949723723,11.7953338609094));
#14524=CARTESIAN_POINT('Origin',(-4.34456072216505,0.116603380068228,11.7547577775405));
#14525=CARTESIAN_POINT('Ctrl Pts',(-4.28933737992813,0.0388717366042249,
11.7451918835388));
#14526=CARTESIAN_POINT('Ctrl Pts',(-4.2909926879354,0.0419078436176716,
11.7526417353203));
#14527=CARTESIAN_POINT('Ctrl Pts',(-4.2925597985808,0.045175191270237,11.7599143873744));
#14528=CARTESIAN_POINT('Ctrl Pts',(-4.29404906906754,0.048603587745722,
11.7669287724202));
#14529=CARTESIAN_POINT('Ctrl Pts',(-4.29544178305482,0.0518097049472987,
11.773488381472));
#14530=CARTESIAN_POINT('Ctrl Pts',(-4.29676629412499,0.055156301714286,
11.7798217675776));
#14531=CARTESIAN_POINT('Ctrl Pts',(-4.29801615211051,0.0585984518134254,
11.7859058819922));
#14532=CARTESIAN_POINT('Ctrl Pts',(-4.29854849608121,0.0600645446597914,
11.7884972497021));
#14533=CARTESIAN_POINT('Ctrl Pts',(-4.29906711701482,0.061548155517918,
11.791043982633));
#14534=CARTESIAN_POINT('Ctrl Pts',(-4.2995707431049,0.0630465295669297,
11.7935470041674));
#14535=CARTESIAN_POINT('Ctrl Pts',(-4.29968948856959,0.0633998177031627,
11.7941371690954));
#14536=CARTESIAN_POINT('Ctrl Pts',(-4.29980739879513,0.0637539277173913,
11.794724911699));
#14537=CARTESIAN_POINT('Ctrl Pts',(-4.29992448656911,0.0641087544296572,
11.7953102793706));
#14538=CARTESIAN_POINT('Origin',(-4.34456072216505,0.116603380068228,11.7547577775405));
#14539=CARTESIAN_POINT('Origin',(-4.34456072216505,0.116603380068228,11.7547577775405));
#14540=CARTESIAN_POINT('Ctrl Pts',(-4.2998985866006,0.064078396601051,11.7953338759064));
#14541=CARTESIAN_POINT('Ctrl Pts',(-4.29821195997181,0.0679078725578545,
11.7984345883761));
#14542=CARTESIAN_POINT('Ctrl Pts',(-4.29531934379238,0.0747519942657476,
11.8037156359142));
#14543=CARTESIAN_POINT('Ctrl Pts',(-4.2912761668828,0.0857111829491446,
11.8105333018319));
#14544=CARTESIAN_POINT('Ctrl Pts',(-4.28845382290292,0.0942165736780995,
11.8148613164417));
#14545=CARTESIAN_POINT('Ctrl Pts',(-4.2864128668125,0.100856657618271,11.8176056635397));
#14546=CARTESIAN_POINT('Ctrl Pts',(-4.28514086404414,0.105200715903957,
11.8191332343535));
#14547=CARTESIAN_POINT('Ctrl Pts',(-4.28411650287131,0.108864535984662,
11.8201045080524));
#14548=CARTESIAN_POINT('Ctrl Pts',(-4.30795938649042,0.0651995776992974,
11.8056577506247));
#14549=CARTESIAN_POINT('Ctrl Pts',(-4.30631269428566,0.0692259606646627,
11.8084959096106));
#14550=CARTESIAN_POINT('Ctrl Pts',(-4.30347431591841,0.0763856825373679,
11.8133201493039));
#14551=CARTESIAN_POINT('Ctrl Pts',(-4.29949162445147,0.0876978144383768,
11.8194950118656));
#14552=CARTESIAN_POINT('Ctrl Pts',(-4.29671134521685,0.096384223729235,
11.8233849066295));
#14553=CARTESIAN_POINT('Ctrl Pts',(-4.29470323588274,0.103112943879637,
11.8258358009157));
#14554=CARTESIAN_POINT('Ctrl Pts',(-4.29345297485791,0.107492911285536,
11.8271931981825));
#14555=CARTESIAN_POINT('Ctrl Pts',(-4.29244646900149,0.111166126951951,
11.8280516647877));
#14556=CARTESIAN_POINT('Ctrl Pts',(-4.32773770108309,0.071786906985305,
11.8228894198173));
#14557=CARTESIAN_POINT('Ctrl Pts',(-4.32604509607268,0.0760054220053826,
11.8251425773725));
#14558=CARTESIAN_POINT('Ctrl Pts',(-4.32313045108372,0.0834482477498973,
11.8289613255584));
#14559=CARTESIAN_POINT('Ctrl Pts',(-4.31908434704812,0.0948720157954402,
11.8337366208354));
#14560=CARTESIAN_POINT('Ctrl Pts',(-4.31631218946471,0.103451916842004,
11.8366810362039));
#14561=CARTESIAN_POINT('Ctrl Pts',(-4.31434777281709,0.109977688871195,
11.8385003202736));
#14562=CARTESIAN_POINT('Ctrl Pts',(-4.31314270025451,0.114174994801066,
11.8394921390526));
#14563=CARTESIAN_POINT('Ctrl Pts',(-4.31219079724573,0.11764156937273,11.8401081161105));
#14564=CARTESIAN_POINT('Ctrl Pts',(-4.36711540513978,0.0957581984702657,
11.8342768900003));
#14565=CARTESIAN_POINT('Ctrl Pts',(-4.36512365334321,0.0996049620227929,
11.8357058653262));
#14566=CARTESIAN_POINT('Ctrl Pts',(-4.36174755499454,0.106299259541304,
11.838076628538));
#14567=CARTESIAN_POINT('Ctrl Pts',(-4.35740902944085,0.115985641359757,
11.8408395466436));
#14568=CARTESIAN_POINT('Ctrl Pts',(-4.35465467492231,0.122890231767463,
11.8424013451887));
#14569=CARTESIAN_POINT('Ctrl Pts',(-4.35285551426538,0.127878032137172,
11.8432892482311));
#14570=CARTESIAN_POINT('Ctrl Pts',(-4.35182072520549,0.130969600301793,
11.8437365863237));
#14571=CARTESIAN_POINT('Ctrl Pts',(-4.35107864844448,0.133383930697635,
11.8439884456233));
#14572=CARTESIAN_POINT('Ctrl Pts',(-4.39089217151298,0.118900218345273,
11.8228529842754));
#14573=CARTESIAN_POINT('Ctrl Pts',(-4.38876480488994,0.122050896380848,
11.8241142878602));
#14574=CARTESIAN_POINT('Ctrl Pts',(-4.3852578467149,0.127458307394871,11.8261928035957));
#14575=CARTESIAN_POINT('Ctrl Pts',(-4.38105329091733,0.134756486516246,
11.8283977830178));
#14576=CARTESIAN_POINT('Ctrl Pts',(-4.37861013558601,0.139584989063466,
11.8295332346106));
#14577=CARTESIAN_POINT('Ctrl Pts',(-4.37716840812328,0.142775051211099,
11.8301075639033));
#14578=CARTESIAN_POINT('Ctrl Pts',(-4.37641616631218,0.144611204644327,
11.8303632616803));
#14579=CARTESIAN_POINT('Ctrl Pts',(-4.37596057093255,0.14586216270989,11.830479908078));
#14580=CARTESIAN_POINT('Ctrl Pts',(-4.39990749973883,0.131433504422785,
11.8105861003151));
#14581=CARTESIAN_POINT('Ctrl Pts',(-4.3978421585968,0.134197554896133,11.8118993900741));
#14582=CARTESIAN_POINT('Ctrl Pts',(-4.39446005348131,0.138892971386962,
11.8140046108773));
#14583=CARTESIAN_POINT('Ctrl Pts',(-4.39064941066155,0.144825508674648,
11.8162052857216));
#14584=CARTESIAN_POINT('Ctrl Pts',(-4.38858693511445,0.14845239833212,11.817285750215));
#14585=CARTESIAN_POINT('Ctrl Pts',(-4.38748854871073,0.150590557851844,
11.8178062692381));
#14586=CARTESIAN_POINT('Ctrl Pts',(-4.3869775568074,0.151688294341147,11.8180210706515));
#14587=CARTESIAN_POINT('Ctrl Pts',(-4.38674149675009,0.152249769834917,
11.8181058720862));
#14588=CARTESIAN_POINT('',(-4.2841165028712,0.108864535984968,11.8201045080524));
#14589=CARTESIAN_POINT('Ctrl Pts',(-4.2998985866006,0.064078396601051,11.7953338759064));
#14590=CARTESIAN_POINT('Ctrl Pts',(-4.29821195997181,0.0679078725578545,
11.7984345883761));
#14591=CARTESIAN_POINT('Ctrl Pts',(-4.29531934379238,0.0747519942657476,
11.8037156359142));
#14592=CARTESIAN_POINT('Ctrl Pts',(-4.2912761668828,0.0857111829491446,
11.8105333018319));
#14593=CARTESIAN_POINT('Ctrl Pts',(-4.28845382290292,0.0942165736780995,
11.8148613164417));
#14594=CARTESIAN_POINT('Ctrl Pts',(-4.2864128668125,0.100856657618271,11.8176056635397));
#14595=CARTESIAN_POINT('Ctrl Pts',(-4.28514086404414,0.105200715903957,
11.8191332343535));
#14596=CARTESIAN_POINT('Ctrl Pts',(-4.28411650287131,0.108864535984662,
11.8201045080524));
#14597=CARTESIAN_POINT('Origin',(-4.33141800137305,0.137425883926612,11.7622528214458));
#14598=CARTESIAN_POINT('Ctrl Pts',(-4.3311987144153,-0.00670693054967494,
11.638842338191));
#14599=CARTESIAN_POINT('Ctrl Pts',(-4.32865175517181,-0.00423844336129769,
11.6757969496053));
#14600=CARTESIAN_POINT('Ctrl Pts',(-4.32053855991217,0.0128128759699999,
11.7357728410368));
#14601=CARTESIAN_POINT('Ctrl Pts',(-4.30180491658975,0.060867221367586,
11.7992439240354));
#14602=CARTESIAN_POINT('Ctrl Pts',(-4.28926759889689,0.0944043425441492,
11.8171772285701));
#14603=CARTESIAN_POINT('Ctrl Pts',(-4.28411650287131,0.108864535984677,
11.8201045080524));
#14604=CARTESIAN_POINT('Ctrl Pts',(-4.32340379388905,0.000847827738124409,
11.638842338191));
#14605=CARTESIAN_POINT('Ctrl Pts',(-4.31988349734736,0.00359272330750201,
11.6744199079636));
#14606=CARTESIAN_POINT('Ctrl Pts',(-4.31012377341186,0.0204532503036035,
11.7318681580362));
#14607=CARTESIAN_POINT('Ctrl Pts',(-4.28935754019246,0.0661213671384488,
11.7913563224866));
#14608=CARTESIAN_POINT('Ctrl Pts',(-4.2761201452253,0.096359272667129,11.8069169849178));
#14609=CARTESIAN_POINT('Ctrl Pts',(-4.27107064996794,0.108365776698791,
11.8091915396309));
#14610=CARTESIAN_POINT('Ctrl Pts',(-4.30157877347568,0.0147332594892646,
11.638842338191));
#14611=CARTESIAN_POINT('Ctrl Pts',(-4.2953386362925,0.0173336386664227,
11.6716031387927));
#14612=CARTESIAN_POINT('Ctrl Pts',(-4.28103898314758,0.0323127313395658,
11.724213122074));
#14613=CARTESIAN_POINT('Ctrl Pts',(-4.25429940326487,0.0709362647361591,
11.7778555072083));
#14614=CARTESIAN_POINT('Ctrl Pts',(-4.23840934345728,0.0944555394156121,
11.7911968100006));
#14615=CARTESIAN_POINT('Ctrl Pts',(-4.23285157171247,0.102524661495376,
11.7931703698428));
#14616=CARTESIAN_POINT('Ctrl Pts',(-4.27543328147234,0.0171451713454814,
11.638842338191));
#14617=CARTESIAN_POINT('Ctrl Pts',(-4.26664745710568,0.0173596858998116,
11.670251961572));
#14618=CARTESIAN_POINT('Ctrl Pts',(-4.2487117108702,0.0266051976481541,
11.722201613145));
#14619=CARTESIAN_POINT('Ctrl Pts',(-4.2184725963509,0.0562721118852402,
11.7810985911187));
#14620=CARTESIAN_POINT('Ctrl Pts',(-4.20102503055697,0.0781925592767865,
11.8019661605246));
#14621=CARTESIAN_POINT('Ctrl Pts',(-4.19434863166431,0.0884303231042628,
11.8069260082108));
#14622=CARTESIAN_POINT('Ctrl Pts',(-4.26119373042795,0.0145528918841497,
11.638842338191));
#14623=CARTESIAN_POINT('Ctrl Pts',(-4.2515576859341,0.0127986708309713,
11.670082443596));
#14624=CARTESIAN_POINT('Ctrl Pts',(-4.23284451070938,0.0179955453015912,
11.7229716250566));
#14625=CARTESIAN_POINT('Ctrl Pts',(-4.20334790059126,0.0435290176544484,
11.7880179360481));
#14626=CARTESIAN_POINT('Ctrl Pts',(-4.18652333699586,0.0670043771977565,
11.8149459781635));
#14627=CARTESIAN_POINT('Ctrl Pts',(-4.17955578083775,0.0803031880431222,
11.8220868710498));
#14628=CARTESIAN_POINT('',(-4.17955578083768,0.080303188043321,11.8220868710499));
#14629=CARTESIAN_POINT('Ctrl Pts',(-4.26119373042795,0.0145528918841497,
11.638842338191));
#14630=CARTESIAN_POINT('Ctrl Pts',(-4.2515576859341,0.0127986708309713,
11.670082443596));
#14631=CARTESIAN_POINT('Ctrl Pts',(-4.23284451070938,0.0179955453015912,
11.7229716250566));
#14632=CARTESIAN_POINT('Ctrl Pts',(-4.20334819884833,0.0435287594709281,
11.7880172783277));
#14633=CARTESIAN_POINT('Ctrl Pts',(-4.18652393242557,0.0670035463958563,
11.8149450251635));
#14634=CARTESIAN_POINT('Ctrl Pts',(-4.17955652059904,0.0803017760943429,
11.8220861128668));
#14635=CARTESIAN_POINT('Origin',(-4.2368150043693,0.0803031880435051,11.8779561946592));
#14636=CARTESIAN_POINT('Ctrl Pts',(-4.25298213616247,0.198467231410946,
11.8394929583522));
#14637=CARTESIAN_POINT('Ctrl Pts',(-4.2286257884895,0.267808752164977,11.8547475451914));
#14638=CARTESIAN_POINT('Ctrl Pts',(-4.20375550827876,0.336898704931691,
11.8704997107853));
#14639=CARTESIAN_POINT('Ctrl Pts',(-4.17831101056731,0.405641108349178,
11.8866997463764));
#14640=CARTESIAN_POINT('Ctrl Pts',(-4.26764395882653,0.202972445897108,
11.8508559827845));
#14641=CARTESIAN_POINT('Ctrl Pts',(-4.24322404174216,0.272657752950044,
11.8641477704669));
#14642=CARTESIAN_POINT('Ctrl Pts',(-4.21791862804,0.341979351501413,11.8780814874676));
#14643=CARTESIAN_POINT('Ctrl Pts',(-4.19175410711448,0.410851995456146,
11.892562174259));
#14644=CARTESIAN_POINT('Ctrl Pts',(-4.30407807870002,0.216966069077792,
11.862230432717));
#14645=CARTESIAN_POINT('Ctrl Pts',(-4.27759840717805,0.286590344056463,
11.8724273890985));
#14646=CARTESIAN_POINT('Ctrl Pts',(-4.24997131879908,0.355728405406215,
11.8835722239453));
#14647=CARTESIAN_POINT('Ctrl Pts',(-4.22116750718431,0.424212414426285,
11.8957681405415));
#14648=CARTESIAN_POINT('Ctrl Pts',(-4.3369990180675,0.234073734275867,11.8456124354964));
#14649=CARTESIAN_POINT('Ctrl Pts',(-4.3077197084613,0.303022130841672,11.8562178951535));
#14650=CARTESIAN_POINT('Ctrl Pts',(-4.27744040849402,0.371404354559313,
11.8680190687516));
#14651=CARTESIAN_POINT('Ctrl Pts',(-4.24596884413302,0.439041104136474,
11.8809722029021));
#14652=CARTESIAN_POINT('Ctrl Pts',(-4.34855965130146,0.24132741635741,11.8322680295746));
#14653=CARTESIAN_POINT('Ctrl Pts',(-4.31851137785818,0.310100961669604,
11.8437509230397));
#14654=CARTESIAN_POINT('Ctrl Pts',(-4.28743292633124,0.378248514869065,
11.8563834756258));
#14655=CARTESIAN_POINT('Ctrl Pts',(-4.25516769303209,0.445602794179394,
11.8702702241066));
#14656=CARTESIAN_POINT('',(-4.17831869257478,0.405606437847502,11.8867128997031));
#14657=CARTESIAN_POINT('Origin',(-4.20023746323962,0.430852097115001,11.8140111108424));
#14658=CARTESIAN_POINT('',(-4.25297464465416,0.19849748388496,11.8395016149463));
#14659=CARTESIAN_POINT('Origin',(-4.29328772795413,0.226549903216342,11.7763516578244));
#14660=CARTESIAN_POINT('Ctrl Pts',(-4.25297464465415,0.198497483885009,
11.8395016149464));
#14661=CARTESIAN_POINT('Ctrl Pts',(-4.23691634103563,0.244214515550849,
11.8495588444424));
#14662=CARTESIAN_POINT('Ctrl Pts',(-4.22062846601348,0.289815884959662,
11.859850949835));
#14663=CARTESIAN_POINT('Ctrl Pts',(-4.20410226715093,0.335282633479534,
11.8703374283436));
#14664=CARTESIAN_POINT('Ctrl Pts',(-4.19556935771983,0.358758306891982,
11.8757518719255));
#14665=CARTESIAN_POINT('Ctrl Pts',(-4.18697273257692,0.382197862800513,
11.8812189300755));
#14666=CARTESIAN_POINT('Ctrl Pts',(-4.17831110315985,0.405597624417347,
11.8867383703356));
#14667=CARTESIAN_POINT('Ctrl Pts',(-4.17832438065528,0.405613001090449,
11.8866940169724));
#14668=CARTESIAN_POINT('Ctrl Pts',(-4.17353003744589,0.418565725487248,
11.8897464020236));
#14669=CARTESIAN_POINT('Ctrl Pts',(-4.16871489377343,0.431505611461712,
11.8928150545396));
#14670=CARTESIAN_POINT('Ctrl Pts',(-4.16387784115802,0.444431102132758,
11.8959002913408));
#14671=CARTESIAN_POINT('Ctrl Pts',(-4.19176708001533,0.410823686905363,
11.8925562479089));
#14672=CARTESIAN_POINT('Ctrl Pts',(-4.18683712032951,0.423800954990201,
11.8952847659635));
#14673=CARTESIAN_POINT('Ctrl Pts',(-4.18187186452005,0.436758289002851,
11.898043001497));
#14674=CARTESIAN_POINT('Ctrl Pts',(-4.17687624823759,0.449699275767736,
11.9008161302017));
#14675=CARTESIAN_POINT('Ctrl Pts',(-4.22117628298598,0.424185231737969,
11.8957460251486));
#14676=CARTESIAN_POINT('Ctrl Pts',(-4.21574899813179,0.43708928465133,11.8980438924075));
#14677=CARTESIAN_POINT('Ctrl Pts',(-4.21027895401589,0.449969857826206,
11.9003772371141));
#14678=CARTESIAN_POINT('Ctrl Pts',(-4.20476498303276,0.462824517622096,
11.9027501529791));
#14679=CARTESIAN_POINT('Ctrl Pts',(-4.2459821724517,0.439012459536339,11.8809667172436));
#14680=CARTESIAN_POINT('Ctrl Pts',(-4.24005221860176,0.451756844238467,
11.883407410326));
#14681=CARTESIAN_POINT('Ctrl Pts',(-4.23408529886524,0.464475341488486,
11.8858987952752));
#14682=CARTESIAN_POINT('Ctrl Pts',(-4.22806909913246,0.477163666032771,
11.8884288073028));
#14683=CARTESIAN_POINT('Ctrl Pts',(-4.2551813574745,0.445574269204196,11.8702643430631));
#14684=CARTESIAN_POINT('Ctrl Pts',(-4.24910188448058,0.45826545703258,11.8728808695122));
#14685=CARTESIAN_POINT('Ctrl Pts',(-4.24297931347368,0.47092779002261,11.8755428064202));
#14686=CARTESIAN_POINT('Ctrl Pts',(-4.2368109319615,0.483558887244307,11.8782524024265));
#14687=CARTESIAN_POINT('',(-4.16387023623629,0.44442096356818,11.8959309387847));
#14688=CARTESIAN_POINT('Origin',(-4.18196216438191,0.468862204265513,11.821899760923));
#14689=CARTESIAN_POINT('Ctrl Pts',(-4.17832438065528,0.405613001090449,
11.8866940169724));
#14690=CARTESIAN_POINT('Ctrl Pts',(-4.17353003744589,0.418565725487248,
11.8897464020236));
#14691=CARTESIAN_POINT('Ctrl Pts',(-4.16871489377343,0.431505611461712,
11.8928150545396));
#14692=CARTESIAN_POINT('Ctrl Pts',(-4.16387784115802,0.444431102132758,
11.8959002913408));
#14693=CARTESIAN_POINT('Ctrl Pts',(-4.28411650287118,0.108864535985058,
11.8201045080525));
#14694=CARTESIAN_POINT('Ctrl Pts',(-4.27383348446592,0.138789589880342,
11.8264707476279));
#14695=CARTESIAN_POINT('Ctrl Pts',(-4.26345245300614,0.168667789068198,
11.8329394197285));
#14696=CARTESIAN_POINT('Ctrl Pts',(-4.25297464465416,0.198497483884985,
11.8395016149463));
#14697=CARTESIAN_POINT('Ctrl Pts',(-4.30077643513154,0.113467717919639,
11.835998821523));
#14698=CARTESIAN_POINT('Ctrl Pts',(-4.29061215932074,0.143598492746439,
11.841360239256));
#14699=CARTESIAN_POINT('Ctrl Pts',(-4.28023908095909,0.173646869395274,
11.8468941305194));
#14700=CARTESIAN_POINT('Ctrl Pts',(-4.26973042744931,0.203646502026694,
11.8524853083802));
#14701=CARTESIAN_POINT('Ctrl Pts',(-4.34104542870178,0.128332090592554,
11.8495698235112));
#14702=CARTESIAN_POINT('Ctrl Pts',(-4.32996580556451,0.158437379738818,
11.8535197351198));
#14703=CARTESIAN_POINT('Ctrl Pts',(-4.31867086063058,0.18845912219569,11.8576528974894));
#14704=CARTESIAN_POINT('Ctrl Pts',(-4.30715498164588,0.218382296444562,
11.8619899386228));
#14705=CARTESIAN_POINT('Ctrl Pts',(-4.37596057093238,0.145862162710285,
11.8304799080781));
#14706=CARTESIAN_POINT('Ctrl Pts',(-4.36371043865105,0.175725323285883,
11.8346706366403));
#14707=CARTESIAN_POINT('Ctrl Pts',(-4.35128087581798,0.20549030245879,11.8390867979876));
#14708=CARTESIAN_POINT('Ctrl Pts',(-4.33863808356346,0.235139180415304,
11.8437106389784));
#14709=CARTESIAN_POINT('Ctrl Pts',(-4.38674149674992,0.152249769835312,
11.8181058720863));
#14710=CARTESIAN_POINT('Ctrl Pts',(-4.37420531076058,0.182067441230975,
11.8226093301053));
#14711=CARTESIAN_POINT('Ctrl Pts',(-4.36147336656485,0.211771272545564,
11.8273329847674));
#14712=CARTESIAN_POINT('Ctrl Pts',(-4.34854691846783,0.241356558688859,
11.8322728954492));
#14713=CARTESIAN_POINT('Origin',(2.32049299786841,-3.62262617981002,18.6886752212914));
#14714=CARTESIAN_POINT('Ctrl Pts',(-4.16387784115802,0.444431102132757,
11.8959002913408));
#14715=CARTESIAN_POINT('Ctrl Pts',(-4.15828181192265,0.459384717366581,
11.8994696292642));
#14716=CARTESIAN_POINT('Ctrl Pts',(-4.15265646004605,0.474319169743533,
11.9030611537802));
#14717=CARTESIAN_POINT('Ctrl Pts',(-4.14699952201194,0.489230927920841,
11.90667591896));
#14718=CARTESIAN_POINT('Ctrl Pts',(-4.17687624823759,0.449699275767735,
11.9008161302017));
#14719=CARTESIAN_POINT('Ctrl Pts',(-4.17109677528411,0.464670818570484,
11.9040243874894));
#14720=CARTESIAN_POINT('Ctrl Pts',(-4.16526996333276,0.47961431758977,11.9072712243025));
#14721=CARTESIAN_POINT('Ctrl Pts',(-4.15939846344752,0.49453108177116,11.9105424838858));
#14722=CARTESIAN_POINT('Ctrl Pts',(-4.20476498083012,0.462824518205306,
11.9027501451694));
#14723=CARTESIAN_POINT('Ctrl Pts',(-4.19838581870849,0.477696188569049,
11.9054953926599));
#14724=CARTESIAN_POINT('Ctrl Pts',(-4.19194742237,0.492533642599708,11.9082903960795));
#14725=CARTESIAN_POINT('Ctrl Pts',(-4.18544686834643,0.507332016553614,
11.9111411005044));
#14726=CARTESIAN_POINT('Ctrl Pts',(-4.22806909913247,0.477163666032769,
11.8884288073027));
#14727=CARTESIAN_POINT('Ctrl Pts',(-4.221108904099,0.491842901663036,11.8913558007423));
#14728=CARTESIAN_POINT('Ctrl Pts',(-4.21409456216484,0.506484223480552,
11.8943508066784));
#14729=CARTESIAN_POINT('Ctrl Pts',(-4.20701096015312,0.521080619220583,
11.8974040141978));
#14730=CARTESIAN_POINT('Ctrl Pts',(-4.23681093196151,0.483558887244306,
11.8782524024265));
#14731=CARTESIAN_POINT('Ctrl Pts',(-4.22967467647256,0.498171916075573,
11.8813871581699));
#14732=CARTESIAN_POINT('Ctrl Pts',(-4.22247713691368,0.512743255380418,
11.8845856560674));
#14733=CARTESIAN_POINT('Ctrl Pts',(-4.21521271352384,0.527267762951524,
11.8878527735462));
#14734=CARTESIAN_POINT('Ctrl Pts',(-4.16386860738941,0.444418764937274,
11.8959375572369));
#14735=CARTESIAN_POINT('Ctrl Pts',(-4.16391834371126,0.4445411940699,11.8959904740987));
#14736=CARTESIAN_POINT('Ctrl Pts',(-4.163968157019,0.444663693166018,11.8960431989357));
#14737=CARTESIAN_POINT('Ctrl Pts',(-4.16401805752376,0.444786241611601,
11.8960957271683));
#14738=CARTESIAN_POINT('Ctrl Pts',(-4.16561890128454,0.448717683096392,
11.8977808703098));
#14739=CARTESIAN_POINT('Ctrl Pts',(-4.16724284026456,0.452546011395253,
11.899195612021));
#14740=CARTESIAN_POINT('Ctrl Pts',(-4.16886553453554,0.456301479369417,
11.9004052791275));
#14741=CARTESIAN_POINT('Ctrl Pts',(-4.16924869277134,0.457188238205828,
11.9006909114384));
#14742=CARTESIAN_POINT('Ctrl Pts',(-4.16963159810811,0.458070820883551,
11.9009650379668));
#14743=CARTESIAN_POINT('Ctrl Pts',(-4.17001364086649,0.45894930734541,11.9012282802084));
#14744=CARTESIAN_POINT('Ctrl Pts',(-4.17055703829997,0.460198820072074,
11.9016027020638));
#14745=CARTESIAN_POINT('Ctrl Pts',(-4.17109864146052,0.461440173594932,
11.9019550639622));
#14746=CARTESIAN_POINT('Ctrl Pts',(-4.17163327228824,0.46268105659674,11.9022825344791));
#14747=CARTESIAN_POINT('Ctrl Pts',(-4.17269401152293,0.465143041984486,
11.9029322553846));
#14748=CARTESIAN_POINT('Ctrl Pts',(-4.17374475353427,0.467580949994859,
11.9034907549559));
#14749=CARTESIAN_POINT('Ctrl Pts',(-4.17476688820595,0.4700231092791,11.9039700966035));
#14750=CARTESIAN_POINT('Ctrl Pts',(-4.17534733062492,0.471409944968901,
11.9042423016594));
#14751=CARTESIAN_POINT('Ctrl Pts',(-4.17591872561242,0.472797307639367,
11.9044893141433));
#14752=CARTESIAN_POINT('Ctrl Pts',(-4.17647934282577,0.474183601581782,
11.9047162802904));
#14753=CARTESIAN_POINT('Ctrl Pts',(-4.17651181682008,0.47426390325737,11.9047294274025));
#14754=CARTESIAN_POINT('Ctrl Pts',(-4.17654425502559,0.474344199989393,
11.9047425078853));
#14755=CARTESIAN_POINT('Ctrl Pts',(-4.17657665727905,0.474424489992879,
11.9047555221994));
#14756=CARTESIAN_POINT('Ctrl Pts',(-4.17794092023881,0.47780501653376,11.9053034762694));
#14757=CARTESIAN_POINT('Ctrl Pts',(-4.17923643699538,0.48119604508226,11.9057257123795));
#14758=CARTESIAN_POINT('Ctrl Pts',(-4.18044332363875,0.484607579902023,
11.9060319457311));
#14759=CARTESIAN_POINT('Ctrl Pts',(-4.18153051926195,0.487680781303985,
11.9063078088881));
#14760=CARTESIAN_POINT('Ctrl Pts',(-4.1825475622151,0.490770285934714,11.9064918264379));
#14761=CARTESIAN_POINT('Ctrl Pts',(-4.18349249663733,0.493896424319563,
11.9066042613417));
#14762=CARTESIAN_POINT('Ctrl Pts',(-4.18440502081064,0.496915339471953,
11.9067128398475));
#14763=CARTESIAN_POINT('Ctrl Pts',(-4.18524674175396,0.499965615042457,
11.9067514773718));
#14764=CARTESIAN_POINT('Ctrl Pts',(-4.18601047565315,0.503059942136878,
11.9067297730278));
#14765=CARTESIAN_POINT('Ctrl Pts',(-4.18604651909286,0.503205974926828,
11.9067287487192));
#14766=CARTESIAN_POINT('Ctrl Pts',(-4.18608238856455,0.503352107249628,
11.9067275884811));
#14767=CARTESIAN_POINT('Ctrl Pts',(-4.18611808342164,0.50349833985629,11.9067262938402));
#14768=CARTESIAN_POINT('Ctrl Pts',(-4.18637628476887,0.504556124062116,
11.9067169289611));
#14769=CARTESIAN_POINT('Ctrl Pts',(-4.1866253519351,0.505619124128795,11.9067005504272));
#14770=CARTESIAN_POINT('Ctrl Pts',(-4.18686494960606,0.506687549510347,
11.9066776046077));
#14771=CARTESIAN_POINT('Ctrl Pts',(-4.18706148986136,0.507563971206857,
11.9066587823162));
#14772=CARTESIAN_POINT('Ctrl Pts',(-4.18725052829967,0.508439469984838,
11.9066356211609));
#14773=CARTESIAN_POINT('Ctrl Pts',(-4.1874280189678,0.50930672791011,11.9066032159468));
#14774=CARTESIAN_POINT('Ctrl Pts',(-4.28411650287119,0.108864535985059,
11.8201045080525));
#14775=CARTESIAN_POINT('Ctrl Pts',(-4.27608425813253,0.138890274178381,
11.8283607642014));
#14776=CARTESIAN_POINT('Ctrl Pts',(-4.26805801086052,0.168913049189128,
11.8366050116627));
#14777=CARTESIAN_POINT('Ctrl Pts',(-4.26003736024089,0.198935548997806,
11.8448257475953));
#14778=CARTESIAN_POINT('Ctrl Pts',(-4.26672203233337,0.10819952360388,11.8055538834905));
#14779=CARTESIAN_POINT('Ctrl Pts',(-4.25869817607788,0.138222655883494,
11.8138093209203));
#14780=CARTESIAN_POINT('Ctrl Pts',(-4.25068357204439,0.168242310003863,
11.8220515500891));
#14781=CARTESIAN_POINT('Ctrl Pts',(-4.2426781599081,0.198260104377667,11.8302708366033));
#14782=CARTESIAN_POINT('Ctrl Pts',(-4.22594174945398,0.1006372010266,11.793301386559));
#14783=CARTESIAN_POINT('Ctrl Pts',(-4.21793377436576,0.130663341317267,
11.8015463165459));
#14784=CARTESIAN_POINT('Ctrl Pts',(-4.20994143979378,0.160686561995819,
11.8097749635335));
#14785=CARTESIAN_POINT('Ctrl Pts',(-4.20196492133035,0.190709798308366,
11.8179752139256));
#14786=CARTESIAN_POINT('Ctrl Pts',(-4.19065041895756,0.0863985393393625,
11.8107162239207));
#14787=CARTESIAN_POINT('Ctrl Pts',(-4.18264086798039,0.116436218388614,
11.8189393524712));
#14788=CARTESIAN_POINT('Ctrl Pts',(-4.17464603081676,0.146475576888081,
11.8271373943832));
#14789=CARTESIAN_POINT('Ctrl Pts',(-4.16666679209685,0.176519661076779,
11.8352979905427));
#14790=CARTESIAN_POINT('Ctrl Pts',(-4.17955578083765,0.0803031880435048,
11.8220868710499));
#14791=CARTESIAN_POINT('Ctrl Pts',(-4.1715408983818,0.110345789757979,11.8303011452969));
#14792=CARTESIAN_POINT('Ctrl Pts',(-4.1635389344325,0.140392086225485,11.8384867715752));
#14793=CARTESIAN_POINT('Ctrl Pts',(-4.15555007706065,0.170445064553628,
11.8466312332458));
#14794=CARTESIAN_POINT('',(-4.15555007706065,0.170445064553628,11.8466312332458));
#14795=CARTESIAN_POINT('Origin',(-16.9242493907379,13.7717485420172,-25.8067217625208));
#14796=CARTESIAN_POINT('Origin',(-4.21266156135419,0.170445064553628,11.9026515720683));
#14797=CARTESIAN_POINT('Origin',(-4.1,0.9,6.5));
#14798=CARTESIAN_POINT('',(-4.10062628980501,2.179093092077E-7,3.09201395474528));
#14799=CARTESIAN_POINT('Ctrl Pts',(-4.10062628985477,2.17910570921021E-7,
3.09201395473902));
#14800=CARTESIAN_POINT('Ctrl Pts',(-4.10946509570597,6.36863920784053E-6,
3.16223612469626));
#14801=CARTESIAN_POINT('Ctrl Pts',(-4.11980376888638,8.0145983837535E-5,
3.23266996300447));
#14802=CARTESIAN_POINT('Ctrl Pts',(-4.13221833032745,0.000519669739900586,
3.30274456732768));
#14803=CARTESIAN_POINT('Ctrl Pts',(-4.1427684836723,0.000893186198551402,
3.36229542820175));
#14804=CARTESIAN_POINT('Ctrl Pts',(-4.15482146373736,0.00153084307074809,
3.42158490272002));
#14805=CARTESIAN_POINT('Ctrl Pts',(-4.16871245653638,0.0026156074478858,
3.480242356807));
#14806=CARTESIAN_POINT('Ctrl Pts',(-4.17290633342143,0.00294311235072616,
3.49795182828901));
#14807=CARTESIAN_POINT('Ctrl Pts',(-4.17726742698064,0.0033113718635993,
3.51560363027309));
#14808=CARTESIAN_POINT('Ctrl Pts',(-4.18180390848863,0.0037254212262936,
3.53318749645313));
#14809=CARTESIAN_POINT('Ctrl Pts',(-4.19639560025769,0.00505722003710435,
3.58974638574991));
#14810=CARTESIAN_POINT('Ctrl Pts',(-4.21284049567206,0.0068867784862876,
3.64574064454163));
#14811=CARTESIAN_POINT('Ctrl Pts',(-4.23143875004913,0.00963952341296004,
3.70094503351942));
#14812=CARTESIAN_POINT('Ctrl Pts',(-4.24030470587491,0.0109517817800476,
3.72726146430606));
#14813=CARTESIAN_POINT('Ctrl Pts',(-4.24965932888634,0.0124738356593051,
3.75339825043382));
#14814=CARTESIAN_POINT('Ctrl Pts',(-4.25953080556008,0.014251772749529,
3.77933080745784));
#14815=CARTESIAN_POINT('Ctrl Pts',(-4.27693923829638,0.0173871798692027,
3.82506309144671));
#14816=CARTESIAN_POINT('Ctrl Pts',(-4.29591937405777,0.0213206157856711,
3.87005702106385));
#14817=CARTESIAN_POINT('Ctrl Pts',(-4.31656055867041,0.026441281981235,
3.9141641214968));
#14818=CARTESIAN_POINT('Ctrl Pts',(-4.32190785897979,0.0277678405313199,
3.92559049630121));
#14819=CARTESIAN_POINT('Ctrl Pts',(-4.32736638333248,0.0291740764308477,
3.93695744733596));
#14820=CARTESIAN_POINT('Ctrl Pts',(-4.33293714059227,0.0306667563398393,
3.94826261099145));
#14821=CARTESIAN_POINT('',(-4.1,2.23481172803575E-17,3.08202325217327));
#14822=CARTESIAN_POINT('Origin',(-4.18002610983571,4.86909770516006E-5,
3.08202161556327));
#14823=CARTESIAN_POINT('',(-4.1,0.,11.7890187209227));
#14824=CARTESIAN_POINT('',(-4.1,0.,-0.5));
#14825=CARTESIAN_POINT('Ctrl Pts',(-4.26119373042794,0.014552891884149,
11.638842338191));
#14826=CARTESIAN_POINT('Ctrl Pts',(-4.20740273136266,0.00476035687747917,
11.6883109569019));
#14827=CARTESIAN_POINT('Ctrl Pts',(-4.15394513638752,2.66182811039857E-16,
11.7388892266742));
#14828=CARTESIAN_POINT('Ctrl Pts',(-4.1,0.,11.7890187209227));
#14829=CARTESIAN_POINT('Ctrl Pts',(-4.25297464465415,0.198497483885009,
11.8395016149464));
#14830=CARTESIAN_POINT('Ctrl Pts',(-4.23432610916137,0.268350649999046,
11.8586270490361));
#14831=CARTESIAN_POINT('Ctrl Pts',(-4.21571553863559,0.338200359108088,
11.877624289993));
#14832=CARTESIAN_POINT('Ctrl Pts',(-4.19713727273351,0.408083416458755,
11.8963406005087));
#14833=CARTESIAN_POINT('Ctrl Pts',(-4.23780121350118,0.19723139322301,11.8292529191487));
#14834=CARTESIAN_POINT('Ctrl Pts',(-4.2191816325323,0.267079242619096,11.8483714100219));
#14835=CARTESIAN_POINT('Ctrl Pts',(-4.20061568185391,0.336921901139932,
11.8673561360113));
#14836=CARTESIAN_POINT('Ctrl Pts',(-4.18209944631418,0.406793934797266,
11.886058258236));
#14837=CARTESIAN_POINT('Ctrl Pts',(-4.20089925437152,0.190087479799487,
11.8192080583286));
#14838=CARTESIAN_POINT('Ctrl Pts',(-4.1823370650831,0.259947915222703,11.8382842185072));
#14839=CARTESIAN_POINT('Ctrl Pts',(-4.16386011311889,0.329808442959132,
11.8572064988123));
#14840=CARTESIAN_POINT('Ctrl Pts',(-4.14546763523864,0.399706853583148,
11.8758191065186));
#14841=CARTESIAN_POINT('Ctrl Pts',(-4.16755381812912,0.17700436588702,11.8343936873133));
#14842=CARTESIAN_POINT('Ctrl Pts',(-4.14898961110941,0.246909238451779,
11.8533850386243));
#14843=CARTESIAN_POINT('Ctrl Pts',(-4.1305071888592,0.31683856296458,11.8721748641617));
#14844=CARTESIAN_POINT('Ctrl Pts',(-4.11211341232255,0.386829622935632,
11.8906052241705));
#14845=CARTESIAN_POINT('Ctrl Pts',(-4.15555007706064,0.170445064553676,
11.8466312332458));
#14846=CARTESIAN_POINT('Ctrl Pts',(-4.13696158210585,0.240372415866411,
11.8655817887042));
#14847=CARTESIAN_POINT('Ctrl Pts',(-4.11844401855589,0.310335983331864,
11.8843096665637));
#14848=CARTESIAN_POINT('Ctrl Pts',(-4.1,0.380373905065778,11.9026515720683));
#14849=CARTESIAN_POINT('',(-4.1,0.380373905065777,11.9026515720683));
#14850=CARTESIAN_POINT('Ctrl Pts',(-4.15555007706064,0.170445064553676,
11.8466312332458));
#14851=CARTESIAN_POINT('Ctrl Pts',(-4.13696158210585,0.240372415866411,
11.8655817887042));
#14852=CARTESIAN_POINT('Ctrl Pts',(-4.11844401855589,0.310335983331864,
11.8843096665637));
#14853=CARTESIAN_POINT('Ctrl Pts',(-4.1,0.380373905065778,11.9026515720683));
#14854=CARTESIAN_POINT('Origin',(-4.15641129807095,0.380373905065777,11.9593769231025));
#14855=CARTESIAN_POINT('Ctrl Pts',(-4.08957475120669,0.420000000000004,
11.9129846529869));
#14856=CARTESIAN_POINT('Ctrl Pts',(-4.09304720501634,0.406788497264506,
11.9095547476558));
#14857=CARTESIAN_POINT('Ctrl Pts',(-4.09652229439691,0.393579881415503,
11.90611002378));
#14858=CARTESIAN_POINT('Ctrl Pts',(-4.1,0.380373905065779,11.9026515720683));
#14859=CARTESIAN_POINT('Ctrl Pts',(-4.09935159372593,0.425175588381722,
11.9033276075325));
#14860=CARTESIAN_POINT('Ctrl Pts',(-4.10281576552394,0.411971887580064,
11.8998828402856));
#14861=CARTESIAN_POINT('Ctrl Pts',(-4.10628316887034,0.398770707124635,
11.8964240952639));
#14862=CARTESIAN_POINT('Ctrl Pts',(-4.10975331598555,0.385571833991309,
11.892952254123));
#14863=CARTESIAN_POINT('Ctrl Pts',(-4.12472484253256,0.435512908316209,
11.8899576288478));
#14864=CARTESIAN_POINT('Ctrl Pts',(-4.12818546048421,0.422324742310494,
11.886482228227));
#14865=CARTESIAN_POINT('Ctrl Pts',(-4.13164915696943,0.409138427226951,
11.8829942449745));
#14866=CARTESIAN_POINT('Ctrl Pts',(-4.13511596185361,0.395953697471928,
11.8794947521918));
#14867=CARTESIAN_POINT('Ctrl Pts',(-4.15423485006789,0.44280432443085,11.892284208906));
#14868=CARTESIAN_POINT('Ctrl Pts',(-4.15771124289688,0.429624324733392,
11.8887884960684));
#14869=CARTESIAN_POINT('Ctrl Pts',(-4.16118998038772,0.416445694643035,
11.8852813895583));
#14870=CARTESIAN_POINT('Ctrl Pts',(-4.16467098162167,0.403268395711099,
11.8817635071735));
#14871=CARTESIAN_POINT('Ctrl Pts',(-4.16786079472921,0.445145811119343,
11.8972322351616));
#14872=CARTESIAN_POINT('Ctrl Pts',(-4.1713468289151,0.43196686310669,11.8937304736977));
#14873=CARTESIAN_POINT('Ctrl Pts',(-4.17483467940513,0.418789345178509,
11.8902173887752));
#14874=CARTESIAN_POINT('Ctrl Pts',(-4.17832438065533,0.405613001090281,
11.8866940169724));
#14875=CARTESIAN_POINT('',(-4.08957475121441,0.420000000004092,11.9129846529793));
#14876=CARTESIAN_POINT('Ctrl Pts',(-4.1,0.380373905065779,11.9026515720683));
#14877=CARTESIAN_POINT('Ctrl Pts',(-4.09652229439691,0.393579881415503,
11.90611002378));
#14878=CARTESIAN_POINT('Ctrl Pts',(-4.09304720501634,0.406788497264506,
11.9095547476558));
#14879=CARTESIAN_POINT('Ctrl Pts',(-4.08957475120669,0.420000000000004,
11.9129846529869));
#14880=CARTESIAN_POINT('Origin',(-4.14579351793413,0.420000000000002,11.9699008217586));
#14881=CARTESIAN_POINT('Ctrl Pts',(-4.20389723040784,0.448082122854196,
11.9226213021674));
#14882=CARTESIAN_POINT('Ctrl Pts',(-4.20184390702141,0.454587762651284,
11.9239619770498));
#14883=CARTESIAN_POINT('Ctrl Pts',(-4.19793638990807,0.467244934591944,
11.9248776171878));
#14884=CARTESIAN_POINT('Ctrl Pts',(-4.19264636363395,0.486132237432104,
11.9213061489869));
#14885=CARTESIAN_POINT('Ctrl Pts',(-4.18798032404462,0.506067458447531,
11.9109852930588));
#14886=CARTESIAN_POINT('Ctrl Pts',(-4.18528583117895,0.519829640007596,
11.8969505489161));
#14887=CARTESIAN_POINT('Ctrl Pts',(-4.18416745800402,0.52598322777095,11.8885969417624));
#14888=CARTESIAN_POINT('Ctrl Pts',(-4.19174908380885,0.448683750825517,
11.9080492965203));
#14889=CARTESIAN_POINT('Ctrl Pts',(-4.18980989453422,0.453995201447333,
11.9090114292076));
#14890=CARTESIAN_POINT('Ctrl Pts',(-4.18629251150101,0.463929335183028,
11.9094067500189));
#14891=CARTESIAN_POINT('Ctrl Pts',(-4.18220013538096,0.477785316871903,
11.9066119377239));
#14892=CARTESIAN_POINT('Ctrl Pts',(-4.17917348866453,0.493275358206986,
11.899219888217));
#14893=CARTESIAN_POINT('Ctrl Pts',(-4.17754427524001,0.505531647607768,
11.8877547429666));
#14894=CARTESIAN_POINT('Ctrl Pts',(-4.1769096978644,0.511201122881534,11.880578516275));
#14895=CARTESIAN_POINT('Ctrl Pts',(-4.16303328561123,0.445542625831325,
11.890845536232));
#14896=CARTESIAN_POINT('Ctrl Pts',(-4.16100917724248,0.449355522427211,
11.8915365465931));
#14897=CARTESIAN_POINT('Ctrl Pts',(-4.15757466275877,0.455975296164343,
11.8916732129521));
#14898=CARTESIAN_POINT('Ctrl Pts',(-4.15465267900733,0.464139333458313,
11.8899004794177));
#14899=CARTESIAN_POINT('Ctrl Pts',(-4.15404544758576,0.474490462284283,
11.885476111969));
#14900=CARTESIAN_POINT('Ctrl Pts',(-4.15452950414342,0.48467806297157,11.8766922820171));
#14901=CARTESIAN_POINT('Ctrl Pts',(-4.15493036552924,0.489633970339022,
11.8707859261611));
#14902=CARTESIAN_POINT('Ctrl Pts',(-4.11911994815048,0.43335877848646,11.8924222558676));
#14903=CARTESIAN_POINT('Ctrl Pts',(-4.11669542890408,0.437016335410973,
11.8938247509459));
#14904=CARTESIAN_POINT('Ctrl Pts',(-4.11252036702983,0.443826518601221,
11.8952537752929));
#14905=CARTESIAN_POINT('Ctrl Pts',(-4.10893178611961,0.453405904273695,
11.89379446554));
#14906=CARTESIAN_POINT('Ctrl Pts',(-4.10901293703883,0.464398928863795,
11.8871965822423));
#14907=CARTESIAN_POINT('Ctrl Pts',(-4.11127193969944,0.473342094480854,
11.8767538807855));
#14908=CARTESIAN_POINT('Ctrl Pts',(-4.11272151139406,0.477535811726914,
11.8702935234762));
#14909=CARTESIAN_POINT('Ctrl Pts',(-4.09799980361865,0.424459988313498,
11.9046628339601));
#14910=CARTESIAN_POINT('Ctrl Pts',(-4.0953727901903,0.428957878019816,11.9068711895671));
#14911=CARTESIAN_POINT('Ctrl Pts',(-4.09066232230966,0.438065597562857,
11.9096177858811));
#14912=CARTESIAN_POINT('Ctrl Pts',(-4.08582024878189,0.452523147275828,
11.9077859527864));
#14913=CARTESIAN_POINT('Ctrl Pts',(-4.08474695018234,0.467269876710216,
11.8974070840654));
#14914=CARTESIAN_POINT('Ctrl Pts',(-4.08693113570529,0.476307270345706,
11.8837903326451));
#14915=CARTESIAN_POINT('Ctrl Pts',(-4.088504487915,0.480216196086898,11.8760208135731));
#14916=CARTESIAN_POINT('Ctrl Pts',(-4.08957475120669,0.420000000000002,
11.9129846529869));
#14917=CARTESIAN_POINT('Ctrl Pts',(-4.08688537940494,0.425116071352305,
11.9156410715272));
#14918=CARTESIAN_POINT('Ctrl Pts',(-4.08194577754747,0.435809942712488,
11.9190952094536));
#14919=CARTESIAN_POINT('Ctrl Pts',(-4.0763463965552,0.453454331933779,11.9169484279061));
#14920=CARTESIAN_POINT('Ctrl Pts',(-4.07432022781093,0.470721130278274,
11.9042829130981));
#14921=CARTESIAN_POINT('Ctrl Pts',(-4.07611770769293,0.48001701618929,11.888710974919));
#14922=CARTESIAN_POINT('Ctrl Pts',(-4.07758517014024,0.483840236412191,
11.8801119543743));
#14923=CARTESIAN_POINT('Ctrl Pts',(-4.08957475120669,0.420000000000002,
11.9129846529869));
#14924=CARTESIAN_POINT('Ctrl Pts',(-4.08688537940494,0.425116071352305,
11.9156410715272));
#14925=CARTESIAN_POINT('Ctrl Pts',(-4.08194577754747,0.435809942712488,
11.9190952094536));
#14926=CARTESIAN_POINT('Ctrl Pts',(-4.0763463965552,0.453454331933779,11.9169484279061));
#14927=CARTESIAN_POINT('Ctrl Pts',(-4.07457762006514,0.468527660380283,
11.9058918636934));
#14928=CARTESIAN_POINT('Ctrl Pts',(-4.07558957056381,0.476670041956566,
11.8939568640326));
#14929=CARTESIAN_POINT('Ctrl Pts',(-4.07626606489887,0.479531832015509,
11.8887931799445));
#14930=CARTESIAN_POINT('Origin',(-4.11158163835162,0.547680472824379,11.9142976877142));
#14931=CARTESIAN_POINT('Ctrl Pts',(-4.16771789344709,0.504034482698269,
11.8776405136582));
#14932=CARTESIAN_POINT('Ctrl Pts',(-4.16747677218029,0.509230674892329,
11.8710844000372));
#14933=CARTESIAN_POINT('Ctrl Pts',(-4.16740198755876,0.514183898751254,
11.8631601154487));
#14934=CARTESIAN_POINT('Ctrl Pts',(-4.16750381345594,0.518518893325527,
11.8542908886285));
#14935=CARTESIAN_POINT('Ctrl Pts',(-4.15716840981065,0.494162146356706,
11.8732397213383));
#14936=CARTESIAN_POINT('Ctrl Pts',(-4.15737066207015,0.49902515398837,11.8672225409494));
#14937=CARTESIAN_POINT('Ctrl Pts',(-4.15774524939355,0.503761760048647,
11.8598165458383));
#14938=CARTESIAN_POINT('Ctrl Pts',(-4.15827955078225,0.507967835497394,
11.8514452383884));
#14939=CARTESIAN_POINT('Ctrl Pts',(-4.12991591613054,0.479256016633343,
11.8684902470024));
#14940=CARTESIAN_POINT('Ctrl Pts',(-4.13102224542203,0.48352297529437,11.8628269450333));
#14941=CARTESIAN_POINT('Ctrl Pts',(-4.13236454521323,0.487741753406994,
11.8558585890896));
#14942=CARTESIAN_POINT('Ctrl Pts',(-4.13387372265488,0.491526065878086,
11.8479575722917));
#14943=CARTESIAN_POINT('Ctrl Pts',(-4.09886149942541,0.47853885680583,11.8732397213383));
#14944=CARTESIAN_POINT('Ctrl Pts',(-4.10035784041994,0.482395955248883,
11.8663776500601));
#14945=CARTESIAN_POINT('Ctrl Pts',(-4.10225093958688,0.485898763965467,
11.8584280339396));
#14946=CARTESIAN_POINT('Ctrl Pts',(-4.10441543782456,0.488897063406756,
11.8498117164234));
#14947=CARTESIAN_POINT('Ctrl Pts',(-4.08478921042867,0.481813809054108,
11.8776405136582));
#14948=CARTESIAN_POINT('Ctrl Pts',(-4.08624010985666,0.485540704403993,
11.8698834704985));
#14949=CARTESIAN_POINT('Ctrl Pts',(-4.08818793877976,0.488689291789136,
11.861178695302));
#14950=CARTESIAN_POINT('Ctrl Pts',(-4.09047268188156,0.491245759629021,
11.8519547869365));
#14951=CARTESIAN_POINT('Ctrl Pts',(-4.1,0.5,11.7890187209227));
#14952=CARTESIAN_POINT('Ctrl Pts',(-4.13477970278813,0.5,11.7464513530047));
#14953=CARTESIAN_POINT('Ctrl Pts',(-4.16929090131684,0.504455968886619,
11.7035428752933));
#14954=CARTESIAN_POINT('Ctrl Pts',(-4.20352761804122,0.513629669484429,
11.6617726299259));
#14955=CARTESIAN_POINT('Ctrl Pts',(-4.10836665945874,0.5,11.7972219040708));
#14956=CARTESIAN_POINT('Ctrl Pts',(-4.14352422788613,0.500728939428738,
11.754930342142));
#14957=CARTESIAN_POINT('Ctrl Pts',(-4.17822160408369,0.506004692387703,
11.7124031482063));
#14958=CARTESIAN_POINT('Ctrl Pts',(-4.21239479773503,0.516005623122533,
11.6711203195198));
#14959=CARTESIAN_POINT('Ctrl Pts',(-4.1167281686604,0.497385130283631,11.8054200375929));
#14960=CARTESIAN_POINT('Ctrl Pts',(-4.1524905396068,0.49863124735402,11.763403178915));
#14961=CARTESIAN_POINT('Ctrl Pts',(-4.18765174637402,0.504533209103448,
11.7212564005378));
#14962=CARTESIAN_POINT('Ctrl Pts',(-4.22210281883105,0.515209463850521,
11.6804590353039));
#14963=CARTESIAN_POINT('Ctrl Pts',(-4.12430006992852,0.492400711949332,
11.8128439913451));
#14964=CARTESIAN_POINT('Ctrl Pts',(-4.16077688798415,0.493922555267979,
11.7710156405394));
#14965=CARTESIAN_POINT('Ctrl Pts',(-4.19655913075278,0.500206823344764,
11.7291447804131));
#14966=CARTESIAN_POINT('Ctrl Pts',(-4.23152093150711,0.511333924981017,
11.6887010425988));
#14967=CARTESIAN_POINT('',(-4.1,0.5,11.7890187209227));
#14968=CARTESIAN_POINT('Origin',(-4.1,0.42,11.7890187209227));
#14969=CARTESIAN_POINT('Ctrl Pts',(-4.1,0.5,11.7890187209227));
#14970=CARTESIAN_POINT('Ctrl Pts',(-4.13477970278813,0.5,11.7464513530047));
#14971=CARTESIAN_POINT('Ctrl Pts',(-4.16929090131684,0.504455968886619,
11.7035428752933));
#14972=CARTESIAN_POINT('Ctrl Pts',(-4.20352761804122,0.513629669484429,
11.6617726299259));
#14973=CARTESIAN_POINT('Ctrl Pts',(-4.13726390506229,0.480634448429844,
11.8255545258696));
#14974=CARTESIAN_POINT('Ctrl Pts',(-4.11846919910142,0.480634448429844,
11.8447237802385));
#14975=CARTESIAN_POINT('Ctrl Pts',(-4.0995468371381,0.480634448429845,11.8638771748766));
#14976=CARTESIAN_POINT('Ctrl Pts',(-4.08038777665855,0.480634448429845,
11.8829301635628));
#14977=CARTESIAN_POINT('Ctrl Pts',(-4.12700765835792,0.492996832959403,
11.8154986761552));
#14978=CARTESIAN_POINT('Ctrl Pts',(-4.10823910349475,0.492996832959403,
11.8346412582769));
#14979=CARTESIAN_POINT('Ctrl Pts',(-4.08935809686133,0.492996832959405,
11.8537525739076));
#14980=CARTESIAN_POINT('Ctrl Pts',(-4.0702594664804,0.492996832959404,11.872745467059));
#14981=CARTESIAN_POINT('Ctrl Pts',(-4.11353190731664,0.500000000000001,
11.8022862280574));
#14982=CARTESIAN_POINT('Ctrl Pts',(-4.09479778199198,0.500000000000001,
11.821393694515));
#14983=CARTESIAN_POINT('Ctrl Pts',(-4.0759708825117,0.500000000000003,11.8404499526433));
#14984=CARTESIAN_POINT('Ctrl Pts',(-4.05695181209536,0.500000000000002,
11.8593637263041));
#14985=CARTESIAN_POINT('Ctrl Pts',(-4.09999999999997,0.500000000000001,
11.7890187209227));
#14986=CARTESIAN_POINT('Ctrl Pts',(-4.08130046851071,0.500000000000001,
11.8080909041452));
#14987=CARTESIAN_POINT('Ctrl Pts',(-4.06252783272246,0.500000000000003,
11.8270919444204));
#14988=CARTESIAN_POINT('Ctrl Pts',(-4.04358870192888,0.500000000000002,
11.8459262210343));
#14989=CARTESIAN_POINT('',(-4.04358870192886,0.5,11.8459262210343));
#14990=CARTESIAN_POINT('Origin',(-4.04358870192886,0.42,11.8459262210343));
#14991=CARTESIAN_POINT('Ctrl Pts',(-4.04358870192888,0.500000000000002,
11.8459262210343));
#14992=CARTESIAN_POINT('Ctrl Pts',(-4.06252783272246,0.500000000000003,
11.8270919444204));
#14993=CARTESIAN_POINT('Ctrl Pts',(-4.08130046851071,0.500000000000001,
11.8080909041452));
#14994=CARTESIAN_POINT('Ctrl Pts',(-4.09999999999997,0.500000000000001,
11.7890187209227));
#14995=CARTESIAN_POINT('Ctrl Pts',(-4.0999999999998,0.42,11.9026515720685));
#14996=CARTESIAN_POINT('Ctrl Pts',(-4.06432399954019,0.42,11.9381300567181));
#14997=CARTESIAN_POINT('Ctrl Pts',(-3.98818997166498,0.42,12.0113742928463));
#14998=CARTESIAN_POINT('Ctrl Pts',(-3.86894020585271,0.42,12.109102240647));
#14999=CARTESIAN_POINT('Ctrl Pts',(-3.73111144412829,0.42,12.1934025947443));
#15000=CARTESIAN_POINT('Ctrl Pts',(-3.52459207479152,0.42,12.2691713922624));
#15001=CARTESIAN_POINT('Ctrl Pts',(-3.26513732430851,0.42,12.297823424652));
#15002=CARTESIAN_POINT('Ctrl Pts',(-2.86516759113243,0.42,12.3018709397382));
#15003=CARTESIAN_POINT('Ctrl Pts',(-2.37243413007993,0.42,12.2928374209075));
#15004=CARTESIAN_POINT('Ctrl Pts',(-1.18525443737258,0.42,12.2925016573196));
#15005=CARTESIAN_POINT('Ctrl Pts',(0.197222451502637,0.42,12.3061814082829));
#15006=CARTESIAN_POINT('Ctrl Pts',(1.58273499720914,0.42,12.2905377746514));
#15007=CARTESIAN_POINT('Ctrl Pts',(2.37158402949751,0.42,12.2934888460097));
#15008=CARTESIAN_POINT('Ctrl Pts',(2.86495583790509,0.42,12.3017734583628));
#15009=CARTESIAN_POINT('Ctrl Pts',(3.26529661019376,0.42,12.2978358829359));
#15010=CARTESIAN_POINT('Ctrl Pts',(3.52422846912908,0.42,12.2692306735397));
#15011=CARTESIAN_POINT('Ctrl Pts',(3.73122727647141,0.42,12.1933706003979));
#15012=CARTESIAN_POINT('Ctrl Pts',(3.86889495391816,0.42,12.1090059816509));
#15013=CARTESIAN_POINT('Ctrl Pts',(3.98631775211335,0.42,12.0130270377017));
#15014=CARTESIAN_POINT('Ctrl Pts',(4.06432399954022,0.42,11.9381300567193));
#15015=CARTESIAN_POINT('Ctrl Pts',(4.09999999999981,0.42,11.9026515720696));
#15016=CARTESIAN_POINT('Ctrl Pts',(-4.0999999999998,0.443935944027351,11.9026515720685));
#15017=CARTESIAN_POINT('Ctrl Pts',(-4.0643220054189,0.443935944027351,11.9381320397991));
#15018=CARTESIAN_POINT('Ctrl Pts',(-3.98819821833631,0.443935944027351,
12.0113730441545));
#15019=CARTESIAN_POINT('Ctrl Pts',(-3.86894133667588,0.443935944027351,
12.1091109056158));
#15020=CARTESIAN_POINT('Ctrl Pts',(-3.73109426468088,0.443935944027351,
12.1934251234395));
#15021=CARTESIAN_POINT('Ctrl Pts',(-3.52453039533999,0.443935944027351,
12.2692079948208));
#15022=CARTESIAN_POINT('Ctrl Pts',(-3.26508191635705,0.443935944027351,
12.2978445388081));
#15023=CARTESIAN_POINT('Ctrl Pts',(-2.86512840714357,0.443935944027351,
12.301883045595));
#15024=CARTESIAN_POINT('Ctrl Pts',(-2.37242384296456,0.443935944027351,
12.2928403209455));
#15025=CARTESIAN_POINT('Ctrl Pts',(-1.18525600106237,0.443935944027351,
12.2925029665493));
#15026=CARTESIAN_POINT('Ctrl Pts',(0.197225231324838,0.44393594402735,12.306179798813));
#15027=CARTESIAN_POINT('Ctrl Pts',(1.58273129397298,0.443935944027351,12.2905396651414));
#15028=CARTESIAN_POINT('Ctrl Pts',(2.3715789007231,0.443935944027351,12.2934900210802));
#15029=CARTESIAN_POINT('Ctrl Pts',(2.8649096643031,0.443935944027351,12.3017877807429));
#15030=CARTESIAN_POINT('Ctrl Pts',(3.26524130832891,0.443935944027351,12.2978569519032));
#15031=CARTESIAN_POINT('Ctrl Pts',(3.52416578331235,0.443935944027351,12.2692675954058));
#15032=CARTESIAN_POINT('Ctrl Pts',(3.73120989460243,0.443935944027351,12.1933931820489));
#15033=CARTESIAN_POINT('Ctrl Pts',(3.86889576959486,0.443935944027351,12.1090147570509));
#15034=CARTESIAN_POINT('Ctrl Pts',(3.98632566897136,0.443935944027351,12.0130260375901));
#15035=CARTESIAN_POINT('Ctrl Pts',(4.06432200541893,0.443935944027351,11.9381320398003));
#15036=CARTESIAN_POINT('Ctrl Pts',(4.09999999999981,0.443935944027351,11.9026515720696));
#15037=CARTESIAN_POINT('Ctrl Pts',(-4.08582416466455,0.48536014866598,11.8883968170266));
#15038=CARTESIAN_POINT('Ctrl Pts',(-4.05030544143939,0.48536014866598,11.9237188951879));
#15039=CARTESIAN_POINT('Ctrl Pts',(-3.97469565176084,0.48536014866598,11.9964466583217));
#15040=CARTESIAN_POINT('Ctrl Pts',(-3.85709194674926,0.48536014866598,12.0927846652945));
#15041=CARTESIAN_POINT('Ctrl Pts',(-3.72224972003245,0.48536014866598,12.1751942765285));
#15042=CARTESIAN_POINT('Ctrl Pts',(-3.52063687145968,0.48536014866598,12.2492378201496));
#15043=CARTESIAN_POINT('Ctrl Pts',(-3.26439665787152,0.48536014866598,12.2777279953723));
#15044=CARTESIAN_POINT('Ctrl Pts',(-2.86552312724983,0.48536014866598,12.2817557317464));
#15045=CARTESIAN_POINT('Ctrl Pts',(-2.37263653108989,0.48536014866598,12.2727373685992));
#15046=CARTESIAN_POINT('Ctrl Pts',(-1.18492906129251,0.485360148665981,
12.2723917905604));
#15047=CARTESIAN_POINT('Ctrl Pts',(0.19708118789358,0.48536014866598,12.2860843598974));
#15048=CARTESIAN_POINT('Ctrl Pts',(1.58260427556699,0.485360148665981,12.2704294766691));
#15049=CARTESIAN_POINT('Ctrl Pts',(2.37177678789268,0.48536014866598,12.2733912458457));
#15050=CARTESIAN_POINT('Ctrl Pts',(2.86532273287249,0.48536014866598,12.2816545608874));
#15051=CARTESIAN_POINT('Ctrl Pts',(3.26455255367795,0.48536014866598,12.2777416788692));
#15052=CARTESIAN_POINT('Ctrl Pts',(3.5202829538042,0.48536014866598,12.2492936061086));
#15053=CARTESIAN_POINT('Ctrl Pts',(3.72236308599005,0.48536014866598,12.1751634108215));
#15054=CARTESIAN_POINT('Ctrl Pts',(3.85705298820777,0.48536014866598,12.092684991886));
#15055=CARTESIAN_POINT('Ctrl Pts',(3.97284435283825,0.48536014866598,11.9980807271348));
#15056=CARTESIAN_POINT('Ctrl Pts',(4.05030544143941,0.48536014866598,11.9237188951891));
#15057=CARTESIAN_POINT('Ctrl Pts',(4.08582416466454,0.48536014866598,11.8883968170278));
#15058=CARTESIAN_POINT('Ctrl Pts',(-4.05624736761451,0.5,11.8586553600401));
#15059=CARTESIAN_POINT('Ctrl Pts',(-4.02105560774434,0.5,11.893652285039));
#15060=CARTESIAN_POINT('Ctrl Pts',(-3.94654567923738,0.5,11.9653005485802));
#15061=CARTESIAN_POINT('Ctrl Pts',(-3.83237213080353,0.5,12.0587444343159));
#15062=CARTESIAN_POINT('Ctrl Pts',(-3.7037502134039,0.5,12.1372173836306));
#15063=CARTESIAN_POINT('Ctrl Pts',(-3.51234803324907,0.5,12.2076696701355));
#15064=CARTESIAN_POINT('Ctrl Pts',(-3.26281842755994,0.5,12.2358129498859));
#15065=CARTESIAN_POINT('Ctrl Pts',(-2.86624166923353,0.5,12.2397940727743));
#15066=CARTESIAN_POINT('Ctrl Pts',(-2.37305271959604,0.5,12.230801866854));
#15067=CARTESIAN_POINT('Ctrl Pts',(-1.18425111706809,0.500000000000001,
12.2304348675178));
#15068=CARTESIAN_POINT('Ctrl Pts',(0.196788102082843,0.499999999999999,
12.24415244907));
#15069=CARTESIAN_POINT('Ctrl Pts',(1.58232933686155,0.5,12.2284761717562));
#15070=CARTESIAN_POINT('Ctrl Pts',(2.37217591946072,0.499999999999999,12.2314598364887));
#15071=CARTESIAN_POINT('Ctrl Pts',(2.86606082566913,0.5,12.2396865196674));
#15072=CARTESIAN_POINT('Ctrl Pts',(3.26296731319181,0.5,12.2358291628754));
#15073=CARTESIAN_POINT('Ctrl Pts',(3.51201373156969,0.5,12.2077183528994));
#15074=CARTESIAN_POINT('Ctrl Pts',(3.70385831329287,0.5,12.1371889041741));
#15075=CARTESIAN_POINT('Ctrl Pts',(3.83234611589616,0.5,12.0586377025416));
#15076=CARTESIAN_POINT('Ctrl Pts',(3.94473783385368,0.5,11.9668957987984));
#15077=CARTESIAN_POINT('Ctrl Pts',(4.02105560774433,0.5,11.8936522850402));
#15078=CARTESIAN_POINT('Ctrl Pts',(4.05624736761446,0.5,11.8586553600413));
#15079=CARTESIAN_POINT('Ctrl Pts',(-4.04358870192886,0.5,11.8459262210343));
#15080=CARTESIAN_POINT('Ctrl Pts',(-4.00853667496434,0.5,11.8807841867417));
#15081=CARTESIAN_POINT('Ctrl Pts',(-3.9344985330766,0.5,11.9519700993884));
#15082=CARTESIAN_POINT('Ctrl Pts',(-3.82179233596298,0.5,12.0441763410897));
#15083=CARTESIAN_POINT('Ctrl Pts',(-3.69583078434751,0.5,12.120965852524));
#15084=CARTESIAN_POINT('Ctrl Pts',(-3.50879412174487,0.5,12.1898825536479));
#15085=CARTESIAN_POINT('Ctrl Pts',(-3.26213725530659,0.5,12.2178757710291));
#15086=CARTESIAN_POINT('Ctrl Pts',(-2.86654516889356,0.5,12.2218360168654));
#15087=CARTESIAN_POINT('Ctrl Pts',(-2.37322978704452,0.5,12.2128540589361));
#15088=CARTESIAN_POINT('Ctrl Pts',(-1.18396112248055,0.500000000000001,
12.2124777277647));
#15089=CARTESIAN_POINT('Ctrl Pts',(0.196662949368364,0.499999999999999,
12.2262057140885));
#15090=CARTESIAN_POINT('Ctrl Pts',(1.58221128398681,0.5,12.2105206403396));
#15091=CARTESIAN_POINT('Ctrl Pts',(2.37234621736262,0.499999999999999,12.2135136026149));
#15092=CARTESIAN_POINT('Ctrl Pts',(2.86637197383024,0.5,12.2217259602429));
#15093=CARTESIAN_POINT('Ctrl Pts',(3.26228315154647,0.5,12.2178930619748));
#15094=CARTESIAN_POINT('Ctrl Pts',(3.50846811203046,0.5,12.1899282291445));
#15095=CARTESIAN_POINT('Ctrl Pts',(3.69593660956959,0.5,12.1209383998147));
#15096=CARTESIAN_POINT('Ctrl Pts',(3.82177182841876,0.5,12.0440665997448));
#15097=CARTESIAN_POINT('Ctrl Pts',(3.93270925157646,0.5,11.9535487610897));
#15098=CARTESIAN_POINT('Ctrl Pts',(4.00853667496432,0.5,11.8807841867429));
#15099=CARTESIAN_POINT('Ctrl Pts',(4.0435887019288,0.5,11.8459262210355));
#15100=CARTESIAN_POINT('',(4.09999999999981,0.42,11.9026515720696));
#15101=CARTESIAN_POINT('Ctrl Pts',(-4.08957475120668,0.42,11.9129846529869));
#15102=CARTESIAN_POINT('Ctrl Pts',(-4.07070912639531,0.42,11.9316191145701));
#15103=CARTESIAN_POINT('Ctrl Pts',(-4.0512337618078,0.42,11.9504965620406));
#15104=CARTESIAN_POINT('Ctrl Pts',(-4.03136941462863,0.42,11.9691382395571));
#15105=CARTESIAN_POINT('Ctrl Pts',(-4.01968819006244,0.42,11.9801004735231));
#15106=CARTESIAN_POINT('Ctrl Pts',(-4.00787168701817,0.42,11.9909814506739));
#15107=CARTESIAN_POINT('Ctrl Pts',(-3.9959601173972,0.42,12.0016910697278));
#15108=CARTESIAN_POINT('Ctrl Pts',(-3.98877368957404,0.42,12.0081523428256));
#15109=CARTESIAN_POINT('Ctrl Pts',(-3.98155552980581,0.42,12.0145488528393));
#15110=CARTESIAN_POINT('Ctrl Pts',(-3.97430247432981,0.42,12.0208725332347));
#15111=CARTESIAN_POINT('Ctrl Pts',(-3.95549323097764,0.42,12.0372716416975));
#15112=CARTESIAN_POINT('Ctrl Pts',(-3.93643357392197,0.42,12.0531996537834));
#15113=CARTESIAN_POINT('Ctrl Pts',(-3.91688135136191,0.42,12.0686460330885));
#15114=CARTESIAN_POINT('Ctrl Pts',(-3.89958719643529,0.42,12.0823085247022));
#15115=CARTESIAN_POINT('Ctrl Pts',(-3.88190823253498,0.42,12.0955935663832));
#15116=CARTESIAN_POINT('Ctrl Pts',(-3.86365572107541,0.42,12.1084664329205));
#15117=CARTESIAN_POINT('Ctrl Pts',(-3.84554580736162,0.42,12.121238730188));
#15118=CARTESIAN_POINT('Ctrl Pts',(-3.82687067374783,0.42,12.1335981171097));
#15119=CARTESIAN_POINT('Ctrl Pts',(-3.80766293258994,0.42,12.1453574730567));
#15120=CARTESIAN_POINT('Ctrl Pts',(-3.78860525190984,0.42,12.1570249590355));
#15121=CARTESIAN_POINT('Ctrl Pts',(-3.76902255736466,0.42,12.1681009219439));
#15122=CARTESIAN_POINT('Ctrl Pts',(-3.74894872534242,0.42,12.1784597126869));
#15123=CARTESIAN_POINT('Ctrl Pts',(-3.73602631200023,0.42,12.1851281243563));
#15124=CARTESIAN_POINT('Ctrl Pts',(-3.72289678284864,0.42,12.1915021804535));
#15125=CARTESIAN_POINT('Ctrl Pts',(-3.70958667619023,0.42,12.1975557390669));
#15126=CARTESIAN_POINT('Ctrl Pts',(-3.69192772874079,0.42,12.2055871903678));
#15127=CARTESIAN_POINT('Ctrl Pts',(-3.67395508821995,0.42,12.213050119862));
#15128=CARTESIAN_POINT('Ctrl Pts',(-3.65577503211398,0.42,12.2199120405514));
#15129=CARTESIAN_POINT('Ctrl Pts',(-3.63730907646068,0.42,12.2268818718));
#15130=CARTESIAN_POINT('Ctrl Pts',(-3.61862858092384,0.42,12.2332320858495));
#15131=CARTESIAN_POINT('Ctrl Pts',(-3.59987390808581,0.42,12.2389739060236));
#15132=CARTESIAN_POINT('Ctrl Pts',(-3.58812827122212,0.42,12.2425698810258));
#15133=CARTESIAN_POINT('Ctrl Pts',(-3.57635645365837,0.42,12.2459275182189));
#15134=CARTESIAN_POINT('Ctrl Pts',(-3.56459228573084,0.42,12.2490589093387));
#15135=CARTESIAN_POINT('Ctrl Pts',(-3.53640474847592,0.42,12.2565618797478));
#15136=CARTESIAN_POINT('Ctrl Pts',(-3.50822366783652,0.42,12.2627808667959));
#15137=CARTESIAN_POINT('Ctrl Pts',(-3.48006243281124,0.42,12.2680130438463));
#15138=CARTESIAN_POINT('Ctrl Pts',(-3.45179977817908,0.42,12.2732640640098));
#15139=CARTESIAN_POINT('Ctrl Pts',(-3.42355783651323,0.42,12.2775216531967));
#15140=CARTESIAN_POINT('Ctrl Pts',(-3.39537788085669,0.42,12.2810411396377));
#15141=CARTESIAN_POINT('Ctrl Pts',(-3.36659368263903,0.42,12.2846360919002));
#15142=CARTESIAN_POINT('Ctrl Pts',(-3.33787477852993,0.42,12.2874610919638));
#15143=CARTESIAN_POINT('Ctrl Pts',(-3.30928381995259,0.42,12.2897363835961));
#15144=CARTESIAN_POINT('Ctrl Pts',(-3.29376488816646,0.42,12.2909713927525));
#15145=CARTESIAN_POINT('Ctrl Pts',(-3.27828562790243,0.42,12.2920434331052));
#15146=CARTESIAN_POINT('Ctrl Pts',(-3.26285194183848,0.42,12.292981865386));
#15147=CARTESIAN_POINT('Ctrl Pts',(-3.23369857325195,0.42,12.2947545114061));
#15148=CARTESIAN_POINT('Ctrl Pts',(-3.20468141212112,0.42,12.2960551913495));
#15149=CARTESIAN_POINT('Ctrl Pts',(-3.17579045328073,0.42,12.2970396330972));
#15150=CARTESIAN_POINT('Ctrl Pts',(-3.14550795106456,0.42,12.2980714908341));
#15151=CARTESIAN_POINT('Ctrl Pts',(-3.11536462644417,0.42,12.2987553967142));
#15152=CARTESIAN_POINT('Ctrl Pts',(-3.08532794916976,0.42,12.2992169145794));
#15153=CARTESIAN_POINT('Ctrl Pts',(-3.05377633819841,0.42,12.2997017096187));
#15154=CARTESIAN_POINT('Ctrl Pts',(-3.0223429235208,0.42,12.2999404094041));
#15155=CARTESIAN_POINT('Ctrl Pts',(-2.99095908120567,0.42,12.300030121024));
#15156=CARTESIAN_POINT('Ctrl Pts',(-2.97279349404179,0.42,12.3000820478797));
#15157=CARTESIAN_POINT('Ctrl Pts',(-2.95464182185859,0.42,12.3000832384085));
#15158=CARTESIAN_POINT('Ctrl Pts',(-2.93649043054004,0.42,12.3000470713686));
#15159=CARTESIAN_POINT('Ctrl Pts',(-2.89676042107724,0.42,12.2999679084653));
#15160=CARTESIAN_POINT('Ctrl Pts',(-2.85705476098733,0.42,12.2997128386374));
#15161=CARTESIAN_POINT('Ctrl Pts',(-2.81741363626107,0.42,12.2993798909943));
#15162=CARTESIAN_POINT('Ctrl Pts',(-2.77585567983252,0.42,12.2990308437929));
#15163=CARTESIAN_POINT('Ctrl Pts',(-2.73436928668848,0.42,12.2985951218158));
#15164=CARTESIAN_POINT('Ctrl Pts',(-2.69296287950309,0.42,12.2981386342706));
#15165=CARTESIAN_POINT('Ctrl Pts',(-2.65015799313489,0.42,12.2976667291035));
#15166=CARTESIAN_POINT('Ctrl Pts',(-2.60743892093361,0.42,12.2971716744601));
#15167=CARTESIAN_POINT('Ctrl Pts',(-2.56476785938501,0.42,12.2966935956038));
#15168=CARTESIAN_POINT('Ctrl Pts',(-2.52908709297847,0.42,12.29629383475));
#15169=CARTESIAN_POINT('Ctrl Pts',(-2.49343899198747,0.42,12.2959052051901));
#15170=CARTESIAN_POINT('Ctrl Pts',(-2.45777598101278,0.42,12.29554055751));
#15171=CARTESIAN_POINT('Ctrl Pts',(-2.4327936161251,0.42,12.2952851174574));
#15172=CARTESIAN_POINT('Ctrl Pts',(-2.40780344620683,0.42,12.2950412596816));
#15173=CARTESIAN_POINT('Ctrl Pts',(-2.38278265214531,0.42,12.2948116115015));
#15174=CARTESIAN_POINT('Ctrl Pts',(-2.36409688161798,0.42,12.2946401080239));
#15175=CARTESIAN_POINT('Ctrl Pts',(-2.34539571618718,0.42,12.294476523425));
#15176=CARTESIAN_POINT('Ctrl Pts',(-2.3266909260608,0.42,12.2943217432458));
#15177=CARTESIAN_POINT('Ctrl Pts',(-2.27024903989047,0.42,12.2938546925492));
#15178=CARTESIAN_POINT('Ctrl Pts',(-2.21375528545711,0.42,12.2934689635508));
#15179=CARTESIAN_POINT('Ctrl Pts',(-2.15726656535151,0.42,12.2931722059907));
#15180=CARTESIAN_POINT('Ctrl Pts',(-2.09932295136259,0.42,12.2928678052983));
#15181=CARTESIAN_POINT('Ctrl Pts',(-2.04138464776779,0.42,12.2926564220354));
#15182=CARTESIAN_POINT('Ctrl Pts',(-1.98346034243504,0.42,12.2925319928656));
#15183=CARTESIAN_POINT('Ctrl Pts',(-1.92373696814234,0.42,12.2924036990547));
#15184=CARTESIAN_POINT('Ctrl Pts',(-1.86402835174857,0.42,12.2923674602502));
#15185=CARTESIAN_POINT('Ctrl Pts',(-1.80428946616947,0.42,12.2924092102655));
#15186=CARTESIAN_POINT('Ctrl Pts',(-1.78362811703507,0.42,12.2924236499664));
#15187=CARTESIAN_POINT('Ctrl Pts',(-1.76296338243997,0.42,12.2924473754325));
#15188=CARTESIAN_POINT('Ctrl Pts',(-1.74227825988445,0.42,12.2924797416047));
#15189=CARTESIAN_POINT('Ctrl Pts',(-1.66551379267926,0.42,12.2925998555636));
#15190=CARTESIAN_POINT('Ctrl Pts',(-1.58853637524402,0.42,12.2928393894616));
#15191=CARTESIAN_POINT('Ctrl Pts',(-1.51149675923115,0.42,12.2931600654634));
#15192=CARTESIAN_POINT('Ctrl Pts',(-1.43226893428785,0.42,12.2934898498452));
#15193=CARTESIAN_POINT('Ctrl Pts',(-1.35297520958703,0.42,12.2939050013854));
#15194=CARTESIAN_POINT('Ctrl Pts',(-1.27372326985414,0.42,12.2943620060925));
#15195=CARTESIAN_POINT('Ctrl Pts',(-1.19121670263452,0.42,12.2948377785431));
#15196=CARTESIAN_POINT('Ctrl Pts',(-1.10875518516202,0.42,12.2953586061595));
#15197=CARTESIAN_POINT('Ctrl Pts',(-1.02640265123843,0.42,12.2958793155528));
#15198=CARTESIAN_POINT('Ctrl Pts',(-0.939286032192044,0.42,12.2964301479279));
#15199=CARTESIAN_POINT('Ctrl Pts',(-0.852290996877637,0.42,12.2969806094654));
#15200=CARTESIAN_POINT('Ctrl Pts',(-0.765434646151399,0.42,12.2974858650896));
#15201=CARTESIAN_POINT('Ctrl Pts',(-0.671380899427911,0.42,12.2980329889799));
#15202=CARTESIAN_POINT('Ctrl Pts',(-0.57748916422919,0.42,12.2985268001515));
#15203=CARTESIAN_POINT('Ctrl Pts',(-0.483721777843278,0.42,12.2989246112183));
#15204=CARTESIAN_POINT('Ctrl Pts',(-0.371719028569128,0.42,12.2993997863818));
#15205=CARTESIAN_POINT('Ctrl Pts',(-0.259892687853164,0.42,12.2997368001716));
#15206=CARTESIAN_POINT('Ctrl Pts',(-0.148108023827894,0.42,12.2998948321153));
#15207=CARTESIAN_POINT('Ctrl Pts',(-0.0348382015673389,0.42,12.3000549636533));
#15208=CARTESIAN_POINT('Ctrl Pts',(0.0783927177796026,0.42,12.3000304822599));
#15209=CARTESIAN_POINT('Ctrl Pts',(0.191748815331185,0.42,12.299824260992));
#15210=CARTESIAN_POINT('Ctrl Pts',(0.273957475225655,0.42,12.2996747042021));
#15211=CARTESIAN_POINT('Ctrl Pts',(0.356232687434953,0.42,12.2994307737856));
#15212=CARTESIAN_POINT('Ctrl Pts',(0.438626822026294,0.42,12.2991085248334));
#15213=CARTESIAN_POINT('Ctrl Pts',(0.486761625529418,0.42,12.2989202664085));
#15214=CARTESIAN_POINT('Ctrl Pts',(0.534936768026288,0.42,12.2987054934661));
#15215=CARTESIAN_POINT('Ctrl Pts',(0.583159437202681,0.42,12.2984690821935));
#15216=CARTESIAN_POINT('Ctrl Pts',(0.600704406570152,0.42,12.2983830681132));
#15217=CARTESIAN_POINT('Ctrl Pts',(0.61825202790425,0.42,12.2982942177471));
#15218=CARTESIAN_POINT('Ctrl Pts',(0.635793398928577,0.42,12.2982028570652));
#15219=CARTESIAN_POINT('Ctrl Pts',(0.722624179925258,0.42,12.2977506165105));
#15220=CARTESIAN_POINT('Ctrl Pts',(0.809376157106363,0.42,12.2972357585868));
#15221=CARTESIAN_POINT('Ctrl Pts',(0.896142685250265,0.42,12.2966978388299));
#15222=CARTESIAN_POINT('Ctrl Pts',(0.976708017257756,0.42,12.2961983641508));
#15223=CARTESIAN_POINT('Ctrl Pts',(1.05728638072386,0.42,12.2956791514925));
#15224=CARTESIAN_POINT('Ctrl Pts',(1.13791082663924,0.42,12.2951788015391));
#15225=CARTESIAN_POINT('Ctrl Pts',(1.21452814789454,0.42,12.294703319535));
#15226=CARTESIAN_POINT('Ctrl Pts',(1.29118742965583,0.42,12.2942450181282));
#15227=CARTESIAN_POINT('Ctrl Pts',(1.36787207531147,0.42,12.2938415740963));
#15228=CARTESIAN_POINT('Ctrl Pts',(1.44182337776109,0.42,12.2934525104009));
#15229=CARTESIAN_POINT('Ctrl Pts',(1.51579851999178,0.42,12.2931146870792));
#15230=CARTESIAN_POINT('Ctrl Pts',(1.5897353553651,0.42,12.2928636232826));
#15231=CARTESIAN_POINT('Ctrl Pts',(1.64315891931009,0.42,12.2926822154264));
#15232=CARTESIAN_POINT('Ctrl Pts',(1.69656152233123,0.42,12.2925461826626));
#15233=CARTESIAN_POINT('Ctrl Pts',(1.74990250989962,0.42,12.2924682031349));
#15234=CARTESIAN_POINT('Ctrl Pts',(1.81164714531486,0.42,12.2923779382612));
#15235=CARTESIAN_POINT('Ctrl Pts',(1.87329665865665,0.42,12.2923655874348));
#15236=CARTESIAN_POINT('Ctrl Pts',(1.93494398932289,0.42,12.2924476940399));
#15237=CARTESIAN_POINT('Ctrl Pts',(1.99177230648263,0.42,12.2925233823161));
#15238=CARTESIAN_POINT('Ctrl Pts',(2.04859905035996,0.42,12.2926795846011));
#15239=CARTESIAN_POINT('Ctrl Pts',(2.10544947311221,0.42,12.2929245095271));
#15240=CARTESIAN_POINT('Ctrl Pts',(2.16086336245647,0.42,12.2931632455309));
#15241=CARTESIAN_POINT('Ctrl Pts',(2.2162998172383,0.42,12.2934867203752));
#15242=CARTESIAN_POINT('Ctrl Pts',(2.2717345377493,0.42,12.2938928339529));
#15243=CARTESIAN_POINT('Ctrl Pts',(2.30424765863584,0.42,12.2941310243817));
#15244=CARTESIAN_POINT('Ctrl Pts',(2.33675926922426,0.42,12.2943974408816));
#15245=CARTESIAN_POINT('Ctrl Pts',(2.36925649852847,0.42,12.2946888798043));
#15246=CARTESIAN_POINT('Ctrl Pts',(2.38798692621633,0.42,12.2948568564528));
#15247=CARTESIAN_POINT('Ctrl Pts',(2.40670347471599,0.42,12.2950330172923));
#15248=CARTESIAN_POINT('Ctrl Pts',(2.42541331068238,0.42,12.2952163892074));
#15249=CARTESIAN_POINT('Ctrl Pts',(2.46864196476304,0.42,12.295640065882));
#15250=CARTESIAN_POINT('Ctrl Pts',(2.51184253377794,0.42,12.2961032804126));
#15251=CARTESIAN_POINT('Ctrl Pts',(2.55510163816728,0.42,12.2965855577766));
#15252=CARTESIAN_POINT('Ctrl Pts',(2.59710888202152,0.42,12.2970538786797));
#15253=CARTESIAN_POINT('Ctrl Pts',(2.63917124418029,0.42,12.2975407387835));
#15254=CARTESIAN_POINT('Ctrl Pts',(2.68132348844875,0.42,12.298009707522));
#15255=CARTESIAN_POINT('Ctrl Pts',(2.72181559106942,0.42,12.2984602061993));
#15256=CARTESIAN_POINT('Ctrl Pts',(2.76239031938167,0.42,12.2988949370747));
#15257=CARTESIAN_POINT('Ctrl Pts',(2.80303973715188,0.42,12.2992556829302));
#15258=CARTESIAN_POINT('Ctrl Pts',(2.83631806432058,0.42,12.2995510135712));
#15259=CARTESIAN_POINT('Ctrl Pts',(2.86964564495769,0.42,12.2997966701148));
#15260=CARTESIAN_POINT('Ctrl Pts',(2.90300032749941,0.42,12.2999403096602));
#15261=CARTESIAN_POINT('Ctrl Pts',(2.9253128012298,0.42,12.3000363967262));
#15262=CARTESIAN_POINT('Ctrl Pts',(2.94763579581574,0.42,12.3000864441799));
#15263=CARTESIAN_POINT('Ctrl Pts',(2.96996315170153,0.42,12.3000682690189));
#15264=CARTESIAN_POINT('Ctrl Pts',(3.001246560905,0.42,12.3000428033523));
#15265=CARTESIAN_POINT('Ctrl Pts',(3.03255914305104,0.42,12.2998853345777));
#15266=CARTESIAN_POINT('Ctrl Pts',(3.06397042497329,0.42,12.299508487312));
#15267=CARTESIAN_POINT('Ctrl Pts',(3.09387571006892,0.42,12.2991497077835));
#15268=CARTESIAN_POINT('Ctrl Pts',(3.12387002346923,0.42,12.2985926943181));
#15269=CARTESIAN_POINT('Ctrl Pts',(3.15398744202724,0.42,12.2977244393391));
#15270=CARTESIAN_POINT('Ctrl Pts',(3.18152646583026,0.42,12.2969305168957));
#15271=CARTESIAN_POINT('Ctrl Pts',(3.20916793051934,0.42,12.295876467876));
#15272=CARTESIAN_POINT('Ctrl Pts',(3.23692222273258,0.42,12.2944393742418));
#15273=CARTESIAN_POINT('Ctrl Pts',(3.25616037421766,0.42,12.2934432391279));
#15274=CARTESIAN_POINT('Ctrl Pts',(3.275450562525,0.42,12.2922625424322));
#15275=CARTESIAN_POINT('Ctrl Pts',(3.29480672148807,0.42,12.2908428966008));
#15276=CARTESIAN_POINT('Ctrl Pts',(3.32306225045922,0.42,12.2887705410268));
#15277=CARTESIAN_POINT('Ctrl Pts',(3.35144553838964,0.42,12.2861918016504));
#15278=CARTESIAN_POINT('Ctrl Pts',(3.37990572257727,0.42,12.2829011177135));
#15279=CARTESIAN_POINT('Ctrl Pts',(3.40779276483902,0.42,12.2796767028112));
#15280=CARTESIAN_POINT('Ctrl Pts',(3.43575306489468,0.42,12.2757687321118));
#15281=CARTESIAN_POINT('Ctrl Pts',(3.46375142663797,0.42,12.2709352312518));
#15282=CARTESIAN_POINT('Ctrl Pts',(3.49164628247108,0.42,12.2661195991483));
#15283=CARTESIAN_POINT('Ctrl Pts',(3.5195782146669,0.42,12.2603849831845));
#15284=CARTESIAN_POINT('Ctrl Pts',(3.54753465345975,0.42,12.253445044257));
#15285=CARTESIAN_POINT('Ctrl Pts',(3.55922703608369,0.42,12.2505425135761));
#15286=CARTESIAN_POINT('Ctrl Pts',(3.57092593140847,0.42,12.2474280556932));
#15287=CARTESIAN_POINT('Ctrl Pts',(3.582625824136,0.42,12.2440804130704));
#15288=CARTESIAN_POINT('Ctrl Pts',(3.60127037025197,0.42,12.2387457250768));
#15289=CARTESIAN_POINT('Ctrl Pts',(3.61989878758966,0.42,12.232820362843));
#15290=CARTESIAN_POINT('Ctrl Pts',(3.63835640205551,0.42,12.2262827655873));
#15291=CARTESIAN_POINT('Ctrl Pts',(3.65652907738884,0.42,12.2198460923861));
#15292=CARTESIAN_POINT('Ctrl Pts',(3.67453667498046,0.42,12.2128154357668));
#15293=CARTESIAN_POINT('Ctrl Pts',(3.69226143752051,0.42,12.2052109768377));
#15294=CARTESIAN_POINT('Ctrl Pts',(3.70807253769151,0.42,12.1984275369128));
#15295=CARTESIAN_POINT('Ctrl Pts',(3.72365839535628,0.42,12.1911883500437));
#15296=CARTESIAN_POINT('Ctrl Pts',(3.73895335801981,0.42,12.1835382315404));
#15297=CARTESIAN_POINT('Ctrl Pts',(3.75809368978208,0.42,12.1739647654655));
#15298=CARTESIAN_POINT('Ctrl Pts',(3.77678640737143,0.42,12.1637435281572));
#15299=CARTESIAN_POINT('Ctrl Pts',(3.79498734855382,0.42,12.1529840694506));
#15300=CARTESIAN_POINT('Ctrl Pts',(3.80954442722186,0.42,12.1443786745292));
#15301=CARTESIAN_POINT('Ctrl Pts',(3.82378730102014,0.42,12.135430261965));
#15302=CARTESIAN_POINT('Ctrl Pts',(3.83769546581467,0.42,12.1262188936489));
#15303=CARTESIAN_POINT('Ctrl Pts',(3.84723128386294,0.42,12.1199033276821));
#15304=CARTESIAN_POINT('Ctrl Pts',(3.85660972029853,0.42,12.1134646514204));
#15305=CARTESIAN_POINT('Ctrl Pts',(3.86582411962837,0.42,12.106933278707));
#15306=CARTESIAN_POINT('Ctrl Pts',(3.8833908188634,0.42,12.0944816086696));
#15307=CARTESIAN_POINT('Ctrl Pts',(3.90037718862227,0.42,12.0816882444054));
#15308=CARTESIAN_POINT('Ctrl Pts',(3.91703215924884,0.42,12.0685268765388));
#15309=CARTESIAN_POINT('Ctrl Pts',(3.93298261941915,0.42,12.0559222386412));
#15310=CARTESIAN_POINT('Ctrl Pts',(3.94862830275337,0.42,12.0429793468167));
#15311=CARTESIAN_POINT('Ctrl Pts',(3.96417057138444,0.42,12.0296382333238));
#15312=CARTESIAN_POINT('Ctrl Pts',(3.97157392199353,0.42,12.0232833733579));
#15313=CARTESIAN_POINT('Ctrl Pts',(3.97895364133667,0.42,12.0168376559896));
#15314=CARTESIAN_POINT('Ctrl Pts',(3.98633070224374,0.42,12.0102922388325));
#15315=CARTESIAN_POINT('Ctrl Pts',(4.00248995147145,0.42,11.9959546823893));
#15316=CARTESIAN_POINT('Ctrl Pts',(4.01861703151618,0.42,11.9811508058126));
#15317=CARTESIAN_POINT('Ctrl Pts',(4.0345005913335,0.42,11.9661948419058));
#15318=CARTESIAN_POINT('Ctrl Pts',(4.05281961135389,0.42,11.948945648061));
#15319=CARTESIAN_POINT('Ctrl Pts',(4.07081647195516,0.42,11.9314955882412));
#15320=CARTESIAN_POINT('Ctrl Pts',(4.08814786889807,0.42,11.9143933611413));
#15321=CARTESIAN_POINT('Ctrl Pts',(4.09213542393225,0.42,11.9104585328067));
#15322=CARTESIAN_POINT('Ctrl Pts',(4.09608761671172,0.42,11.9065422949265));
#15323=CARTESIAN_POINT('Ctrl Pts',(4.09999999999981,0.42,11.9026515720696));
#15324=CARTESIAN_POINT('',(4.0435887019288,0.5,11.8459262210355));
#15325=CARTESIAN_POINT('Origin',(4.0435887019288,0.42,11.8459262210355));
#15326=CARTESIAN_POINT('Ctrl Pts',(4.0435887019288,0.5,11.8459262210355));
#15327=CARTESIAN_POINT('Ctrl Pts',(4.00853667496432,0.5,11.8807841867429));
#15328=CARTESIAN_POINT('Ctrl Pts',(3.93270925157646,0.5,11.9535487610897));
#15329=CARTESIAN_POINT('Ctrl Pts',(3.82177182841876,0.5,12.0440665997448));
#15330=CARTESIAN_POINT('Ctrl Pts',(3.69593660956959,0.5,12.1209383998147));
#15331=CARTESIAN_POINT('Ctrl Pts',(3.50846811203046,0.5,12.1899282291445));
#15332=CARTESIAN_POINT('Ctrl Pts',(3.26228315154647,0.5,12.2178930619748));
#15333=CARTESIAN_POINT('Ctrl Pts',(2.86637197383024,0.5,12.2217259602429));
#15334=CARTESIAN_POINT('Ctrl Pts',(2.37234621736262,0.499999999999999,12.2135136026149));
#15335=CARTESIAN_POINT('Ctrl Pts',(1.58221128398681,0.5,12.2105206403396));
#15336=CARTESIAN_POINT('Ctrl Pts',(0.196662949368364,0.499999999999999,
12.2262057140885));
#15337=CARTESIAN_POINT('Ctrl Pts',(-1.18396112248055,0.500000000000001,
12.2124777277647));
#15338=CARTESIAN_POINT('Ctrl Pts',(-2.37322978704452,0.5,12.2128540589361));
#15339=CARTESIAN_POINT('Ctrl Pts',(-2.86654516889356,0.5,12.2218360168654));
#15340=CARTESIAN_POINT('Ctrl Pts',(-3.26213725530659,0.5,12.2178757710291));
#15341=CARTESIAN_POINT('Ctrl Pts',(-3.50879412174487,0.5,12.1898825536479));
#15342=CARTESIAN_POINT('Ctrl Pts',(-3.69583078434751,0.5,12.120965852524));
#15343=CARTESIAN_POINT('Ctrl Pts',(-3.82179233596298,0.5,12.0441763410897));
#15344=CARTESIAN_POINT('Ctrl Pts',(-3.9344985330766,0.5,11.9519700993884));
#15345=CARTESIAN_POINT('Ctrl Pts',(-4.00853667496434,0.5,11.8807841867417));
#15346=CARTESIAN_POINT('Ctrl Pts',(-4.04358870192886,0.5,11.8459262210343));
#15347=CARTESIAN_POINT('Ctrl Pts',(-4.0999999999998,0.,11.9026515720685));
#15348=CARTESIAN_POINT('Ctrl Pts',(-4.0999999999998,0.6,11.9026515720685));
#15349=CARTESIAN_POINT('Ctrl Pts',(-4.09081961446015,0.,11.9117811315272));
#15350=CARTESIAN_POINT('Ctrl Pts',(-4.09081961446015,0.6,11.9117811315272));
#15351=CARTESIAN_POINT('Ctrl Pts',(-4.05565687163378,0.,11.9465013108369));
#15352=CARTESIAN_POINT('Ctrl Pts',(-4.05565687163378,0.6,11.9465013108369));
#15353=CARTESIAN_POINT('Ctrl Pts',(-3.99482565231276,0.,12.0046763352293));
#15354=CARTESIAN_POINT('Ctrl Pts',(-3.99482565231276,0.6,12.0046763352293));
#15355=CARTESIAN_POINT('Ctrl Pts',(-3.9081172594404,0.,12.0806818325556));
#15356=CARTESIAN_POINT('Ctrl Pts',(-3.9081172594404,0.6,12.0806818325556));
#15357=CARTESIAN_POINT('Ctrl Pts',(-3.79241297762166,0.,12.1626050652586));
#15358=CARTESIAN_POINT('Ctrl Pts',(-3.79241297762166,0.6,12.1626050652586));
#15359=CARTESIAN_POINT('Ctrl Pts',(-3.64927048315908,0.,12.2301117722809));
#15360=CARTESIAN_POINT('Ctrl Pts',(-3.64927048315908,0.6,12.2301117722809));
#15361=CARTESIAN_POINT('Ctrl Pts',(-3.48993681214334,0.,12.2723364229645));
#15362=CARTESIAN_POINT('Ctrl Pts',(-3.48993681214334,0.6,12.2723364229645));
#15363=CARTESIAN_POINT('Ctrl Pts',(-3.30884480305534,0.,12.2938762651139));
#15364=CARTESIAN_POINT('Ctrl Pts',(-3.30884480305534,0.6,12.2938762651139));
#15365=CARTESIAN_POINT('Ctrl Pts',(-3.10127560868576,0.,12.3010487961981));
#15366=CARTESIAN_POINT('Ctrl Pts',(-3.10127560868576,0.6,12.3010487961981));
#15367=CARTESIAN_POINT('Ctrl Pts',(-2.86376302967345,0.,12.300400839059));
#15368=CARTESIAN_POINT('Ctrl Pts',(-2.86376302967345,0.6,12.300400839059));
#15369=CARTESIAN_POINT('Ctrl Pts',(-2.59461297443094,0.,12.2969132923574));
#15370=CARTESIAN_POINT('Ctrl Pts',(-2.59461297443094,0.6,12.2969132923574));
#15371=CARTESIAN_POINT('Ctrl Pts',(-2.29394197380209,0.,12.2935845551224));
#15372=CARTESIAN_POINT('Ctrl Pts',(-2.29394197380209,0.6,12.2935845551224));
#15373=CARTESIAN_POINT('Ctrl Pts',(-1.96338745719135,0.,12.2919684497906));
#15374=CARTESIAN_POINT('Ctrl Pts',(-1.96338745719135,0.6,12.2919684497906));
#15375=CARTESIAN_POINT('Ctrl Pts',(-1.60591558979456,0.,12.2924280531798));
#15376=CARTESIAN_POINT('Ctrl Pts',(-1.60591558979456,0.6,12.2924280531798));
#15377=CARTESIAN_POINT('Ctrl Pts',(-1.22558901314075,0.,12.2945066442122));
#15378=CARTESIAN_POINT('Ctrl Pts',(-1.22558901314075,0.6,12.2945066442122));
#15379=CARTESIAN_POINT('Ctrl Pts',(-0.827351903312651,0.,12.2972483292773));
#15380=CARTESIAN_POINT('Ctrl Pts',(-0.827351903312651,0.6,12.2972483292773));
#15381=CARTESIAN_POINT('Ctrl Pts',(-0.498916532526571,0.,12.299081889758));
#15382=CARTESIAN_POINT('Ctrl Pts',(-0.498916532526571,0.6,12.299081889758));
#15383=CARTESIAN_POINT('Ctrl Pts',(-0.249771440080693,0.,12.2998330708668));
#15384=CARTESIAN_POINT('Ctrl Pts',(-0.249771440080693,0.6,12.2998330708668));
#15385=CARTESIAN_POINT('Ctrl Pts',(-0.0832571466935557,0.,12.2999999999989));
#15386=CARTESIAN_POINT('Ctrl Pts',(-0.0832571466935557,0.6,12.2999999999989));
#15387=CARTESIAN_POINT('Ctrl Pts',(0.,0.,12.3));
#15388=CARTESIAN_POINT('Ctrl Pts',(0.,0.6,12.3));
#15389=CARTESIAN_POINT('Ctrl Pts',(0.0832571466935396,0.,12.3000000000011));
#15390=CARTESIAN_POINT('Ctrl Pts',(0.0832571466935396,0.6,12.3000000000011));
#15391=CARTESIAN_POINT('Ctrl Pts',(0.24977144008061,0.,12.2998330708736));
#15392=CARTESIAN_POINT('Ctrl Pts',(0.24977144008061,0.6,12.2998330708736));
#15393=CARTESIAN_POINT('Ctrl Pts',(0.498916532526534,0.,12.2990818897713));
#15394=CARTESIAN_POINT('Ctrl Pts',(0.498916532526534,0.6,12.2990818897713));
#15395=CARTESIAN_POINT('Ctrl Pts',(0.827351903312438,0.,12.2972483292974));
#15396=CARTESIAN_POINT('Ctrl Pts',(0.827351903312438,0.6,12.2972483292974));
#15397=CARTESIAN_POINT('Ctrl Pts',(1.22558901314046,0.,12.2945066442369));
#15398=CARTESIAN_POINT('Ctrl Pts',(1.22558901314046,0.6,12.2945066442369));
#15399=CARTESIAN_POINT('Ctrl Pts',(1.60591558979418,0.,12.2924280532047));
#15400=CARTESIAN_POINT('Ctrl Pts',(1.60591558979418,0.6,12.2924280532047));
#15401=CARTESIAN_POINT('Ctrl Pts',(1.96338745719096,0.,12.291968449812));
#15402=CARTESIAN_POINT('Ctrl Pts',(1.96338745719096,0.6,12.291968449812));
#15403=CARTESIAN_POINT('Ctrl Pts',(2.29394197380175,0.,12.2935845551378));
#15404=CARTESIAN_POINT('Ctrl Pts',(2.29394197380175,0.6,12.2935845551378));
#15405=CARTESIAN_POINT('Ctrl Pts',(2.59461297443069,0.,12.2969132923658));
#15406=CARTESIAN_POINT('Ctrl Pts',(2.59461297443069,0.6,12.2969132923658));
#15407=CARTESIAN_POINT('Ctrl Pts',(2.86376302967335,0.,12.3004008390612));
#15408=CARTESIAN_POINT('Ctrl Pts',(2.86376302967335,0.6,12.3004008390612));
#15409=CARTESIAN_POINT('Ctrl Pts',(3.10127560868576,0.,12.3010487961961));
#15410=CARTESIAN_POINT('Ctrl Pts',(3.10127560868576,0.6,12.3010487961961));
#15411=CARTESIAN_POINT('Ctrl Pts',(3.30884480305537,0.,12.2938762651102));
#15412=CARTESIAN_POINT('Ctrl Pts',(3.30884480305537,0.6,12.2938762651102));
#15413=CARTESIAN_POINT('Ctrl Pts',(3.48993681214337,0.,12.2723364229612));
#15414=CARTESIAN_POINT('Ctrl Pts',(3.48993681214337,0.6,12.2723364229612));
#15415=CARTESIAN_POINT('Ctrl Pts',(3.64927048315907,0.,12.2301117722792));
#15416=CARTESIAN_POINT('Ctrl Pts',(3.64927048315907,0.6,12.2301117722792));
#15417=CARTESIAN_POINT('Ctrl Pts',(3.79241297762162,0.,12.1626050652587));
#15418=CARTESIAN_POINT('Ctrl Pts',(3.79241297762162,0.6,12.1626050652587));
#15419=CARTESIAN_POINT('Ctrl Pts',(3.90811725944037,0.,12.0806818325567));
#15420=CARTESIAN_POINT('Ctrl Pts',(3.90811725944037,0.6,12.0806818325567));
#15421=CARTESIAN_POINT('Ctrl Pts',(3.99482565231275,0.,12.0046763352306));
#15422=CARTESIAN_POINT('Ctrl Pts',(3.99482565231275,0.6,12.0046763352306));
#15423=CARTESIAN_POINT('Ctrl Pts',(4.05565687163378,0.,11.9465013108382));
#15424=CARTESIAN_POINT('Ctrl Pts',(4.05565687163378,0.6,11.9465013108382));
#15425=CARTESIAN_POINT('Ctrl Pts',(4.09081961446015,0.,11.9117811315284));
#15426=CARTESIAN_POINT('Ctrl Pts',(4.09081961446015,0.6,11.9117811315284));
#15427=CARTESIAN_POINT('Ctrl Pts',(4.09999999999981,0.,11.9026515720696));
#15428=CARTESIAN_POINT('Ctrl Pts',(4.09999999999981,0.6,11.9026515720696));
#15429=CARTESIAN_POINT('',(-4.09999999999981,0.08,11.9026515720685));
#15430=CARTESIAN_POINT('',(-4.1,0.,11.9026515720683));
#15431=CARTESIAN_POINT('',(4.0999999999999,0.08,11.9026515720696));
#15432=CARTESIAN_POINT('Ctrl Pts',(4.09999999999981,0.08,11.9026515720696));
#15433=CARTESIAN_POINT('Ctrl Pts',(4.08085111799688,0.08,11.9216944386311));
#15434=CARTESIAN_POINT('Ctrl Pts',(4.06101542096552,0.08,11.9410853975879));
#15435=CARTESIAN_POINT('Ctrl Pts',(4.04073585097501,0.08,11.9603045561526));
#15436=CARTESIAN_POINT('Ctrl Pts',(4.02436441134365,0.08,11.97581993909));
#15437=CARTESIAN_POINT('Ctrl Pts',(4.00770239235104,0.08,11.9912224049274));
#15438=CARTESIAN_POINT('Ctrl Pts',(3.99086144408298,0.08,12.0062594906044));
#15439=CARTESIAN_POINT('Ctrl Pts',(3.98153193750382,0.08,12.0145896978778));
#15440=CARTESIAN_POINT('Ctrl Pts',(3.97215358351719,0.08,12.0228031793437));
#15441=CARTESIAN_POINT('Ctrl Pts',(3.96270172391276,0.08,12.0308975945789));
#15442=CARTESIAN_POINT('Ctrl Pts',(3.94584705089436,0.08,12.045331655999));
#15443=CARTESIAN_POINT('Ctrl Pts',(3.92875556290024,0.08,12.0593923164246));
#15444=CARTESIAN_POINT('Ctrl Pts',(3.91125351666559,0.08,12.0730677817931));
#15445=CARTESIAN_POINT('Ctrl Pts',(3.89832363377578,0.08,12.0831707242324));
#15446=CARTESIAN_POINT('Ctrl Pts',(3.8851694742044,0.08,12.0930629305754));
#15447=CARTESIAN_POINT('Ctrl Pts',(3.87171397149225,0.08,12.102730041241));
#15448=CARTESIAN_POINT('Ctrl Pts',(3.8614190416025,0.08,12.1101264372485));
#15449=CARTESIAN_POINT('Ctrl Pts',(3.85094099847984,0.08,12.1173949809926));
#15450=CARTESIAN_POINT('Ctrl Pts',(3.84027953928806,0.08,12.12450190652));
#15451=CARTESIAN_POINT('Ctrl Pts',(3.82175706889362,0.08,12.136848979778));
#15452=CARTESIAN_POINT('Ctrl Pts',(3.80268700852572,0.08,12.1487003513866));
#15453=CARTESIAN_POINT('Ctrl Pts',(3.78310122932964,0.08,12.1598936311512));
#15454=CARTESIAN_POINT('Ctrl Pts',(3.76586254638967,0.08,12.1697455445721));
#15455=CARTESIAN_POINT('Ctrl Pts',(3.74822395968075,0.08,12.1790882008887));
#15456=CARTESIAN_POINT('Ctrl Pts',(3.73021120715776,0.08,12.1878507821834));
#15457=CARTESIAN_POINT('Ctrl Pts',(3.71288220522445,0.08,12.1962807424575));
#15458=CARTESIAN_POINT('Ctrl Pts',(3.69520648253534,0.08,12.2041725145781));
#15459=CARTESIAN_POINT('Ctrl Pts',(3.6772807651628,0.08,12.2114752670303));
#15460=CARTESIAN_POINT('Ctrl Pts',(3.6591356399706,0.08,12.2188674039663));
#15461=CARTESIAN_POINT('Ctrl Pts',(3.64073365439416,0.08,12.2256564236659));
#15462=CARTESIAN_POINT('Ctrl Pts',(3.62219995454964,0.08,12.2318367403961));
#15463=CARTESIAN_POINT('Ctrl Pts',(3.6080919145163,0.08,12.2365412600861));
#15464=CARTESIAN_POINT('Ctrl Pts',(3.59390804694076,0.08,12.2408941383227));
#15465=CARTESIAN_POINT('Ctrl Pts',(3.57971589417065,0.08,12.2449082304703));
#15466=CARTESIAN_POINT('Ctrl Pts',(3.56437379192782,0.08,12.2492475730026));
#15467=CARTESIAN_POINT('Ctrl Pts',(3.54903220918601,0.08,12.2531896473898));
#15468=CARTESIAN_POINT('Ctrl Pts',(3.5336945114111,0.08,12.2567838613074));
#15469=CARTESIAN_POINT('Ctrl Pts',(3.50554417223935,0.08,12.2633805710823));
#15470=CARTESIAN_POINT('Ctrl Pts',(3.47740156491547,0.08,12.2688092691411));
#15471=CARTESIAN_POINT('Ctrl Pts',(3.44929127767962,0.08,12.2733508469725));
#15472=CARTESIAN_POINT('Ctrl Pts',(3.4208806380215,0.08,12.2779409505942));
#15473=CARTESIAN_POINT('Ctrl Pts',(3.39250369100482,0.08,12.2816252157076));
#15474=CARTESIAN_POINT('Ctrl Pts',(3.364210072182,0.08,12.2846455979633));
#15475=CARTESIAN_POINT('Ctrl Pts',(3.34067447290198,0.08,12.2871580551675));
#15476=CARTESIAN_POINT('Ctrl Pts',(3.31719712358888,0.08,12.2892101937693));
#15477=CARTESIAN_POINT('Ctrl Pts',(3.29381437654729,0.08,12.2909154727553));
#15478=CARTESIAN_POINT('Ctrl Pts',(3.26990846383811,0.08,12.2926589056595));
#15479=CARTESIAN_POINT('Ctrl Pts',(3.24611026789158,0.08,12.2940396163213));
#15480=CARTESIAN_POINT('Ctrl Pts',(3.22239636521847,0.08,12.2951574602113));
#15481=CARTESIAN_POINT('Ctrl Pts',(3.19272700000078,0.08,12.2965560372015));
#15482=CARTESIAN_POINT('Ctrl Pts',(3.16319729337309,0.08,12.2975435340936));
#15483=CARTESIAN_POINT('Ctrl Pts',(3.13378818621321,0.08,12.2982614632568));
#15484=CARTESIAN_POINT('Ctrl Pts',(3.10291902762736,0.08,12.2990150348996));
#15485=CARTESIAN_POINT('Ctrl Pts',(3.07218325518306,0.08,12.2994710273203));
#15486=CARTESIAN_POINT('Ctrl Pts',(3.04153322298808,0.08,12.2997413666759));
#15487=CARTESIAN_POINT('Ctrl Pts',(3.01414756926293,0.08,12.2999829135667));
#15488=CARTESIAN_POINT('Ctrl Pts',(2.98683142537097,0.08,12.3000750815676));
#15489=CARTESIAN_POINT('Ctrl Pts',(2.95952635057301,0.08,12.3000718531387));
#15490=CARTESIAN_POINT('Ctrl Pts',(2.92022752887084,0.08,12.3000672066233));
#15491=CARTESIAN_POINT('Ctrl Pts',(2.88094163407949,0.08,12.2998660100441));
#15492=CARTESIAN_POINT('Ctrl Pts',(2.84171310121476,0.08,12.299573016108));
#15493=CARTESIAN_POINT('Ctrl Pts',(2.80046664143214,0.08,12.2992649504803));
#15494=CARTESIAN_POINT('Ctrl Pts',(2.75928426917026,0.08,12.2988543578822));
#15495=CARTESIAN_POINT('Ctrl Pts',(2.71818210888147,0.08,12.2984132059186));
#15496=CARTESIAN_POINT('Ctrl Pts',(2.67559761222298,0.08,12.2979561439494));
#15497=CARTESIAN_POINT('Ctrl Pts',(2.63309961275455,0.08,12.2974652765352));
#15498=CARTESIAN_POINT('Ctrl Pts',(2.59066040545446,0.08,12.2969852179935));
#15499=CARTESIAN_POINT('Ctrl Pts',(2.54700739090149,0.08,12.296491429258));
#15500=CARTESIAN_POINT('Ctrl Pts',(2.50341670354419,0.08,12.2960083404301));
#15501=CARTESIAN_POINT('Ctrl Pts',(2.45980678945122,0.08,12.2955613475654));
#15502=CARTESIAN_POINT('Ctrl Pts',(2.43495747913403,0.08,12.2953066471231));
#15503=CARTESIAN_POINT('Ctrl Pts',(2.41010097941813,0.08,12.2950633182646));
#15504=CARTESIAN_POINT('Ctrl Pts',(2.38521498311308,0.08,12.2948339814447));
#15505=CARTESIAN_POINT('Ctrl Pts',(2.36524312905612,0.08,12.2946499308871));
#15506=CARTESIAN_POINT('Ctrl Pts',(2.3452529798216,0.08,12.2944748786647));
#15507=CARTESIAN_POINT('Ctrl Pts',(2.32525887175618,0.08,12.2943099103763));
#15508=CARTESIAN_POINT('Ctrl Pts',(2.26880377106821,0.08,12.2938441080859));
#15509=CARTESIAN_POINT('Ctrl Pts',(2.21229745148629,0.08,12.2934598053646));
#15510=CARTESIAN_POINT('Ctrl Pts',(2.15579643324432,0.08,12.2931645025908));
#15511=CARTESIAN_POINT('Ctrl Pts',(2.09783882688532,0.08,12.292861586954));
#15512=CARTESIAN_POINT('Ctrl Pts',(2.03988681065597,0.08,12.2926517251859));
#15513=CARTESIAN_POINT('Ctrl Pts',(1.98194864244373,0.08,12.2925287651092));
#15514=CARTESIAN_POINT('Ctrl Pts',(1.92220737766913,0.0800000000000001,
12.292401978386));
#15515=CARTESIAN_POINT('Ctrl Pts',(1.86248071190454,0.08,12.2923672037462));
#15516=CARTESIAN_POINT('Ctrl Pts',(1.80272313765481,0.08,12.2924103227315));
#15517=CARTESIAN_POINT('Ctrl Pts',(1.78236504214316,0.08,12.2924250124245));
#15518=CARTESIAN_POINT('Ctrl Pts',(1.76200320414501,0.08,12.2924487012689));
#15519=CARTESIAN_POINT('Ctrl Pts',(1.74162156320725,0.08,12.292480772058));
#15520=CARTESIAN_POINT('Ctrl Pts',(1.66485073951616,0.08,12.2926015719925));
#15521=CARTESIAN_POINT('Ctrl Pts',(1.5878674439253,0.08,12.2928417064317));
#15522=CARTESIAN_POINT('Ctrl Pts',(1.5108223052039,0.08,12.2931628749459));
#15523=CARTESIAN_POINT('Ctrl Pts',(1.43158637455503,0.08,12.2934931759427));
#15524=CARTESIAN_POINT('Ctrl Pts',(1.35228491570348,0.08,12.2939087355891));
#15525=CARTESIAN_POINT('Ctrl Pts',(1.27302549034632,0.0800000000000001,
12.2943660309377));
#15526=CARTESIAN_POINT('Ctrl Pts',(1.1905078550462,0.0800000000000001,12.2948421248613));
#15527=CARTESIAN_POINT('Ctrl Pts',(1.10803554212318,0.08,12.2953631505531));
#15528=CARTESIAN_POINT('Ctrl Pts',(1.02567235785951,0.08,12.2958839331962));
#15529=CARTESIAN_POINT('Ctrl Pts',(0.938539807628001,0.08,12.2964348725534));
#15530=CARTESIAN_POINT('Ctrl Pts',(0.851529016120771,0.0800000000000001,
12.2969853013965));
#15531=CARTESIAN_POINT('Ctrl Pts',(0.764656942700882,0.0800000000000001,
12.2974903879526));
#15532=CARTESIAN_POINT('Ctrl Pts',(0.670578247057742,0.0800000000000001,
12.2980373748324));
#15533=CARTESIAN_POINT('Ctrl Pts',(0.576661628618322,0.0800000000000001,
12.2985308796243));
#15534=CARTESIAN_POINT('Ctrl Pts',(0.482869249226626,0.0800000000000001,
12.2989282255145));
#15535=CARTESIAN_POINT('Ctrl Pts',(0.370835051600932,0.0800000000000001,
12.2994028517929));
#15536=CARTESIAN_POINT('Ctrl Pts',(0.258977105568546,0.08,12.2997390836903));
#15537=CARTESIAN_POINT('Ctrl Pts',(0.147160428731306,0.08,12.2998961675423));
#15538=CARTESIAN_POINT('Ctrl Pts',(0.0339191259990135,0.08,12.3000552527569));
#15539=CARTESIAN_POINT('Ctrl Pts',(-0.0792837384867833,0.08,12.3000297581724));
#15540=CARTESIAN_POINT('Ctrl Pts',(-0.192612106107584,0.08,12.2998226870296));
#15541=CARTESIAN_POINT('Ctrl Pts',(-0.274803209508849,0.08,12.2996725092226));
#15542=CARTESIAN_POINT('Ctrl Pts',(-0.357061036136113,0.08,12.2994280361329));
#15543=CARTESIAN_POINT('Ctrl Pts',(-0.439437867128799,0.08,12.2991053502863));
#15544=CARTESIAN_POINT('Ctrl Pts',(-0.48787066530124,0.08,12.2989156297265));
#15545=CARTESIAN_POINT('Ctrl Pts',(-0.536344351747438,0.08,12.2986990890481));
#15546=CARTESIAN_POINT('Ctrl Pts',(-0.584866221452301,0.08,12.2984607057927));
#15547=CARTESIAN_POINT('Ctrl Pts',(-0.601617610893425,0.08,12.2983784078357));
#15548=CARTESIAN_POINT('Ctrl Pts',(-0.618370748229175,0.08,12.2982935358771));
#15549=CARTESIAN_POINT('Ctrl Pts',(-0.635118395921561,0.08,12.2982063714116));
#15550=CARTESIAN_POINT('Ctrl Pts',(-0.7219687678754,0.08,12.2977543517373));
#15551=CARTESIAN_POINT('Ctrl Pts',(-0.808739990504138,0.08,12.2972395965865));
#15552=CARTESIAN_POINT('Ctrl Pts',(-0.895525604899384,0.08,12.2967016641001));
#15553=CARTESIAN_POINT('Ctrl Pts',(-0.976102388614265,0.08,12.296202216468));
#15554=CARTESIAN_POINT('Ctrl Pts',(-1.05669206509419,0.08,12.2956829345119));
#15555=CARTESIAN_POINT('Ctrl Pts',(-1.13732782725138,0.08,12.2951824199131));
#15556=CARTESIAN_POINT('Ctrl Pts',(-1.21395246397961,0.08,12.2947068027889));
#15557=CARTESIAN_POINT('Ctrl Pts',(-1.29061906065972,0.08,12.2942482785114));
#15558=CARTESIAN_POINT('Ctrl Pts',(-1.36731114548385,0.08,12.2938445261533));
#15559=CARTESIAN_POINT('Ctrl Pts',(-1.44126731795944,0.08,12.2934551772512));
#15560=CARTESIAN_POINT('Ctrl Pts',(-1.51524744450851,0.08,12.2931169858094));
#15561=CARTESIAN_POINT('Ctrl Pts',(-1.58918949676173,0.08,12.292865478377));
#15562=CARTESIAN_POINT('Ctrl Pts',(-1.64262457071585,0.08,12.2926837236402));
#15563=CARTESIAN_POINT('Ctrl Pts',(-1.69603879964548,0.08,12.2925473178858));
#15564=CARTESIAN_POINT('Ctrl Pts',(-1.74939155466375,0.08,12.2924689518492));
#15565=CARTESIAN_POINT('Ctrl Pts',(-1.81138702877719,0.08,12.2923778911421));
#15566=CARTESIAN_POINT('Ctrl Pts',(-1.87328650735159,0.08,12.292365329224));
#15567=CARTESIAN_POINT('Ctrl Pts',(-1.93518382952162,0.08,12.2924480139311));
#15568=CARTESIAN_POINT('Ctrl Pts',(-1.99201075404425,0.08,12.2925239254156));
#15569=CARTESIAN_POINT('Ctrl Pts',(-2.04883617969711,0.08,12.2926803633538));
#15570=CARTESIAN_POINT('Ctrl Pts',(-2.10568527146238,0.08,12.2929255258877));
#15571=CARTESIAN_POINT('Ctrl Pts',(-2.1610981357588,0.08,12.2931644946697));
#15572=CARTESIAN_POINT('Ctrl Pts',(-2.21653355338608,0.08,12.2934882052722));
#15573=CARTESIAN_POINT('Ctrl Pts',(-2.27196714524091,0.08,12.2938945384932));
#15574=CARTESIAN_POINT('Ctrl Pts',(-2.30462425317035,0.08,12.2941339180356));
#15575=CARTESIAN_POINT('Ctrl Pts',(-2.33727981008809,0.08,12.2944017716056));
#15576=CARTESIAN_POINT('Ctrl Pts',(-2.3699207434827,0.08,12.2946948402871));
#15577=CARTESIAN_POINT('Ctrl Pts',(-2.38860422091697,0.08,12.2948625910689));
#15578=CARTESIAN_POINT('Ctrl Pts',(-2.40727353322535,0.08,12.2950384715363));
#15579=CARTESIAN_POINT('Ctrl Pts',(-2.42593646929677,0.08,12.2952215184717));
#15580=CARTESIAN_POINT('Ctrl Pts',(-2.46915994082182,0.08,12.2956454562686));
#15581=CARTESIAN_POINT('Ctrl Pts',(-2.5123557613935,0.08,12.2961088688924));
#15582=CARTESIAN_POINT('Ctrl Pts',(-2.5556103407381,0.08,12.2965912298652));
#15583=CARTESIAN_POINT('Ctrl Pts',(-2.59761221637401,0.08,12.2970596210944));
#15584=CARTESIAN_POINT('Ctrl Pts',(-2.63966941763936,0.08,12.2975464435437));
#15585=CARTESIAN_POINT('Ctrl Pts',(-2.6818165243447,0.08,12.2980151918792));
#15586=CARTESIAN_POINT('Ctrl Pts',(-2.72230118964439,0.08,12.2984654510063));
#15587=CARTESIAN_POINT('Ctrl Pts',(-2.76286849091756,0.08,12.2988997761342));
#15588=CARTESIAN_POINT('Ctrl Pts',(-2.80351035458597,0.08,12.2992598559852));
#15589=CARTESIAN_POINT('Ctrl Pts',(-2.83665379540435,0.08,12.2995535011125));
#15590=CARTESIAN_POINT('Ctrl Pts',(-2.86984601586543,0.08,12.2997976670906));
#15591=CARTESIAN_POINT('Ctrl Pts',(-2.90306509578608,0.08,12.2999405884475));
#15592=CARTESIAN_POINT('Ctrl Pts',(-2.92537741132963,0.08,12.3000365846769));
#15593=CARTESIAN_POINT('Ctrl Pts',(-2.9477002227499,0.08,12.3000865234911));
#15594=CARTESIAN_POINT('Ctrl Pts',(-2.97002743072866,0.08,12.3000682165033));
#15595=CARTESIAN_POINT('Ctrl Pts',(-3.00130987000378,0.08,12.3000425667564));
#15596=CARTESIAN_POINT('Ctrl Pts',(-3.0326215472723,0.08,12.2998848748288));
#15597=CARTESIAN_POINT('Ctrl Pts',(-3.06403195826998,0.08,12.2995077488028));
#15598=CARTESIAN_POINT('Ctrl Pts',(-3.09393641998059,0.08,12.2991487038095));
#15599=CARTESIAN_POINT('Ctrl Pts',(-3.12392994078988,0.08,12.2985913743274));
#15600=CARTESIAN_POINT('Ctrl Pts',(-3.1540465763897,0.08,12.2977227341565));
#15601=CARTESIAN_POINT('Ctrl Pts',(-3.1815930910073,0.08,12.2969282227947));
#15602=CARTESIAN_POINT('Ctrl Pts',(-3.20924211628561,0.08,12.2958733738442));
#15603=CARTESIAN_POINT('Ctrl Pts',(-3.23700403466603,0.08,12.2944351369897));
#15604=CARTESIAN_POINT('Ctrl Pts',(-3.2562020509982,0.08,12.2934405625427));
#15605=CARTESIAN_POINT('Ctrl Pts',(-3.27545188943979,0.08,12.292262127272));
#15606=CARTESIAN_POINT('Ctrl Pts',(-3.2947674345378,0.08,12.2908457777182));
#15607=CARTESIAN_POINT('Ctrl Pts',(-3.32302318748729,0.08,12.2887738702013));
#15608=CARTESIAN_POINT('Ctrl Pts',(-3.35140672998653,0.08,12.286195650168));
#15609=CARTESIAN_POINT('Ctrl Pts',(-3.37986719282862,0.08,12.2829055722533));
#15610=CARTESIAN_POINT('Ctrl Pts',(-3.40775432368432,0.08,12.2796817724915));
#15611=CARTESIAN_POINT('Ctrl Pts',(-3.43571473452292,0.08,12.2757745092888));
#15612=CARTESIAN_POINT('Ctrl Pts',(-3.46371322028709,0.08,12.2709418264406));
#15613=CARTESIAN_POINT('Ctrl Pts',(-3.49160795780378,0.08,12.2661270510743));
#15614=CARTESIAN_POINT('Ctrl Pts',(-3.51953978424926,0.08,12.2603934176664));
#15615=CARTESIAN_POINT('Ctrl Pts',(-3.54749611690544,0.08,12.2534546098573));
#15616=CARTESIAN_POINT('Ctrl Pts',(-3.55919101099375,0.08,12.2505519178831));
#15617=CARTESIAN_POINT('Ctrl Pts',(-3.57089240832327,0.08,12.2474372356666));
#15618=CARTESIAN_POINT('Ctrl Pts',(-3.58259483305825,0.08,12.2440892798788));
#15619=CARTESIAN_POINT('Ctrl Pts',(-3.60123965610208,0.08,12.2387551679632));
#15620=CARTESIAN_POINT('Ctrl Pts',(-3.61986844142307,0.08,12.2328303885715));
#15621=CARTESIAN_POINT('Ctrl Pts',(-3.63832649186014,0.08,12.2262933590496));
#15622=CARTESIAN_POINT('Ctrl Pts',(-3.65649948761467,0.08,12.2198572833571));
#15623=CARTESIAN_POINT('Ctrl Pts',(-3.67450747348183,0.08,12.2128272165978));
#15624=CARTESIAN_POINT('Ctrl Pts',(-3.69223267685152,0.08,12.2052233154293));
#15625=CARTESIAN_POINT('Ctrl Pts',(-3.7080454670573,0.08,12.1984398167344));
#15626=CARTESIAN_POINT('Ctrl Pts',(-3.72363302436823,0.08,12.1912004677199));
#15627=CARTESIAN_POINT('Ctrl Pts',(-3.73892965687719,0.08,12.1835500857559));
#15628=CARTESIAN_POINT('Ctrl Pts',(-3.75806999941515,0.08,12.1739773297097));
#15629=CARTESIAN_POINT('Ctrl Pts',(-3.77676276852181,0.08,12.1637567909941));
#15630=CARTESIAN_POINT('Ctrl Pts',(-3.79496379833088,0.08,12.1529979906693));
#15631=CARTESIAN_POINT('Ctrl Pts',(-3.80952218159534,0.08,12.144392393061));
#15632=CARTESIAN_POINT('Ctrl Pts',(-3.82376633054058,0.08,12.1354436934871));
#15633=CARTESIAN_POINT('Ctrl Pts',(-3.83767573576978,0.08,12.1262319605201));
#15634=CARTESIAN_POINT('Ctrl Pts',(-3.84721444931906,0.08,12.1199147901871));
#15635=CARTESIAN_POINT('Ctrl Pts',(-3.85659570047497,0.08,12.1134744181737));
#15636=CARTESIAN_POINT('Ctrl Pts',(-3.86581281892743,0.08,12.1069412887918));
#15637=CARTESIAN_POINT('Ctrl Pts',(-3.88337947259145,0.08,12.0944899764009));
#15638=CARTESIAN_POINT('Ctrl Pts',(-3.9003657611309,0.08,12.0816969810865));
#15639=CARTESIAN_POINT('Ctrl Pts',(-3.91702061319308,0.08,12.0685360005523));
#15640=CARTESIAN_POINT('Ctrl Pts',(-3.9329721656094,0.08,12.0559307807606));
#15641=CARTESIAN_POINT('Ctrl Pts',(-3.94861886098581,0.08,12.0429872732068));
#15642=CARTESIAN_POINT('Ctrl Pts',(-3.96416210392647,0.08,12.0296455015386));
#15643=CARTESIAN_POINT('Ctrl Pts',(-3.971565740585,0.08,12.0232904808914));
#15644=CARTESIAN_POINT('Ctrl Pts',(-3.97894573577746,0.08,12.0168445998276));
#15645=CARTESIAN_POINT('Ctrl Pts',(-3.98632307325471,0.08,12.0102990077394));
#15646=CARTESIAN_POINT('Ctrl Pts',(-4.00248188436664,0.08,11.9959619943526));
#15647=CARTESIAN_POINT('Ctrl Pts',(-4.01860857072346,0.08,11.9811586329138));
#15648=CARTESIAN_POINT('Ctrl Pts',(-4.03449178471336,0.08,11.9662031341815));
#15649=CARTESIAN_POINT('Ctrl Pts',(-4.05281046348137,0.08,11.9489544226005));
#15650=CARTESIAN_POINT('Ctrl Pts',(-4.07080704435507,0.08,11.9315047769153));
#15651=CARTESIAN_POINT('Ctrl Pts',(-4.08813823052043,0.08,11.9144028720395));
#15652=CARTESIAN_POINT('Ctrl Pts',(-4.09212905724568,0.08,11.9104648415792));
#15653=CARTESIAN_POINT('Ctrl Pts',(-4.0960844664969,0.08,11.9065454276994));
#15654=CARTESIAN_POINT('Ctrl Pts',(-4.0999999999998,0.08,11.9026515720685));
#15655=CARTESIAN_POINT('',(4.1,0.,11.9026515720695));
#15656=CARTESIAN_POINT('Ctrl Pts',(-4.1,-3.,3.08701851589457));
#15657=CARTESIAN_POINT('Ctrl Pts',(-4.1,4.2,3.08701851589457));
#15658=CARTESIAN_POINT('Ctrl Pts',(-4.10321177777735,-3.,3.11273802327628));
#15659=CARTESIAN_POINT('Ctrl Pts',(-4.10321177777735,4.2,3.11273802327628));
#15660=CARTESIAN_POINT('Ctrl Pts',(-4.1120982065295,-3.,3.18044435652227));
#15661=CARTESIAN_POINT('Ctrl Pts',(-4.1120982065295,4.2,3.18044435652227));
#15662=CARTESIAN_POINT('Ctrl Pts',(-4.12837174871823,-3.,3.28931577678178));
#15663=CARTESIAN_POINT('Ctrl Pts',(-4.12837174871823,4.2,3.28931577678178));
#15664=CARTESIAN_POINT('Ctrl Pts',(-4.1558308051397,-3.,3.43759550531425));
#15665=CARTESIAN_POINT('Ctrl Pts',(-4.1558308051397,4.2,3.43759550531425));
#15666=CARTESIAN_POINT('Ctrl Pts',(-4.20184334854115,-3.,3.62185203209171));
#15667=CARTESIAN_POINT('Ctrl Pts',(-4.20184334854115,4.2,3.62185203209171));
#15668=CARTESIAN_POINT('Ctrl Pts',(-4.26765207024395,-3.,3.81399668859083));
#15669=CARTESIAN_POINT('Ctrl Pts',(-4.26765207024395,4.2,3.81399668859083));
#15670=CARTESIAN_POINT('Ctrl Pts',(-4.35148411330718,-3.,3.99681013615577));
#15671=CARTESIAN_POINT('Ctrl Pts',(-4.35148411330718,4.2,3.99681013615577));
#15672=CARTESIAN_POINT('Ctrl Pts',(-4.45474519640294,-3.,4.16885849319142));
#15673=CARTESIAN_POINT('Ctrl Pts',(-4.45474519640294,4.2,4.16885849319142));
#15674=CARTESIAN_POINT('Ctrl Pts',(-4.57800047823775,-3.,4.32911151507774));
#15675=CARTESIAN_POINT('Ctrl Pts',(-4.57800047823775,4.2,4.32911151507774));
#15676=CARTESIAN_POINT('Ctrl Pts',(-4.7208720035032,-3.,4.47714872481861));
#15677=CARTESIAN_POINT('Ctrl Pts',(-4.7208720035032,4.2,4.47714872481861));
#15678=CARTESIAN_POINT('Ctrl Pts',(-4.88190185104852,-3.,4.61340315498244));
#15679=CARTESIAN_POINT('Ctrl Pts',(-4.88190185104852,4.2,4.61340315498244));
#15680=CARTESIAN_POINT('Ctrl Pts',(-5.05850630701885,-3.,4.73929437247796));
#15681=CARTESIAN_POINT('Ctrl Pts',(-5.05850630701885,4.2,4.73929437247796));
#15682=CARTESIAN_POINT('Ctrl Pts',(-5.24741086000019,-3.,4.8567611153285));
#15683=CARTESIAN_POINT('Ctrl Pts',(-5.24741086000019,4.2,4.8567611153285));
#15684=CARTESIAN_POINT('Ctrl Pts',(-5.44501860313342,-3.,4.96787993373728));
#15685=CARTESIAN_POINT('Ctrl Pts',(-5.44501860313342,4.2,4.96787993373728));
#15686=CARTESIAN_POINT('Ctrl Pts',(-5.64781737380319,-3.,5.07442896098937));
#15687=CARTESIAN_POINT('Ctrl Pts',(-5.64781737380319,4.2,5.07442896098937));
#15688=CARTESIAN_POINT('Ctrl Pts',(-5.85274048349242,-3.,5.17752467829109));
#15689=CARTESIAN_POINT('Ctrl Pts',(-5.85274048349242,4.2,5.17752467829109));
#15690=CARTESIAN_POINT('Ctrl Pts',(-6.05762450882858,-3.,5.27709955371564));
#15691=CARTESIAN_POINT('Ctrl Pts',(-6.05762450882858,4.2,5.27709955371564));
#15692=CARTESIAN_POINT('Ctrl Pts',(-6.26112587698772,-3.,5.37226655127787));
#15693=CARTESIAN_POINT('Ctrl Pts',(-6.26112587698772,4.2,5.37226655127787));
#15694=CARTESIAN_POINT('Ctrl Pts',(-6.46246210121964,-3.,5.46195513100446));
#15695=CARTESIAN_POINT('Ctrl Pts',(-6.46246210121964,4.2,5.46195513100446));
#15696=CARTESIAN_POINT('Ctrl Pts',(-6.66121503090592,-3.,5.54547963906637));
#15697=CARTESIAN_POINT('Ctrl Pts',(-6.66121503090592,4.2,5.54547963906637));
#15698=CARTESIAN_POINT('Ctrl Pts',(-6.8570997603751,-3.,5.62308582598972));
#15699=CARTESIAN_POINT('Ctrl Pts',(-6.8570997603751,4.2,5.62308582598972));
#15700=CARTESIAN_POINT('Ctrl Pts',(-7.04976847947249,-3.,5.69662713609756));
#15701=CARTESIAN_POINT('Ctrl Pts',(-7.04976847947249,4.2,5.69662713609756));
#15702=CARTESIAN_POINT('Ctrl Pts',(-7.23853768475,-3.,5.76979878895672));
#15703=CARTESIAN_POINT('Ctrl Pts',(-7.23853768475,4.2,5.76979878895672));
#15704=CARTESIAN_POINT('Ctrl Pts',(-7.42198551710617,-3.,5.84723737025949));
#15705=CARTESIAN_POINT('Ctrl Pts',(-7.42198551710617,4.2,5.84723737025949));
#15706=CARTESIAN_POINT('Ctrl Pts',(-7.59751903688412,-3.,5.93381436957244));
#15707=CARTESIAN_POINT('Ctrl Pts',(-7.59751903688412,4.2,5.93381436957244));
#15708=CARTESIAN_POINT('Ctrl Pts',(-7.76106756457753,-3.,6.03389995867283));
#15709=CARTESIAN_POINT('Ctrl Pts',(-7.76106756457753,4.2,6.03389995867283));
#15710=CARTESIAN_POINT('Ctrl Pts',(-7.90644860448901,-3.,6.15052660592937));
#15711=CARTESIAN_POINT('Ctrl Pts',(-7.90644860448901,4.2,6.15052660592937));
#15712=CARTESIAN_POINT('Ctrl Pts',(-8.02580908828117,-3.,6.28498018271686));
#15713=CARTESIAN_POINT('Ctrl Pts',(-8.02580908828117,4.2,6.28498018271686));
#15714=CARTESIAN_POINT('Ctrl Pts',(-8.11207116917861,-3.,6.43720976255636));
#15715=CARTESIAN_POINT('Ctrl Pts',(-8.11207116917861,4.2,6.43720976255636));
#15716=CARTESIAN_POINT('Ctrl Pts',(-8.16089752265956,-3.,6.60605451948903));
#15717=CARTESIAN_POINT('Ctrl Pts',(-8.16089752265956,4.2,6.60605451948903));
#15718=CARTESIAN_POINT('Ctrl Pts',(-8.17293082304181,-3.,6.78954489191904));
#15719=CARTESIAN_POINT('Ctrl Pts',(-8.17293082304181,4.2,6.78954489191904));
#15720=CARTESIAN_POINT('Ctrl Pts',(-8.15569042861244,-3.,6.9851692342788));
#15721=CARTESIAN_POINT('Ctrl Pts',(-8.15569042861244,4.2,6.9851692342788));
#15722=CARTESIAN_POINT('Ctrl Pts',(-8.12057943633387,-3.,7.19009032473164));
#15723=CARTESIAN_POINT('Ctrl Pts',(-8.12057943633387,4.2,7.19009032473164));
#15724=CARTESIAN_POINT('Ctrl Pts',(-8.08008348678073,-3.,7.40136016279791));
#15725=CARTESIAN_POINT('Ctrl Pts',(-8.08008348678073,4.2,7.40136016279791));
#15726=CARTESIAN_POINT('Ctrl Pts',(-8.04494633492831,-3.,7.61613341658677));
#15727=CARTESIAN_POINT('Ctrl Pts',(-8.04494633492831,4.2,7.61613341658677));
#15728=CARTESIAN_POINT('Ctrl Pts',(-8.02124364536279,-3.,7.83188673232793));
#15729=CARTESIAN_POINT('Ctrl Pts',(-8.02124364536279,4.2,7.83188673232793));
#15730=CARTESIAN_POINT('Ctrl Pts',(-8.007818938056,-3.,8.04662057355248));
#15731=CARTESIAN_POINT('Ctrl Pts',(-8.007818938056,4.2,8.04662057355248));
#15732=CARTESIAN_POINT('Ctrl Pts',(-7.99879843919661,-3.,8.25883677791483));
#15733=CARTESIAN_POINT('Ctrl Pts',(-7.99879843919661,4.2,8.25883677791483));
#15734=CARTESIAN_POINT('Ctrl Pts',(-7.98575825096101,-3.,8.46752658699528));
#15735=CARTESIAN_POINT('Ctrl Pts',(-7.98575825096101,4.2,8.46752658699528));
#15736=CARTESIAN_POINT('Ctrl Pts',(-7.96007609558389,-3.,8.67216210283896));
#15737=CARTESIAN_POINT('Ctrl Pts',(-7.96007609558389,4.2,8.67216210283896));
#15738=CARTESIAN_POINT('Ctrl Pts',(-7.91508259073019,-3.,8.87266947141823));
#15739=CARTESIAN_POINT('Ctrl Pts',(-7.91508259073019,4.2,8.87266947141823));
#15740=CARTESIAN_POINT('Ctrl Pts',(-7.84862074946261,-3.,9.06945407016992));
#15741=CARTESIAN_POINT('Ctrl Pts',(-7.84862074946261,4.2,9.06945407016992));
#15742=CARTESIAN_POINT('Ctrl Pts',(-7.76209282457479,-3.,9.26297089919765));
#15743=CARTESIAN_POINT('Ctrl Pts',(-7.76209282457479,4.2,9.26297089919765));
#15744=CARTESIAN_POINT('Ctrl Pts',(-7.65900038660722,-3.,9.4532499945042));
#15745=CARTESIAN_POINT('Ctrl Pts',(-7.65900038660722,4.2,9.4532499945042));
#15746=CARTESIAN_POINT('Ctrl Pts',(-7.5436057352653,-3.,9.63939026966035));
#15747=CARTESIAN_POINT('Ctrl Pts',(-7.5436057352653,4.2,9.63939026966035));
#15748=CARTESIAN_POINT('Ctrl Pts',(-7.41967047355001,-3.,9.81917361987397));
#15749=CARTESIAN_POINT('Ctrl Pts',(-7.41967047355001,4.2,9.81917361987397));
#15750=CARTESIAN_POINT('Ctrl Pts',(-7.28883796912703,-3.,9.98835756998572));
#15751=CARTESIAN_POINT('Ctrl Pts',(-7.28883796912703,4.2,9.98835756998572));
#15752=CARTESIAN_POINT('Ctrl Pts',(-7.15081550722306,-3.,10.1414720974148));
#15753=CARTESIAN_POINT('Ctrl Pts',(-7.15081550722306,4.2,10.1414720974148));
#15754=CARTESIAN_POINT('Ctrl Pts',(-7.0044544864105,-3.,10.2733319413008));
#15755=CARTESIAN_POINT('Ctrl Pts',(-7.0044544864105,4.2,10.2733319413008));
#15756=CARTESIAN_POINT('Ctrl Pts',(-6.84859008776113,-3.,10.3804015453596));
#15757=CARTESIAN_POINT('Ctrl Pts',(-6.84859008776113,4.2,10.3804015453596));
#15758=CARTESIAN_POINT('Ctrl Pts',(-6.68288828293938,-3.,10.4620502678778));
#15759=CARTESIAN_POINT('Ctrl Pts',(-6.68288828293938,4.2,10.4620502678778));
#15760=CARTESIAN_POINT('Ctrl Pts',(-6.50892555577766,-3.,10.522290883026));
#15761=CARTESIAN_POINT('Ctrl Pts',(-6.50892555577766,4.2,10.522290883026));
#15762=CARTESIAN_POINT('Ctrl Pts',(-6.32976796473811,-3.,10.5687216653902));
#15763=CARTESIAN_POINT('Ctrl Pts',(-6.32976796473811,4.2,10.5687216653902));
#15764=CARTESIAN_POINT('Ctrl Pts',(-6.14893768388701,-3.,10.6103475969885));
#15765=CARTESIAN_POINT('Ctrl Pts',(-6.14893768388701,4.2,10.6103475969885));
#15766=CARTESIAN_POINT('Ctrl Pts',(-5.96961932707142,-3.,10.6558377434043));
#15767=CARTESIAN_POINT('Ctrl Pts',(-5.96961932707142,4.2,10.6558377434043));
#15768=CARTESIAN_POINT('Ctrl Pts',(-5.79367695415031,-3.,10.7114411549114));
#15769=CARTESIAN_POINT('Ctrl Pts',(-5.79367695415031,4.2,10.7114411549114));
#15770=CARTESIAN_POINT('Ctrl Pts',(-5.62101499943431,-3.,10.7795199127535));
#15771=CARTESIAN_POINT('Ctrl Pts',(-5.62101499943431,4.2,10.7795199127535));
#15772=CARTESIAN_POINT('Ctrl Pts',(-5.45051506148982,-3.,10.8599381259737));
#15773=CARTESIAN_POINT('Ctrl Pts',(-5.45051506148982,4.2,10.8599381259737));
#15774=CARTESIAN_POINT('Ctrl Pts',(-5.28082876351929,-3.,10.9511663773826));
#15775=CARTESIAN_POINT('Ctrl Pts',(-5.28082876351929,4.2,10.9511663773826));
#15776=CARTESIAN_POINT('Ctrl Pts',(-5.11112998264616,-3.,11.0513704191329));
#15777=CARTESIAN_POINT('Ctrl Pts',(-5.11112998264616,4.2,11.0513704191329));
#15778=CARTESIAN_POINT('Ctrl Pts',(-4.94211773226973,-3.,11.1598106424589));
#15779=CARTESIAN_POINT('Ctrl Pts',(-4.94211773226973,4.2,11.1598106424589));
#15780=CARTESIAN_POINT('Ctrl Pts',(-4.77596612414951,-3.,11.2768795166235));
#15781=CARTESIAN_POINT('Ctrl Pts',(-4.77596612414951,4.2,11.2768795166235));
#15782=CARTESIAN_POINT('Ctrl Pts',(-4.61532593596946,-3.,11.4029224160731));
#15783=CARTESIAN_POINT('Ctrl Pts',(-4.61532593596946,4.2,11.4029224160731));
#15784=CARTESIAN_POINT('Ctrl Pts',(-4.46255574628757,-3.,11.5373242211527));
#15785=CARTESIAN_POINT('Ctrl Pts',(-4.46255574628757,4.2,11.5373242211527));
#15786=CARTESIAN_POINT('Ctrl Pts',(-4.3290607566988,-3.,11.6677566212747));
#15787=CARTESIAN_POINT('Ctrl Pts',(-4.3290607566988,4.2,11.6677566212747));
#15788=CARTESIAN_POINT('Ctrl Pts',(-4.22986670297865,-3.,11.7703786717728));
#15789=CARTESIAN_POINT('Ctrl Pts',(-4.22986670297865,4.2,11.7703786717728));
#15790=CARTESIAN_POINT('Ctrl Pts',(-4.15991130277621,-3.,11.842517268501));
#15791=CARTESIAN_POINT('Ctrl Pts',(-4.15991130277621,4.2,11.842517268501));
#15792=CARTESIAN_POINT('Ctrl Pts',(-4.11686402271798,-3.,11.8858809149481));
#15793=CARTESIAN_POINT('Ctrl Pts',(-4.11686402271798,4.2,11.8858809149481));
#15794=CARTESIAN_POINT('Ctrl Pts',(-4.1,-3.,11.9026515720683));
#15795=CARTESIAN_POINT('Ctrl Pts',(-4.1,4.2,11.9026515720683));
#15796=CARTESIAN_POINT('',(-4.15712386170579,0.0799999999999999,11.8450264384607));
#15797=CARTESIAN_POINT('Origin',(-4.01664557121473,1.77216539020708,11.7072473142283));
#15798=CARTESIAN_POINT('Ctrl Pts',(-4.0999999999998,0.08,11.9026515720685));
#15799=CARTESIAN_POINT('Ctrl Pts',(-4.11927627294061,0.08,11.8834820198536));
#15800=CARTESIAN_POINT('Ctrl Pts',(-4.13827843210557,0.08,11.8642474273099));
#15801=CARTESIAN_POINT('Ctrl Pts',(-4.15712386170576,0.08,11.8450264384607));
#15802=CARTESIAN_POINT('Ctrl Pts',(3.98763757557447,0.0893144327047665,
0.904932892569182));
#15803=CARTESIAN_POINT('Ctrl Pts',(3.98203476831165,0.080980516655767,0.901899655408594));
#15804=CARTESIAN_POINT('Ctrl Pts',(3.96967224365401,0.068894102459747,0.897500692078048));
#15805=CARTESIAN_POINT('Ctrl Pts',(3.94855499960848,0.0583913140546653,
0.893678342428863));
#15806=CARTESIAN_POINT('Ctrl Pts',(3.93547774845255,0.055477193409909,0.892617991958012));
#15807=CARTESIAN_POINT('Ctrl Pts',(3.9293765880439,0.0547985738896275,0.892371260600161));
#15808=CARTESIAN_POINT('Ctrl Pts',(3.98243005775679,0.0869928933912105,
0.916663912034212));
#15809=CARTESIAN_POINT('Ctrl Pts',(3.97744058496684,0.0790608728779208,
0.913329286844901));
#15810=CARTESIAN_POINT('Ctrl Pts',(3.96624502189315,0.0673244992554347,
0.908078805155286));
#15811=CARTESIAN_POINT('Ctrl Pts',(3.94633901956984,0.0568639390894838,
0.901649656409215));
#15812=CARTESIAN_POINT('Ctrl Pts',(3.93358166964479,0.0539712488488517,
0.898346678324299));
#15813=CARTESIAN_POINT('Ctrl Pts',(3.92751586915137,0.0536129422494931,
0.896239350875046));
#15814=CARTESIAN_POINT('Ctrl Pts',(3.97972958477838,0.0827272695427162,
0.929109421587075));
#15815=CARTESIAN_POINT('Ctrl Pts',(3.97493957450629,0.0750745480505631,
0.925223897697526));
#15816=CARTESIAN_POINT('Ctrl Pts',(3.96409914923351,0.0637718835013209,
0.918754898918153));
#15817=CARTESIAN_POINT('Ctrl Pts',(3.94450057092466,0.0540981768731819,
0.909481071136272));
#15818=CARTESIAN_POINT('Ctrl Pts',(3.93179086316711,0.0518251218281415,
0.903943073991344));
#15819=CARTESIAN_POINT('Ctrl Pts',(3.92569874356709,0.0520681029751514,
0.900018242283346));
#15820=CARTESIAN_POINT('Ctrl Pts',(3.97984798233949,0.0770101465833284,
0.94083226531257));
#15821=CARTESIAN_POINT('Ctrl Pts',(3.97479328383972,0.0694388470342489,
0.936335429667805));
#15822=CARTESIAN_POINT('Ctrl Pts',(3.96340956460396,0.0585229907363136,
0.928669651644793));
#15823=CARTESIAN_POINT('Ctrl Pts',(3.9431247884684,0.0502165408921483,0.916833416299925));
#15824=CARTESIAN_POINT('Ctrl Pts',(3.93014957889597,0.0490851008089254,
0.909289140537019));
#15825=CARTESIAN_POINT('Ctrl Pts',(3.92395044195663,0.0501855062839886,
0.903655465216232));
#15826=CARTESIAN_POINT('',(3.98750649384402,0.089362716860748,0.904960783852724));
#15827=CARTESIAN_POINT('',(3.97983671972002,0.0769932827027835,0.940822248119245));
#15828=CARTESIAN_POINT('Origin',(4.04916946954199,0.0413995564077306,0.922765214848074));
#15829=CARTESIAN_POINT('',(3.92397049706406,0.0501819523054353,0.903673683563879));
#15830=CARTESIAN_POINT('Ctrl Pts',(3.97983671972021,0.0769932826936726,
0.940822248137924));
#15831=CARTESIAN_POINT('Ctrl Pts',(3.9747831370112,0.0694291188139783,0.936328597068607));
#15832=CARTESIAN_POINT('Ctrl Pts',(3.96340310875481,0.0585203471189109,
0.92866588463502));
#15833=CARTESIAN_POINT('Ctrl Pts',(3.94313104090131,0.0502191012122621,
0.916837064615631));
#15834=CARTESIAN_POINT('Ctrl Pts',(3.93016357755921,0.049086322581369,0.909297279894274));
#15835=CARTESIAN_POINT('Ctrl Pts',(3.92397049706405,0.0501819523054367,
0.903673683563877));
#15836=CARTESIAN_POINT('',(3.929394405843,0.0548135766059198,0.892377353749379));
#15837=CARTESIAN_POINT('Origin',(3.9387684725109,-0.0223136011303559,0.873253054794691));
#15838=CARTESIAN_POINT('Ctrl Pts',(3.929394405843,0.0548135766059198,0.892377353749379));
#15839=CARTESIAN_POINT('Ctrl Pts',(3.93294284341525,0.0552167805124275,
0.892524159568853));
#15840=CARTESIAN_POINT('Ctrl Pts',(3.93664094497026,0.0558681664406091,
0.892761271875184));
#15841=CARTESIAN_POINT('Ctrl Pts',(3.94035177870644,0.0567901148977748,
0.893096851090279));
#15842=CARTESIAN_POINT('Ctrl Pts',(3.9430125834771,0.0574511859743905,0.893337473775081));
#15843=CARTESIAN_POINT('Ctrl Pts',(3.94567955148932,0.0582503453705328,
0.893628363566722));
#15844=CARTESIAN_POINT('Ctrl Pts',(3.94830258562972,0.0591802781982167,
0.89396684560707));
#15845=CARTESIAN_POINT('Ctrl Pts',(3.95411448629012,0.0612407459336948,
0.894716825930824));
#15846=CARTESIAN_POINT('Ctrl Pts',(3.95972301416291,0.0639386192551732,
0.895698385030791));
#15847=CARTESIAN_POINT('Ctrl Pts',(3.96496846008119,0.0672806009961073,
0.896914467460389));
#15848=CARTESIAN_POINT('Ctrl Pts',(3.9653920120109,0.0675504546629755,0.897012661983364));
#15849=CARTESIAN_POINT('Ctrl Pts',(3.96581317192551,0.0678245213626311,
0.897112391282691));
#15850=CARTESIAN_POINT('Ctrl Pts',(3.96623184176758,0.0681028114885871,
0.897213659854605));
#15851=CARTESIAN_POINT('Ctrl Pts',(3.96747264480673,0.0689275741042759,
0.897513787399455));
#15852=CARTESIAN_POINT('Ctrl Pts',(3.9686909782428,0.0697890488164992,0.897827314561264));
#15853=CARTESIAN_POINT('Ctrl Pts',(3.96988312090337,0.0706865001004049,
0.898154007323679));
#15854=CARTESIAN_POINT('Ctrl Pts',(3.97453898522749,0.0741914593251504,
0.899429892524157));
#15855=CARTESIAN_POINT('Ctrl Pts',(3.97879291378003,0.0782485705570666,
0.900907911202756));
#15856=CARTESIAN_POINT('Ctrl Pts',(3.98252105307226,0.0827084187352409,
0.902532503084932));
#15857=CARTESIAN_POINT('Ctrl Pts',(3.98430255563518,0.084839570587914,0.903308819197324));
#15858=CARTESIAN_POINT('Ctrl Pts',(3.98596444849724,0.0870620466537864,
0.904118357281442));
#15859=CARTESIAN_POINT('Ctrl Pts',(3.98749614255641,0.089356831788631,0.90495397253418));
#15860=CARTESIAN_POINT('Ctrl Pts',(3.99995017471379,0.126799874999198,0.918578169368801));
#15861=CARTESIAN_POINT('Ctrl Pts',(3.99944986938898,0.11348851535217,0.913733230679671));
#15862=CARTESIAN_POINT('Ctrl Pts',(3.99505715576901,0.100344093242609,0.90894905228516));
#15863=CARTESIAN_POINT('Ctrl Pts',(3.98762439168473,0.0892955579769557,
0.904927714316222));
#15864=CARTESIAN_POINT('Ctrl Pts',(3.99313598197604,0.122218533523161,0.930421158791107));
#15865=CARTESIAN_POINT('Ctrl Pts',(3.99279640530477,0.109784526212468,0.925839927766699));
#15866=CARTESIAN_POINT('Ctrl Pts',(3.98903809825174,0.0974908830262579,
0.921079001953896));
#15867=CARTESIAN_POINT('Ctrl Pts',(3.98241869839885,0.0869748432979465,
0.916657600142957));
#15868=CARTESIAN_POINT('Ctrl Pts',(3.98984275968184,0.116883323642803,0.943973826544633));
#15869=CARTESIAN_POINT('Ctrl Pts',(3.98959331650047,0.104765282119502,0.939370198048702));
#15870=CARTESIAN_POINT('Ctrl Pts',(3.98607384319811,0.0928557239444475,
0.934253508985834));
#15871=CARTESIAN_POINT('Ctrl Pts',(3.97971891715341,0.0827099677051683,
0.929101291873573));
#15872=CARTESIAN_POINT('Ctrl Pts',(3.99053121895996,0.111540623934062,0.957340198321923));
#15873=CARTESIAN_POINT('Ctrl Pts',(3.99028017432925,0.0991190831119013,
0.952466190557957));
#15874=CARTESIAN_POINT('Ctrl Pts',(3.98654272619743,0.0870307818092068,
0.946785236162934));
#15875=CARTESIAN_POINT('Ctrl Pts',(3.97983671972021,0.0769932826936736,
0.940822248137926));
#15876=CARTESIAN_POINT('',(3.99994696244202,0.126799890819684,0.918578279225942));
#15877=CARTESIAN_POINT('',(3.99053121895996,0.111540623934062,0.957340198321923));
#15878=CARTESIAN_POINT('Origin',(4.07042531154701,0.111540623934061,0.953225107837748));
#15879=CARTESIAN_POINT('Ctrl Pts',(3.99053121895996,0.111540623934062,0.957340198321923));
#15880=CARTESIAN_POINT('Ctrl Pts',(3.99028017432925,0.0991190831119013,
0.952466190557957));
#15881=CARTESIAN_POINT('Ctrl Pts',(3.98654272619743,0.0870307818092068,
0.946785236162934));
#15882=CARTESIAN_POINT('Ctrl Pts',(3.97983671972021,0.0769932826936736,
0.940822248137926));
#15883=CARTESIAN_POINT('Origin',(3.9367321686135,0.121247013319355,0.916540496718191));
#15884=CARTESIAN_POINT('Ctrl Pts',(3.92939607642122,0.0548006123101191,
0.892372580860866));
#15885=CARTESIAN_POINT('Ctrl Pts',(3.92634388981074,0.0544603574102712,
0.892248738205258));
#15886=CARTESIAN_POINT('Ctrl Pts',(3.92326758436874,0.0542854221831822,
0.892185066989672));
#15887=CARTESIAN_POINT('Ctrl Pts',(3.92012020332128,0.0542767513583031,
0.892181911067511));
#15888=CARTESIAN_POINT('Ctrl Pts',(3.92004146981349,0.0542766412926813,
0.892181871006901));
#15889=CARTESIAN_POINT('Ctrl Pts',(3.9199627360209,0.0542766412926813,0.892181871006901));
#15890=CARTESIAN_POINT('Ctrl Pts',(3.92753533006471,0.0536139664579581,
0.896246505841524));
#15891=CARTESIAN_POINT('Ctrl Pts',(3.92511894507891,0.05359185050338,0.894857113199761));
#15892=CARTESIAN_POINT('Ctrl Pts',(3.92263409808172,0.0538017795257374,
0.893523976721591));
#15893=CARTESIAN_POINT('Ctrl Pts',(3.92009002060122,0.0542535960747209,
0.892245667428479));
#15894=CARTESIAN_POINT('Ctrl Pts',(3.92002637871827,0.0542650414753612,
0.892213741243058));
#15895=CARTESIAN_POINT('Ctrl Pts',(3.9199627360209,0.0542766412926813,0.892181871006901));
#15896=CARTESIAN_POINT('Ctrl Pts',(3.92571837401383,0.0520672372167076,
0.900031098340516));
#15897=CARTESIAN_POINT('Ctrl Pts',(3.92389518151557,0.0525997003708216,
0.89742148095101));
#15898=CARTESIAN_POINT('Ctrl Pts',(3.92200062309269,0.0533123669048904,
0.894860812183919));
#15899=CARTESIAN_POINT('Ctrl Pts',(3.92005983815835,0.0542303656386634,
0.892309396431305));
#15900=CARTESIAN_POINT('Ctrl Pts',(3.92001128762305,0.054253441658041,0.892245611479215));
#15901=CARTESIAN_POINT('Ctrl Pts',(3.9199627360209,0.0542766412926813,0.892181871006901));
#15902=CARTESIAN_POINT('Ctrl Pts',(3.92397049706405,0.0501819523054441,
0.903673683563853));
#15903=CARTESIAN_POINT('Ctrl Pts',(3.92267324571416,0.0514837668071902,
0.899940280902761));
#15904=CARTESIAN_POINT('Ctrl Pts',(3.92136717122144,0.0528172498522682,
0.896195564980704));
#15905=CARTESIAN_POINT('Ctrl Pts',(3.92002965606137,0.054207059082659,0.892373097632133));
#15906=CARTESIAN_POINT('Ctrl Pts',(3.91999619652783,0.0542418418407209,
0.892277481715372));
#15907=CARTESIAN_POINT('Ctrl Pts',(3.9199627360209,0.0542766412926813,0.892181871006901));
#15908=CARTESIAN_POINT('',(3.91996276391134,0.0542766409928811,0.892181871823741));
#15909=CARTESIAN_POINT('Origin',(3.89398158889879,0.447015786354718,1.02337823064183));
#15910=CARTESIAN_POINT('Origin',(3.91993477835724,0.128120482093708,0.919068001247204));
#15911=CARTESIAN_POINT('Ctrl Pts',(4.,0.129452050955555,0.919543482472952));
#15912=CARTESIAN_POINT('Ctrl Pts',(4.,0.128568366080467,0.919221847481949));
#15913=CARTESIAN_POINT('Ctrl Pts',(3.99998336677459,0.127682998637521,0.918899600086328));
#15914=CARTESIAN_POINT('Ctrl Pts',(3.99995017471379,0.126799874999197,0.918578169368801));
#15915=CARTESIAN_POINT('Ctrl Pts',(3.99320174100155,0.125572492169931,0.931636190695047));
#15916=CARTESIAN_POINT('Ctrl Pts',(3.99318664336971,0.124450242215544,0.931244569432182));
#15917=CARTESIAN_POINT('Ctrl Pts',(3.99316471933781,0.123330766671213,0.930839013626173));
#15918=CARTESIAN_POINT('Ctrl Pts',(3.99313598197604,0.122218533523161,0.930421158791108));
#15919=CARTESIAN_POINT('Ctrl Pts',(3.98992351495583,0.121055159551916,0.945479161641182));
#15920=CARTESIAN_POINT('Ctrl Pts',(3.98989830405354,0.119653684370202,0.945009099951952));
#15921=CARTESIAN_POINT('Ctrl Pts',(3.98987138440309,0.118261520219538,0.944506745566704));
#15922=CARTESIAN_POINT('Ctrl Pts',(3.98984275968184,0.116883323642802,0.943973826544634));
#15923=CARTESIAN_POINT('Ctrl Pts',(3.99062355969946,0.116531496051876,0.959137393584632));
#15924=CARTESIAN_POINT('Ctrl Pts',(3.99059540935326,0.114850322896056,0.958588165894169));
#15925=CARTESIAN_POINT('Ctrl Pts',(3.9905646125374,0.11318519078342,0.957988531469827));
#15926=CARTESIAN_POINT('Ctrl Pts',(3.99053121895996,0.111540623934061,0.957340198321925));
#15927=CARTESIAN_POINT('',(4.,0.129452050955555,0.919543482472952));
#15928=CARTESIAN_POINT('Origin',(3.92338073148591,0.121553580080691,0.916815722371178));
#15929=CARTESIAN_POINT('',(3.99062355969947,0.116531496051876,0.959137393584632));
#15930=CARTESIAN_POINT('Origin',(4.07051868566465,0.116531496051876,0.955042415317635));
#15931=CARTESIAN_POINT('Origin',(3.98841540917197,0.128777749562786,0.917370672555525));
#15932=CARTESIAN_POINT('Ctrl Pts',(4.,0.524122951685637,1.06319194266973));
#15933=CARTESIAN_POINT('Ctrl Pts',(4.,0.392579508521167,1.01531404484498));
#15934=CARTESIAN_POINT('Ctrl Pts',(4.,0.261012992948574,0.967427749350433));
#15935=CARTESIAN_POINT('Ctrl Pts',(4.,0.129452050955556,0.919543482472952));
#15936=CARTESIAN_POINT('Ctrl Pts',(3.99722173585145,0.521464639036904,1.07150653805471));
#15937=CARTESIAN_POINT('Ctrl Pts',(3.99608172587457,0.389414444976033,1.02512218732467));
#15938=CARTESIAN_POINT('Ctrl Pts',(3.99478956593868,0.257458496604602,0.978440228041136));
#15939=CARTESIAN_POINT('Ctrl Pts',(3.99320174100156,0.125572492169931,0.931636190695047));
#15940=CARTESIAN_POINT('Ctrl Pts',(3.99595792658054,0.518642023625072,1.08027231824298));
#15941=CARTESIAN_POINT('Ctrl Pts',(3.99426602664426,0.385984032905188,1.03565889431257));
#15942=CARTESIAN_POINT('Ctrl Pts',(3.99232735107637,0.253495283774764,0.99057504228606));
#15943=CARTESIAN_POINT('Ctrl Pts',(3.98992351495583,0.121055159551917,0.945479161641181));
#15944=CARTESIAN_POINT('Ctrl Pts',(3.99628184601446,0.515818756594824,1.08898105602234));
#15945=CARTESIAN_POINT('Ctrl Pts',(3.99468731422838,0.38255220960787,1.04611126263635));
#15946=CARTESIAN_POINT('Ctrl Pts',(3.99285055050703,0.249530114845418,1.00258712627989));
#15947=CARTESIAN_POINT('Ctrl Pts',(3.99062355969947,0.116531496051877,0.959137393584631));
#15948=CARTESIAN_POINT('',(4.,0.524122951685637,1.06319194266973));
#15949=CARTESIAN_POINT('',(3.99628071248376,0.515724022809955,1.08895058147547));
#15950=CARTESIAN_POINT('Ctrl Pts',(4.,0.524122951685637,1.06319194266973));
#15951=CARTESIAN_POINT('Ctrl Pts',(3.9986089924126,0.522629326334401,1.06729564459538));
#15952=CARTESIAN_POINT('Ctrl Pts',(3.99759863687363,0.521165724744202,1.07152731239861));
#15953=CARTESIAN_POINT('Ctrl Pts',(3.99697497557878,0.519756336372472,1.07584372036492));
#15954=CARTESIAN_POINT('Ctrl Pts',(3.99635088558503,0.518345979200444,1.08016309538943));
#15955=CARTESIAN_POINT('Ctrl Pts',(3.99611691668579,0.516996538273542,1.084547162494));
#15956=CARTESIAN_POINT('Ctrl Pts',(3.99628071248508,0.515724022802589,1.08895058149858));
#15957=CARTESIAN_POINT('Ctrl Pts',(3.99628071248508,0.515724022802589,1.08895058149858));
#15958=CARTESIAN_POINT('Ctrl Pts',(3.99468644375212,0.382489169567759,1.04609063626742));
#15959=CARTESIAN_POINT('Ctrl Pts',(3.99285002281427,0.249498600387411,1.00257683072353));
#15960=CARTESIAN_POINT('Ctrl Pts',(3.99062355969947,0.116531496051877,0.959137393584631));
#15961=CARTESIAN_POINT('',(4.,0.0542766412926824,0.892181871006898));
#15962=CARTESIAN_POINT('Ctrl Pts',(3.99784434068601,0.000813388873467947,
1.16174107276121));
#15963=CARTESIAN_POINT('Ctrl Pts',(3.99784432727272,0.0008135747227017,
1.16174071881185));
#15964=CARTESIAN_POINT('Ctrl Pts',(3.9958522274879,0.00126345588851946,
1.15121922616146));
#15965=CARTESIAN_POINT('Ctrl Pts',(3.99078965828379,0.00281482454399863,
1.12710950869973));
#15966=CARTESIAN_POINT('Ctrl Pts',(3.98313335463591,0.00589478809278018,
1.0946626330386));
#15967=CARTESIAN_POINT('Ctrl Pts',(3.96225979086675,0.0168110800211123,
1.01686469965838));
#15968=CARTESIAN_POINT('Ctrl Pts',(3.94114259504174,0.0329494505434504,
0.953093833553903));
#15969=CARTESIAN_POINT('Ctrl Pts',(3.92397049706406,0.0501819523054334,
0.903673683563887));
#15970=CARTESIAN_POINT('Ctrl Pts',(3.9982278284976,0.000727245993550886,
1.16376965450937));
#15971=CARTESIAN_POINT('Ctrl Pts',(3.99822932035433,0.00181436044573403,
1.16381581953223));
#15972=CARTESIAN_POINT('Ctrl Pts',(3.99679023674084,0.00394535585146101,
1.15344065726723));
#15973=CARTESIAN_POINT('Ctrl Pts',(3.99313422044013,0.00741388714452286,
1.12958158728165));
#15974=CARTESIAN_POINT('Ctrl Pts',(3.98757564687094,0.0119616813045604,
1.09733717910204));
#15975=CARTESIAN_POINT('Ctrl Pts',(3.97223449897184,0.0244847572237893,
1.01956065811568));
#15976=CARTESIAN_POINT('Ctrl Pts',(3.95599704952542,0.0389933222701742,
0.954854087536785));
#15977=CARTESIAN_POINT('Ctrl Pts',(3.94181237515934,0.0536467548616993,
0.904095794994089));
#15978=CARTESIAN_POINT('Ctrl Pts',(3.99883736539415,0.000553542649297133,
1.16785724348145));
#15979=CARTESIAN_POINT('Ctrl Pts',(3.9988418299182,0.00382806012798106,
1.16799630117926));
#15980=CARTESIAN_POINT('Ctrl Pts',(3.99824607010187,0.00936410973956307,
1.15796429058724));
#15981=CARTESIAN_POINT('Ctrl Pts',(3.99675628178266,0.0169794272648916,
1.1347803839048));
#15982=CARTESIAN_POINT('Ctrl Pts',(3.99453093968089,0.0251577732975947,
1.10326524512036));
#15983=CARTESIAN_POINT('Ctrl Pts',(3.98837066180094,0.0436242941790727,
1.02669421700478));
#15984=CARTESIAN_POINT('Ctrl Pts',(3.98165970299104,0.0589291697315894,
0.961716549736144));
#15985=CARTESIAN_POINT('Ctrl Pts',(3.97502664104943,0.0722507173702981,
0.909843629936585));
#15986=CARTESIAN_POINT('Ctrl Pts',(3.99912832044927,0.000378790238046,1.17197973040507));
#15987=CARTESIAN_POINT('Ctrl Pts',(3.99913571708803,0.00585391903912836,
1.17221224354204));
#15988=CARTESIAN_POINT('Ctrl Pts',(3.99882664657299,0.0148542262907823,
1.16259013266621));
#15989=CARTESIAN_POINT('Ctrl Pts',(3.9980956580057,0.026941094118525,1.14028756032799));
#15990=CARTESIAN_POINT('Ctrl Pts',(3.99704746786599,0.0395222742335762,
1.10990521749973));
#15991=CARTESIAN_POINT('Ctrl Pts',(3.99432345688666,0.0669108953728227,
1.03597240480608));
#15992=CARTESIAN_POINT('Ctrl Pts',(3.99146441961465,0.0882021911235168,
0.973040771868915));
#15993=CARTESIAN_POINT('Ctrl Pts',(3.98866790214921,0.10584241001414,0.922799195037908));
#15994=CARTESIAN_POINT('Ctrl Pts',(3.99919371386846,0.000291414002863247,
1.1740435121275));
#15995=CARTESIAN_POINT('Ctrl Pts',(3.99920256193258,0.00686684929623559,
1.17432275235113));
#15996=CARTESIAN_POINT('Ctrl Pts',(3.99890451851341,0.0175976878297955,
1.16490897998439));
#15997=CARTESIAN_POINT('Ctrl Pts',(3.99819220127434,0.0319198582513071,
1.14305909112717));
#15998=CARTESIAN_POINT('Ctrl Pts',(3.99717818807624,0.0466981217662143,
1.11326101887131));
#15999=CARTESIAN_POINT('Ctrl Pts',(3.99451765518903,0.0785527702394917,
1.0407191721013));
#16000=CARTESIAN_POINT('Ctrl Pts',(3.99178846069233,0.10282206024219,0.978899329348002));
#16001=CARTESIAN_POINT('Ctrl Pts',(3.98904904336713,0.122677505741229,0.929651197081971));
#16002=CARTESIAN_POINT('',(3.99919381669006,0.00037425564854435,1.17404675699404));
#16003=CARTESIAN_POINT('Ctrl Pts',(3.99053162689604,0.111552033777857,0.957344809613607));
#16004=CARTESIAN_POINT('Ctrl Pts',(3.99259503042251,0.0954962439419094,
0.99739900732689));
#16005=CARTESIAN_POINT('Ctrl Pts',(3.99484994314364,0.0745742755413206,
1.04977930513061));
#16006=CARTESIAN_POINT('Ctrl Pts',(3.99717818807624,0.0466981217662143,
1.11326101887131));
#16007=CARTESIAN_POINT('Ctrl Pts',(3.99819220127434,0.0319198582513071,
1.14305909112717));
#16008=CARTESIAN_POINT('Ctrl Pts',(3.99890376983111,0.0176127411724394,
1.16488601461992));
#16009=CARTESIAN_POINT('Ctrl Pts',(3.99920130863952,0.00691194818962238,
1.17428316822488));
#16010=CARTESIAN_POINT('Ctrl Pts',(3.99919381710518,0.000374283339306366,
1.17404677002645));
#16011=CARTESIAN_POINT('',(3.99784430834598,0.000813481663902603,1.16174090062732));
#16012=CARTESIAN_POINT('Origin',(3.91983487919139,0.00718513856492471,1.17675789077508));
#16013=CARTESIAN_POINT('Ctrl Pts',(3.99784427600595,0.000813574454337259,
1.16174072849342));
#16014=CARTESIAN_POINT('Ctrl Pts',(3.99784273578734,0.000813920976441579,
1.16173258218817));
#16015=CARTESIAN_POINT('Ctrl Pts',(3.99784119332941,0.000814267840078317,
1.16172443633252));
#16016=CARTESIAN_POINT('Ctrl Pts',(3.99783965031257,0.000814614752868342,
1.16171629060187));
#16017=CARTESIAN_POINT('Ctrl Pts',(3.99783810729574,0.000814961665658368,
1.16170814487122));
#16018=CARTESIAN_POINT('Ctrl Pts',(3.9978365635392,0.000815308692277274,
1.16169999930219));
#16019=CARTESIAN_POINT('Ctrl Pts',(3.99783501934031,0.000815655834302155,
1.16169185383936));
#16020=CARTESIAN_POINT('Ctrl Pts',(3.99783193094253,0.000816350118351918,
1.16167556291369));
#16021=CARTESIAN_POINT('Ctrl Pts',(3.99782884075641,0.000817044867590349,
1.16165927241632));
#16022=CARTESIAN_POINT('Ctrl Pts',(3.99782574942695,0.000817740093563617,
1.16164298222655));
#16023=CARTESIAN_POINT('Ctrl Pts',(3.99781956676803,0.000819130545510153,
1.161610401847));
#16024=CARTESIAN_POINT('Ctrl Pts',(3.99781337941355,0.00082052164669327,
1.16157782264312));
#16025=CARTESIAN_POINT('Ctrl Pts',(3.99780720576951,0.000821928804838678,
1.16154533134384));
#16026=CARTESIAN_POINT('Ctrl Pts',(3.99779485848145,0.000824743121129494,
1.16148034874528));
#16027=CARTESIAN_POINT('Ctrl Pts',(3.99778250361156,0.000827582818338727,
1.16141539269024));
#16028=CARTESIAN_POINT('Ctrl Pts',(3.99777013683724,0.000830435889113772,
1.1613504218586));
#16029=CARTESIAN_POINT('Ctrl Pts',(3.9977234002965,0.000841218220467512,
1.16110488394862));
#16030=CARTESIAN_POINT('Ctrl Pts',(3.99767648280878,0.000852133710343159,
1.16085906292802));
#16031=CARTESIAN_POINT('Ctrl Pts',(3.99762845973455,0.000863380424841601,
1.16060793645995));
#16032=CARTESIAN_POINT('Ctrl Pts',(3.99756970142126,0.000877141267617072,
1.160300672339));
#16033=CARTESIAN_POINT('Ctrl Pts',(3.99751198108985,0.000890770026660122,
1.15999957986487));
#16034=CARTESIAN_POINT('Ctrl Pts',(3.99745532005822,0.000904237073150987,
1.15970459222681));
#16035=CARTESIAN_POINT('Ctrl Pts',(3.99741296186454,0.000914304658353342,
1.15948406776497));
#16036=CARTESIAN_POINT('Ctrl Pts',(3.99737009284839,0.000924544502561343,
1.1592612178845));
#16037=CARTESIAN_POINT('Ctrl Pts',(3.99732664050266,0.000934975402716219,
1.15903567313117));
#16038=CARTESIAN_POINT('Ctrl Pts',(3.99721602020136,0.00096153022498384,
1.15846148483017));
#16039=CARTESIAN_POINT('Ctrl Pts',(3.99710528340557,0.000988442107634933,
1.15788883833414));
#16040=CARTESIAN_POINT('Ctrl Pts',(3.99699448762094,0.00101568823936224,
1.15731795844143));
#16041=CARTESIAN_POINT('Ctrl Pts',(3.99683542048025,0.00105480492853115,
1.15649835837712));
#16042=CARTESIAN_POINT('Ctrl Pts',(3.99667448325672,0.00109504469120612,
1.15567341858394));
#16043=CARTESIAN_POINT('Ctrl Pts',(3.99651353174244,0.00113600838460423,
1.15485305488917));
#16044=CARTESIAN_POINT('Ctrl Pts',(3.99625082685399,0.00120286928089424,
1.15351405814923));
#16045=CARTESIAN_POINT('Ctrl Pts',(3.99598541481855,0.00127229923616561,
1.15217339875294));
#16046=CARTESIAN_POINT('Ctrl Pts',(3.99571743128359,0.0013449066789999,
1.15083588464134));
#16047=CARTESIAN_POINT('Ctrl Pts',(3.99519502051448,0.00148644862134294,
1.14822851633478));
#16048=CARTESIAN_POINT('Ctrl Pts',(3.99466155494466,0.00164050954618525,
1.1456272130292));
#16049=CARTESIAN_POINT('Ctrl Pts',(3.99411896967372,0.00180574117961086,
1.14303238119294));
#16050=CARTESIAN_POINT('Ctrl Pts',(3.99341629071535,0.00201972559511968,
1.13967192555673));
#16051=CARTESIAN_POINT('Ctrl Pts',(3.99269813258433,0.00225249187749216,
1.13632143548993));
#16052=CARTESIAN_POINT('Ctrl Pts',(3.99196676110863,0.00250303256209103,
1.1329829561429));
#16053=CARTESIAN_POINT('Ctrl Pts',(3.99105452080383,0.00281553218516866,
1.12881886782618));
#16054=CARTESIAN_POINT('Ctrl Pts',(3.99012140143879,0.00315586692512113,
1.12467248508852));
#16055=CARTESIAN_POINT('Ctrl Pts',(3.98917086800784,0.00352214531426548,
1.12054686155091));
#16056=CARTESIAN_POINT('Ctrl Pts',(3.98870515989402,0.00370160119891811,
1.11852553721503));
#16057=CARTESIAN_POINT('Ctrl Pts',(3.98823550683287,0.0038871810438387,
1.11651018939739));
#16058=CARTESIAN_POINT('Ctrl Pts',(3.98775852062678,0.00408030873675932,
1.11448575646417));
#16059=CARTESIAN_POINT('Ctrl Pts',(3.9862084876943,0.00470790400130428,
1.10790708044385));
#16060=CARTESIAN_POINT('Ctrl Pts',(3.98459064329944,0.00541159016947844,
1.10127461612058));
#16061=CARTESIAN_POINT('Ctrl Pts',(3.98292515171806,0.00618848637705155,
1.09466884705581));
#16062=CARTESIAN_POINT('Ctrl Pts',(3.97963238984024,0.0077244498390748,
1.08160890439789));
#16063=CARTESIAN_POINT('Ctrl Pts',(3.97615366065642,0.00954620024828415,
1.06865218726209));
#16064=CARTESIAN_POINT('Ctrl Pts',(3.9725476703773,0.0116345924802287,1.05580609615032));
#16065=CARTESIAN_POINT('Ctrl Pts',(3.96631447912973,0.0152445157395957,
1.03360078318899));
#16066=CARTESIAN_POINT('Ctrl Pts',(3.95970190268761,0.0196489544111943,
1.01172528029353));
#16067=CARTESIAN_POINT('Ctrl Pts',(3.95284326123313,0.024832861200458,0.990102320899307));
#16068=CARTESIAN_POINT('Ctrl Pts',(3.94567549386735,0.0302504119148388,
0.967504792842701));
#16069=CARTESIAN_POINT('Ctrl Pts',(3.93823747405201,0.0365191099549545,
0.945182309268941));
#16070=CARTESIAN_POINT('Ctrl Pts',(3.93065896302406,0.0436712823961812,
0.923055906994704));
#16071=CARTESIAN_POINT('Ctrl Pts',(3.92844049782574,0.0457649450687984,
0.916578822877736));
#16072=CARTESIAN_POINT('Ctrl Pts',(3.92620993731492,0.0479346347022567,
0.910118642894705));
#16073=CARTESIAN_POINT('Ctrl Pts',(3.92397049706406,0.0501819523054339,
0.903673683563887));
#16074=CARTESIAN_POINT('Ctrl Pts',(4.00794703095364,-0.208000000000001,
1.48914872207946));
#16075=CARTESIAN_POINT('Ctrl Pts',(4.00794703095364,0.891200000000001,1.48914872207946));
#16076=CARTESIAN_POINT('Ctrl Pts',(4.00765497692301,-0.208000000000001,
1.47837060024778));
#16077=CARTESIAN_POINT('Ctrl Pts',(4.00765497692301,0.891200000000001,1.47837060024778));
#16078=CARTESIAN_POINT('Ctrl Pts',(4.00609251232828,-0.208000000000001,
1.42037324240448));
#16079=CARTESIAN_POINT('Ctrl Pts',(4.00609251232828,0.891200000000001,1.42037324240448));
#16080=CARTESIAN_POINT('Ctrl Pts',(4.00332489658119,-0.208000000000001,
1.31493320069941));
#16081=CARTESIAN_POINT('Ctrl Pts',(4.00332489658119,0.891200000000001,1.31493320069941));
#16082=CARTESIAN_POINT('Ctrl Pts',(3.99926045685694,-0.208000000000001,
1.16206588280709));
#16083=CARTESIAN_POINT('Ctrl Pts',(3.99926045685694,0.891200000000001,1.16206588280709));
#16084=CARTESIAN_POINT('Ctrl Pts',(3.99260375067002,-0.208000000000001,
0.964078729991153));
#16085=CARTESIAN_POINT('Ctrl Pts',(3.99260375067002,0.891200000000001,0.964078729991153));
#16086=CARTESIAN_POINT('Ctrl Pts',(3.97841403016118,-0.208000000000001,
0.741129277895168));
#16087=CARTESIAN_POINT('Ctrl Pts',(3.97841403016118,0.891200000000001,0.741129277895168));
#16088=CARTESIAN_POINT('Ctrl Pts',(3.95259200169988,-0.208000000000001,
0.538436816836329));
#16089=CARTESIAN_POINT('Ctrl Pts',(3.95259200169988,0.891200000000001,0.538436816836329));
#16090=CARTESIAN_POINT('Ctrl Pts',(3.90986572419832,-0.208000000000001,
0.364350357241537));
#16091=CARTESIAN_POINT('Ctrl Pts',(3.90986572419832,0.891200000000001,0.364350357241537));
#16092=CARTESIAN_POINT('Ctrl Pts',(3.84598208672298,-0.208000000000001,
0.224659532804428));
#16093=CARTESIAN_POINT('Ctrl Pts',(3.84598208672298,0.891200000000001,0.224659532804428));
#16094=CARTESIAN_POINT('Ctrl Pts',(3.75872318140661,-0.208000000000001,
0.120497232333236));
#16095=CARTESIAN_POINT('Ctrl Pts',(3.75872318140661,0.891200000000001,0.120497232333236));
#16096=CARTESIAN_POINT('Ctrl Pts',(3.64881642260075,-0.208000000000001,
0.0470540298718229));
#16097=CARTESIAN_POINT('Ctrl Pts',(3.64881642260075,0.891200000000001,0.0470540298718229));
#16098=CARTESIAN_POINT('Ctrl Pts',(3.52045328348988,-0.208000000000001,
-0.00118366394786523));
#16099=CARTESIAN_POINT('Ctrl Pts',(3.52045328348988,0.891200000000001,-0.00118366394786523));
#16100=CARTESIAN_POINT('Ctrl Pts',(3.3816469894381,-0.208000000000001,-0.0263068037111615));
#16101=CARTESIAN_POINT('Ctrl Pts',(3.3816469894381,0.891200000000001,-0.0263068037111615));
#16102=CARTESIAN_POINT('Ctrl Pts',(3.2451100102617,-0.208000000000001,-0.0214179570895094));
#16103=CARTESIAN_POINT('Ctrl Pts',(3.2451100102617,0.891200000000001,-0.0214179570895094));
#16104=CARTESIAN_POINT('Ctrl Pts',(3.12452733970665,-0.208000000000001,
0.0241851999814078));
#16105=CARTESIAN_POINT('Ctrl Pts',(3.12452733970665,0.891200000000001,0.0241851999814078));
#16106=CARTESIAN_POINT('Ctrl Pts',(3.03063129752059,-0.208000000000001,
0.119017371327004));
#16107=CARTESIAN_POINT('Ctrl Pts',(3.03063129752059,0.891200000000001,0.119017371327004));
#16108=CARTESIAN_POINT('Ctrl Pts',(2.96639254265844,-0.208000000000001,
0.262319630540593));
#16109=CARTESIAN_POINT('Ctrl Pts',(2.96639254265844,0.891200000000001,0.262319630540593));
#16110=CARTESIAN_POINT('Ctrl Pts',(2.92780415844446,-0.208000000000001,
0.444963858672424));
#16111=CARTESIAN_POINT('Ctrl Pts',(2.92780415844446,0.891200000000001,0.444963858672424));
#16112=CARTESIAN_POINT('Ctrl Pts',(2.90717911786689,-0.208000000000001,
0.65402023086958));
#16113=CARTESIAN_POINT('Ctrl Pts',(2.90717911786689,0.891200000000001,0.65402023086958));
#16114=CARTESIAN_POINT('Ctrl Pts',(2.89547076625581,-0.208000000000001,
0.875890304828918));
#16115=CARTESIAN_POINT('Ctrl Pts',(2.89547076625581,0.891200000000001,0.875890304828918));
#16116=CARTESIAN_POINT('Ctrl Pts',(2.88537704766906,-0.208000000000001,
1.10060381648398));
#16117=CARTESIAN_POINT('Ctrl Pts',(2.88537704766906,0.891200000000001,1.10060381648398));
#16118=CARTESIAN_POINT('Ctrl Pts',(2.8728456296504,-0.208000000000001,1.32371934078733));
#16119=CARTESIAN_POINT('Ctrl Pts',(2.8728456296504,0.891200000000001,1.32371934078733));
#16120=CARTESIAN_POINT('Ctrl Pts',(2.85578261679345,-0.208000000000001,
1.54401727992264));
#16121=CARTESIAN_POINT('Ctrl Pts',(2.85578261679345,0.891200000000001,1.54401727992264));
#16122=CARTESIAN_POINT('Ctrl Pts',(2.83335686249019,-0.208000000000001,
1.76209503442146));
#16123=CARTESIAN_POINT('Ctrl Pts',(2.83335686249019,0.891200000000001,1.76209503442146));
#16124=CARTESIAN_POINT('Ctrl Pts',(2.80505146480345,-0.208000000000001,
1.97856787413951));
#16125=CARTESIAN_POINT('Ctrl Pts',(2.80505146480345,0.891200000000001,1.97856787413951));
#16126=CARTESIAN_POINT('Ctrl Pts',(2.76985908233915,-0.208000000000001,
2.19251877196071));
#16127=CARTESIAN_POINT('Ctrl Pts',(2.76985908233915,0.891200000000001,2.19251877196071));
#16128=CARTESIAN_POINT('Ctrl Pts',(2.72531955636536,-0.208000000000001,
2.39962532458029));
#16129=CARTESIAN_POINT('Ctrl Pts',(2.72531955636536,0.891200000000001,2.39962532458029));
#16130=CARTESIAN_POINT('Ctrl Pts',(2.66797634363184,-0.208000000000001,
2.59347738935741));
#16131=CARTESIAN_POINT('Ctrl Pts',(2.66797634363184,0.891200000000001,2.59347738935741));
#16132=CARTESIAN_POINT('Ctrl Pts',(2.59397540849171,-0.208000000000001,
2.7672283971178));
#16133=CARTESIAN_POINT('Ctrl Pts',(2.59397540849171,0.891200000000001,2.7672283971178));
#16134=CARTESIAN_POINT('Ctrl Pts',(2.49960870420485,-0.208000000000001,
2.91510580081997));
#16135=CARTESIAN_POINT('Ctrl Pts',(2.49960870420485,0.891200000000001,2.91510580081997));
#16136=CARTESIAN_POINT('Ctrl Pts',(2.38189256086504,-0.208000000000001,
3.03403241435618));
#16137=CARTESIAN_POINT('Ctrl Pts',(2.38189256086504,0.891200000000001,3.03403241435618));
#16138=CARTESIAN_POINT('Ctrl Pts',(2.23909845280558,-0.208000000000001,
3.12505646843308));
#16139=CARTESIAN_POINT('Ctrl Pts',(2.23909845280558,0.891200000000001,3.12505646843308));
#16140=CARTESIAN_POINT('Ctrl Pts',(2.07061055216582,-0.208000000000001,
3.19196918412265));
#16141=CARTESIAN_POINT('Ctrl Pts',(2.07061055216582,0.891200000000001,3.19196918412265));
#16142=CARTESIAN_POINT('Ctrl Pts',(1.87681490437036,-0.208000000000001,
3.24001322621211));
#16143=CARTESIAN_POINT('Ctrl Pts',(1.87681490437036,0.891200000000001,3.24001322621211));
#16144=CARTESIAN_POINT('Ctrl Pts',(1.65897747541321,-0.208000000000001,
3.27464765209773));
#16145=CARTESIAN_POINT('Ctrl Pts',(1.65897747541321,0.891200000000001,3.27464765209773));
#16146=CARTESIAN_POINT('Ctrl Pts',(1.4191255439272,-0.208000000000001,3.30006519349576));
#16147=CARTESIAN_POINT('Ctrl Pts',(1.4191255439272,0.891200000000001,3.30006519349576));
#16148=CARTESIAN_POINT('Ctrl Pts',(1.15993538533448,-0.208000000000001,
3.31897283641381));
#16149=CARTESIAN_POINT('Ctrl Pts',(1.15993538533448,0.891200000000001,3.31897283641381));
#16150=CARTESIAN_POINT('Ctrl Pts',(0.884625090385968,-0.208000000000001,
3.33300441174764));
#16151=CARTESIAN_POINT('Ctrl Pts',(0.884625090385968,0.891200000000001,
3.33300441174764));
#16152=CARTESIAN_POINT('Ctrl Pts',(0.596845720618978,-0.208000000000001,
3.34293392264922));
#16153=CARTESIAN_POINT('Ctrl Pts',(0.596845720618978,0.891200000000001,
3.34293392264922));
#16154=CARTESIAN_POINT('Ctrl Pts',(0.30057321210183,-0.208000000000001,
3.34897162637417));
#16155=CARTESIAN_POINT('Ctrl Pts',(0.30057321210183,0.891200000000001,3.34897162637417));
#16156=CARTESIAN_POINT('Ctrl Pts',(1.66741620510891E-14,-0.208000000000001,
3.35102435732185));
#16157=CARTESIAN_POINT('Ctrl Pts',(1.66741620510891E-14,0.891200000000001,
3.35102435732185));
#16158=CARTESIAN_POINT('Ctrl Pts',(-0.300573212101791,-0.208000000000001,
3.34897162637426));
#16159=CARTESIAN_POINT('Ctrl Pts',(-0.300573212101791,0.891200000000001,
3.34897162637426));
#16160=CARTESIAN_POINT('Ctrl Pts',(-0.596845720618908,-0.208000000000001,
3.34293392264938));
#16161=CARTESIAN_POINT('Ctrl Pts',(-0.596845720618908,0.891200000000001,
3.34293392264938));
#16162=CARTESIAN_POINT('Ctrl Pts',(-0.884625090385886,-0.208000000000001,
3.33300441174785));
#16163=CARTESIAN_POINT('Ctrl Pts',(-0.884625090385886,0.891200000000001,
3.33300441174785));
#16164=CARTESIAN_POINT('Ctrl Pts',(-1.15993538533442,-0.208000000000001,
3.31897283641402));
#16165=CARTESIAN_POINT('Ctrl Pts',(-1.15993538533442,0.891200000000001,
3.31897283641402));
#16166=CARTESIAN_POINT('Ctrl Pts',(-1.41912554392716,-0.208000000000001,
3.30006519349591));
#16167=CARTESIAN_POINT('Ctrl Pts',(-1.41912554392716,0.891200000000001,
3.30006519349591));
#16168=CARTESIAN_POINT('Ctrl Pts',(-1.65897747541319,-0.208000000000001,
3.27464765209779));
#16169=CARTESIAN_POINT('Ctrl Pts',(-1.65897747541319,0.891200000000001,
3.27464765209779));
#16170=CARTESIAN_POINT('Ctrl Pts',(-1.87681490437034,-0.208000000000001,
3.24001322621208));
#16171=CARTESIAN_POINT('Ctrl Pts',(-1.87681490437034,0.891200000000001,
3.24001322621208));
#16172=CARTESIAN_POINT('Ctrl Pts',(-2.07061055216576,-0.208000000000001,
3.19196918412254));
#16173=CARTESIAN_POINT('Ctrl Pts',(-2.07061055216576,0.891200000000001,
3.19196918412254));
#16174=CARTESIAN_POINT('Ctrl Pts',(-2.23909845280547,-0.208000000000001,
3.12505646843295));
#16175=CARTESIAN_POINT('Ctrl Pts',(-2.23909845280547,0.891200000000001,
3.12505646843295));
#16176=CARTESIAN_POINT('Ctrl Pts',(-2.38189256086493,-0.208000000000001,
3.03403241435609));
#16177=CARTESIAN_POINT('Ctrl Pts',(-2.38189256086493,0.891200000000001,
3.03403241435609));
#16178=CARTESIAN_POINT('Ctrl Pts',(-2.49960870420481,-0.208000000000001,
2.91510580081997));
#16179=CARTESIAN_POINT('Ctrl Pts',(-2.49960870420481,0.891200000000001,
2.91510580081997));
#16180=CARTESIAN_POINT('Ctrl Pts',(-2.59397540849182,-0.208000000000001,
2.76722839711793));
#16181=CARTESIAN_POINT('Ctrl Pts',(-2.59397540849182,0.891200000000001,
2.76722839711793));
#16182=CARTESIAN_POINT('Ctrl Pts',(-2.66797634363209,-0.208000000000001,
2.59347738935767));
#16183=CARTESIAN_POINT('Ctrl Pts',(-2.66797634363209,0.891200000000001,
2.59347738935767));
#16184=CARTESIAN_POINT('Ctrl Pts',(-2.72531955636566,-0.208000000000001,
2.39962532458057));
#16185=CARTESIAN_POINT('Ctrl Pts',(-2.72531955636566,0.891200000000001,
2.39962532458057));
#16186=CARTESIAN_POINT('Ctrl Pts',(-2.76985908233936,-0.208000000000001,
2.19251877196088));
#16187=CARTESIAN_POINT('Ctrl Pts',(-2.76985908233936,0.891200000000001,
2.19251877196088));
#16188=CARTESIAN_POINT('Ctrl Pts',(-2.80505146480344,-0.208000000000001,
1.97856787413951));
#16189=CARTESIAN_POINT('Ctrl Pts',(-2.80505146480344,0.891200000000001,
1.97856787413951));
#16190=CARTESIAN_POINT('Ctrl Pts',(-2.8333568624899,-0.208000000000001,
1.76209503442131));
#16191=CARTESIAN_POINT('Ctrl Pts',(-2.8333568624899,0.891200000000001,1.76209503442131));
#16192=CARTESIAN_POINT('Ctrl Pts',(-2.85578261679294,-0.208000000000001,
1.54401727992238));
#16193=CARTESIAN_POINT('Ctrl Pts',(-2.85578261679294,0.891200000000001,
1.54401727992238));
#16194=CARTESIAN_POINT('Ctrl Pts',(-2.87284562964987,-0.208000000000001,
1.32371934078708));
#16195=CARTESIAN_POINT('Ctrl Pts',(-2.87284562964987,0.891200000000001,
1.32371934078708));
#16196=CARTESIAN_POINT('Ctrl Pts',(-2.88537704766869,-0.208000000000001,
1.10060381648384));
#16197=CARTESIAN_POINT('Ctrl Pts',(-2.88537704766869,0.891200000000001,
1.10060381648384));
#16198=CARTESIAN_POINT('Ctrl Pts',(-2.89547076625573,-0.208000000000001,
0.875890304828914));
#16199=CARTESIAN_POINT('Ctrl Pts',(-2.89547076625573,0.891200000000001,
0.875890304828914));
#16200=CARTESIAN_POINT('Ctrl Pts',(-2.90717911786707,-0.208000000000001,
0.654020230869684));
#16201=CARTESIAN_POINT('Ctrl Pts',(-2.90717911786707,0.891200000000001,
0.654020230869684));
#16202=CARTESIAN_POINT('Ctrl Pts',(-2.92780415844476,-0.208000000000001,
0.444963858672577));
#16203=CARTESIAN_POINT('Ctrl Pts',(-2.92780415844476,0.891200000000001,
0.444963858672577));
#16204=CARTESIAN_POINT('Ctrl Pts',(-2.96639254265869,-0.208000000000001,
0.262319630540737));
#16205=CARTESIAN_POINT('Ctrl Pts',(-2.96639254265869,0.891200000000001,
0.262319630540737));
#16206=CARTESIAN_POINT('Ctrl Pts',(-3.03063129752067,-0.208000000000001,
0.11901737132707));
#16207=CARTESIAN_POINT('Ctrl Pts',(-3.03063129752067,0.891200000000001,
0.11901737132707));
#16208=CARTESIAN_POINT('Ctrl Pts',(-3.12452733970658,-0.208000000000001,
0.0241851999813871));
#16209=CARTESIAN_POINT('Ctrl Pts',(-3.12452733970658,0.891200000000001,
0.0241851999813871));
#16210=CARTESIAN_POINT('Ctrl Pts',(-3.24511001026157,-0.208000000000001,
-0.0214179570895714));
#16211=CARTESIAN_POINT('Ctrl Pts',(-3.24511001026157,0.891200000000001,
-0.0214179570895714));
#16212=CARTESIAN_POINT('Ctrl Pts',(-3.38164698943802,-0.208000000000001,
-0.0263068037112043));
#16213=CARTESIAN_POINT('Ctrl Pts',(-3.38164698943802,0.891200000000001,
-0.0263068037112043));
#16214=CARTESIAN_POINT('Ctrl Pts',(-3.52045328348989,-0.208000000000001,
-0.00118366394785932));
#16215=CARTESIAN_POINT('Ctrl Pts',(-3.52045328348989,0.891200000000001,
-0.00118366394785932));
#16216=CARTESIAN_POINT('Ctrl Pts',(-3.64881642260079,-0.208000000000001,
0.0470540298718583));
#16217=CARTESIAN_POINT('Ctrl Pts',(-3.64881642260079,0.891200000000001,
0.0470540298718583));
#16218=CARTESIAN_POINT('Ctrl Pts',(-3.75872318140663,-0.208000000000001,
0.120497232333251));
#16219=CARTESIAN_POINT('Ctrl Pts',(-3.75872318140663,0.891200000000001,
0.120497232333251));
#16220=CARTESIAN_POINT('Ctrl Pts',(-3.84598208672296,-0.208000000000001,
0.224659532804408));
#16221=CARTESIAN_POINT('Ctrl Pts',(-3.84598208672296,0.891200000000001,
0.224659532804408));
#16222=CARTESIAN_POINT('Ctrl Pts',(-3.9098657241983,-0.208000000000001,
0.364350357241515));
#16223=CARTESIAN_POINT('Ctrl Pts',(-3.9098657241983,0.891200000000001,0.364350357241515));
#16224=CARTESIAN_POINT('Ctrl Pts',(-3.9525920016999,-0.208000000000001,
0.538436816836325));
#16225=CARTESIAN_POINT('Ctrl Pts',(-3.9525920016999,0.891200000000001,0.538436816836325));
#16226=CARTESIAN_POINT('Ctrl Pts',(-3.97841403016126,-0.208000000000001,
0.741129277895169));
#16227=CARTESIAN_POINT('Ctrl Pts',(-3.97841403016126,0.891200000000001,
0.741129277895169));
#16228=CARTESIAN_POINT('Ctrl Pts',(-3.99260375067011,-0.208000000000001,
0.964078729991154));
#16229=CARTESIAN_POINT('Ctrl Pts',(-3.99260375067011,0.891200000000001,
0.964078729991154));
#16230=CARTESIAN_POINT('Ctrl Pts',(-4.00047520099045,-0.208000000000001,
1.1981954227983));
#16231=CARTESIAN_POINT('Ctrl Pts',(-4.00047520099045,0.891200000000001,
1.1981954227983));
#16232=CARTESIAN_POINT('Ctrl Pts',(-4.00639322616607,-0.208000000000001,
1.43558101932923));
#16233=CARTESIAN_POINT('Ctrl Pts',(-4.00639322616607,0.891200000000001,
1.43558101932923));
#16234=CARTESIAN_POINT('Ctrl Pts',(-4.01278239926574,-0.208000000000001,
1.67142113207667));
#16235=CARTESIAN_POINT('Ctrl Pts',(-4.01278239926574,0.891200000000001,
1.67142113207667));
#16236=CARTESIAN_POINT('Ctrl Pts',(-4.02066709528487,-0.208000000000001,
1.90332556813333));
#16237=CARTESIAN_POINT('Ctrl Pts',(-4.02066709528487,0.891200000000001,
1.90332556813333));
#16238=CARTESIAN_POINT('Ctrl Pts',(-4.0302101444685,-0.208000000000001,
2.130657485557));
#16239=CARTESIAN_POINT('Ctrl Pts',(-4.0302101444685,0.891200000000001,2.130657485557));
#16240=CARTESIAN_POINT('Ctrl Pts',(-4.04126813644779,-0.208000000000001,
2.35385258470204));
#16241=CARTESIAN_POINT('Ctrl Pts',(-4.04126813644779,0.891200000000001,
2.35385258470204));
#16242=CARTESIAN_POINT('Ctrl Pts',(-4.05390260344525,-0.208000000000001,
2.57377631141659));
#16243=CARTESIAN_POINT('Ctrl Pts',(-4.05390260344525,0.891200000000001,
2.57377631141659));
#16244=CARTESIAN_POINT('Ctrl Pts',(-4.06899962712502,-0.208000000000001,
2.7909834104825));
#16245=CARTESIAN_POINT('Ctrl Pts',(-4.06899962712502,0.891200000000001,
2.7909834104825));
#16246=CARTESIAN_POINT('Ctrl Pts',(-4.08854433447739,-0.208000000000001,
3.00529120729338));
#16247=CARTESIAN_POINT('Ctrl Pts',(-4.08854433447739,0.891200000000001,
3.00529120729338));
#16248=CARTESIAN_POINT('Ctrl Pts',(-4.11518318246524,-0.208000000000001,
3.21600287470921));
#16249=CARTESIAN_POINT('Ctrl Pts',(-4.11518318246524,0.891200000000001,
3.21600287470921));
#16250=CARTESIAN_POINT('Ctrl Pts',(-4.15193466045748,-0.208000000000001,
3.42199345348447));
#16251=CARTESIAN_POINT('Ctrl Pts',(-4.15193466045748,0.891200000000001,
3.42199345348447));
#16252=CARTESIAN_POINT('Ctrl Pts',(-4.20184334854115,-0.208000000000001,
3.62185203209171));
#16253=CARTESIAN_POINT('Ctrl Pts',(-4.20184334854115,0.891200000000001,
3.62185203209171));
#16254=CARTESIAN_POINT('Ctrl Pts',(-4.26765207024395,-0.208000000000001,
3.81399668859083));
#16255=CARTESIAN_POINT('Ctrl Pts',(-4.26765207024395,0.891200000000001,
3.81399668859083));
#16256=CARTESIAN_POINT('Ctrl Pts',(-4.35148411330718,-0.208000000000001,
3.99681013615577));
#16257=CARTESIAN_POINT('Ctrl Pts',(-4.35148411330718,0.891200000000001,
3.99681013615577));
#16258=CARTESIAN_POINT('Ctrl Pts',(-4.45474519640294,-0.208000000000001,
4.16885849319142));
#16259=CARTESIAN_POINT('Ctrl Pts',(-4.45474519640294,0.891200000000001,
4.16885849319142));
#16260=CARTESIAN_POINT('Ctrl Pts',(-4.57800047823775,-0.208000000000001,
4.32911151507774));
#16261=CARTESIAN_POINT('Ctrl Pts',(-4.57800047823775,0.891200000000001,
4.32911151507774));
#16262=CARTESIAN_POINT('Ctrl Pts',(-4.7208720035032,-0.208000000000001,
4.47714872481861));
#16263=CARTESIAN_POINT('Ctrl Pts',(-4.7208720035032,0.891200000000001,4.47714872481861));
#16264=CARTESIAN_POINT('Ctrl Pts',(-4.88190185104852,-0.208000000000001,
4.61340315498244));
#16265=CARTESIAN_POINT('Ctrl Pts',(-4.88190185104852,0.891200000000001,
4.61340315498244));
#16266=CARTESIAN_POINT('Ctrl Pts',(-5.05850630701885,-0.208000000000001,
4.73929437247796));
#16267=CARTESIAN_POINT('Ctrl Pts',(-5.05850630701885,0.891200000000001,
4.73929437247796));
#16268=CARTESIAN_POINT('Ctrl Pts',(-5.24741086000019,-0.208000000000001,
4.8567611153285));
#16269=CARTESIAN_POINT('Ctrl Pts',(-5.24741086000019,0.891200000000001,
4.8567611153285));
#16270=CARTESIAN_POINT('Ctrl Pts',(-5.44501860313342,-0.208000000000001,
4.96787993373728));
#16271=CARTESIAN_POINT('Ctrl Pts',(-5.44501860313342,0.891200000000001,
4.96787993373728));
#16272=CARTESIAN_POINT('Ctrl Pts',(-5.64781737380319,-0.208000000000001,
5.07442896098937));
#16273=CARTESIAN_POINT('Ctrl Pts',(-5.64781737380319,0.891200000000001,
5.07442896098937));
#16274=CARTESIAN_POINT('Ctrl Pts',(-5.85274048349242,-0.208000000000001,
5.17752467829109));
#16275=CARTESIAN_POINT('Ctrl Pts',(-5.85274048349242,0.891200000000001,
5.17752467829109));
#16276=CARTESIAN_POINT('Ctrl Pts',(-6.05762450882858,-0.208000000000001,
5.27709955371564));
#16277=CARTESIAN_POINT('Ctrl Pts',(-6.05762450882858,0.891200000000001,
5.27709955371564));
#16278=CARTESIAN_POINT('Ctrl Pts',(-6.26112587698772,-0.208000000000001,
5.37226655127787));
#16279=CARTESIAN_POINT('Ctrl Pts',(-6.26112587698772,0.891200000000001,
5.37226655127787));
#16280=CARTESIAN_POINT('Ctrl Pts',(-6.46246210121964,-0.208000000000001,
5.46195513100446));
#16281=CARTESIAN_POINT('Ctrl Pts',(-6.46246210121964,0.891200000000001,
5.46195513100446));
#16282=CARTESIAN_POINT('Ctrl Pts',(-6.66121503090592,-0.208000000000001,
5.54547963906637));
#16283=CARTESIAN_POINT('Ctrl Pts',(-6.66121503090592,0.891200000000001,
5.54547963906637));
#16284=CARTESIAN_POINT('Ctrl Pts',(-6.8570997603751,-0.208000000000001,
5.62308582598972));
#16285=CARTESIAN_POINT('Ctrl Pts',(-6.8570997603751,0.891200000000001,5.62308582598972));
#16286=CARTESIAN_POINT('Ctrl Pts',(-7.04976847947249,-0.208000000000001,
5.69662713609756));
#16287=CARTESIAN_POINT('Ctrl Pts',(-7.04976847947249,0.891200000000001,
5.69662713609756));
#16288=CARTESIAN_POINT('Ctrl Pts',(-7.23853768475,-0.208000000000001,5.76979878895672));
#16289=CARTESIAN_POINT('Ctrl Pts',(-7.23853768475,0.891200000000001,5.76979878895672));
#16290=CARTESIAN_POINT('Ctrl Pts',(-7.42198551710617,-0.208000000000001,
5.84723737025949));
#16291=CARTESIAN_POINT('Ctrl Pts',(-7.42198551710617,0.891200000000001,
5.84723737025949));
#16292=CARTESIAN_POINT('Ctrl Pts',(-7.59751903688412,-0.208000000000001,
5.93381436957244));
#16293=CARTESIAN_POINT('Ctrl Pts',(-7.59751903688412,0.891200000000001,
5.93381436957244));
#16294=CARTESIAN_POINT('Ctrl Pts',(-7.76106756457753,-0.208000000000001,
6.03389995867283));
#16295=CARTESIAN_POINT('Ctrl Pts',(-7.76106756457753,0.891200000000001,
6.03389995867283));
#16296=CARTESIAN_POINT('Ctrl Pts',(-7.90644860448901,-0.208000000000001,
6.15052660592937));
#16297=CARTESIAN_POINT('Ctrl Pts',(-7.90644860448901,0.891200000000001,
6.15052660592937));
#16298=CARTESIAN_POINT('Ctrl Pts',(-8.02580908828117,-0.208000000000001,
6.28498018271686));
#16299=CARTESIAN_POINT('Ctrl Pts',(-8.02580908828117,0.891200000000001,
6.28498018271686));
#16300=CARTESIAN_POINT('Ctrl Pts',(-8.11207116917861,-0.208000000000001,
6.43720976255636));
#16301=CARTESIAN_POINT('Ctrl Pts',(-8.11207116917861,0.891200000000001,
6.43720976255636));
#16302=CARTESIAN_POINT('Ctrl Pts',(-8.16089752265956,-0.208000000000001,
6.60605451948903));
#16303=CARTESIAN_POINT('Ctrl Pts',(-8.16089752265956,0.891200000000001,
6.60605451948903));
#16304=CARTESIAN_POINT('Ctrl Pts',(-8.17293082304181,-0.208000000000001,
6.78954489191904));
#16305=CARTESIAN_POINT('Ctrl Pts',(-8.17293082304181,0.891200000000001,
6.78954489191904));
#16306=CARTESIAN_POINT('Ctrl Pts',(-8.15569042861244,-0.208000000000001,
6.9851692342788));
#16307=CARTESIAN_POINT('Ctrl Pts',(-8.15569042861244,0.891200000000001,
6.9851692342788));
#16308=CARTESIAN_POINT('Ctrl Pts',(-8.12057943633387,-0.208000000000001,
7.19009032473164));
#16309=CARTESIAN_POINT('Ctrl Pts',(-8.12057943633387,0.891200000000001,
7.19009032473164));
#16310=CARTESIAN_POINT('Ctrl Pts',(-8.08008348678073,-0.208000000000001,
7.40136016279791));
#16311=CARTESIAN_POINT('Ctrl Pts',(-8.08008348678073,0.891200000000001,
7.40136016279791));
#16312=CARTESIAN_POINT('Ctrl Pts',(-8.04494633492831,-0.208000000000001,
7.61613341658677));
#16313=CARTESIAN_POINT('Ctrl Pts',(-8.04494633492831,0.891200000000001,
7.61613341658677));
#16314=CARTESIAN_POINT('Ctrl Pts',(-8.02124364536279,-0.208000000000001,
7.83188673232793));
#16315=CARTESIAN_POINT('Ctrl Pts',(-8.02124364536279,0.891200000000001,
7.83188673232793));
#16316=CARTESIAN_POINT('Ctrl Pts',(-8.007818938056,-0.208000000000001,8.04662057355248));
#16317=CARTESIAN_POINT('Ctrl Pts',(-8.007818938056,0.891200000000001,8.04662057355248));
#16318=CARTESIAN_POINT('Ctrl Pts',(-7.99879843919661,-0.208000000000001,
8.25883677791483));
#16319=CARTESIAN_POINT('Ctrl Pts',(-7.99879843919661,0.891200000000001,
8.25883677791483));
#16320=CARTESIAN_POINT('Ctrl Pts',(-7.98575825096101,-0.208000000000001,
8.46752658699528));
#16321=CARTESIAN_POINT('Ctrl Pts',(-7.98575825096101,0.891200000000001,
8.46752658699528));
#16322=CARTESIAN_POINT('Ctrl Pts',(-7.96007609558389,-0.208000000000001,
8.67216210283896));
#16323=CARTESIAN_POINT('Ctrl Pts',(-7.96007609558389,0.891200000000001,
8.67216210283896));
#16324=CARTESIAN_POINT('Ctrl Pts',(-7.91508259073019,-0.208000000000001,
8.87266947141823));
#16325=CARTESIAN_POINT('Ctrl Pts',(-7.91508259073019,0.891200000000001,
8.87266947141823));
#16326=CARTESIAN_POINT('Ctrl Pts',(-7.84862074946261,-0.208000000000001,
9.06945407016992));
#16327=CARTESIAN_POINT('Ctrl Pts',(-7.84862074946261,0.891200000000001,
9.06945407016992));
#16328=CARTESIAN_POINT('Ctrl Pts',(-7.76209282457479,-0.208000000000001,
9.26297089919765));
#16329=CARTESIAN_POINT('Ctrl Pts',(-7.76209282457479,0.891200000000001,
9.26297089919765));
#16330=CARTESIAN_POINT('Ctrl Pts',(-7.65900038660722,-0.208000000000001,
9.4532499945042));
#16331=CARTESIAN_POINT('Ctrl Pts',(-7.65900038660722,0.891200000000001,
9.4532499945042));
#16332=CARTESIAN_POINT('Ctrl Pts',(-7.5436057352653,-0.208000000000001,
9.63939026966035));
#16333=CARTESIAN_POINT('Ctrl Pts',(-7.5436057352653,0.891200000000001,9.63939026966035));
#16334=CARTESIAN_POINT('Ctrl Pts',(-7.41967047355001,-0.208000000000001,
9.81917361987397));
#16335=CARTESIAN_POINT('Ctrl Pts',(-7.41967047355001,0.891200000000001,
9.81917361987397));
#16336=CARTESIAN_POINT('Ctrl Pts',(-7.28883796912703,-0.208000000000001,
9.98835756998572));
#16337=CARTESIAN_POINT('Ctrl Pts',(-7.28883796912703,0.891200000000001,
9.98835756998572));
#16338=CARTESIAN_POINT('Ctrl Pts',(-7.15081550722306,-0.208000000000001,
10.1414720974148));
#16339=CARTESIAN_POINT('Ctrl Pts',(-7.15081550722306,0.891200000000001,
10.1414720974148));
#16340=CARTESIAN_POINT('Ctrl Pts',(-7.0044544864105,-0.208000000000001,
10.2733319413008));
#16341=CARTESIAN_POINT('Ctrl Pts',(-7.0044544864105,0.891200000000001,10.2733319413008));
#16342=CARTESIAN_POINT('Ctrl Pts',(-6.84859008776113,-0.208000000000001,
10.3804015453596));
#16343=CARTESIAN_POINT('Ctrl Pts',(-6.84859008776113,0.891200000000001,
10.3804015453596));
#16344=CARTESIAN_POINT('Ctrl Pts',(-6.68288828293938,-0.208000000000001,
10.4620502678778));
#16345=CARTESIAN_POINT('Ctrl Pts',(-6.68288828293938,0.891200000000001,
10.4620502678778));
#16346=CARTESIAN_POINT('Ctrl Pts',(-6.50892555577766,-0.208000000000001,
10.522290883026));
#16347=CARTESIAN_POINT('Ctrl Pts',(-6.50892555577766,0.891200000000001,
10.522290883026));
#16348=CARTESIAN_POINT('Ctrl Pts',(-6.32976796473811,-0.208000000000001,
10.5687216653902));
#16349=CARTESIAN_POINT('Ctrl Pts',(-6.32976796473811,0.891200000000001,
10.5687216653902));
#16350=CARTESIAN_POINT('Ctrl Pts',(-6.14893768388701,-0.208000000000001,
10.6103475969885));
#16351=CARTESIAN_POINT('Ctrl Pts',(-6.14893768388701,0.891200000000001,
10.6103475969885));
#16352=CARTESIAN_POINT('Ctrl Pts',(-5.96961932707142,-0.208000000000001,
10.6558377434043));
#16353=CARTESIAN_POINT('Ctrl Pts',(-5.96961932707142,0.891200000000001,
10.6558377434043));
#16354=CARTESIAN_POINT('Ctrl Pts',(-5.79367695415031,-0.208000000000001,
10.7114411549114));
#16355=CARTESIAN_POINT('Ctrl Pts',(-5.79367695415031,0.891200000000001,
10.7114411549114));
#16356=CARTESIAN_POINT('Ctrl Pts',(-5.62101499943431,-0.208000000000001,
10.7795199127535));
#16357=CARTESIAN_POINT('Ctrl Pts',(-5.62101499943431,0.891200000000001,
10.7795199127535));
#16358=CARTESIAN_POINT('Ctrl Pts',(-5.45051506148982,-0.208000000000001,
10.8599381259737));
#16359=CARTESIAN_POINT('Ctrl Pts',(-5.45051506148982,0.891200000000001,
10.8599381259737));
#16360=CARTESIAN_POINT('Ctrl Pts',(-5.28082876351929,-0.208000000000001,
10.9511663773826));
#16361=CARTESIAN_POINT('Ctrl Pts',(-5.28082876351929,0.891200000000001,
10.9511663773826));
#16362=CARTESIAN_POINT('Ctrl Pts',(-5.11112998264616,-0.208000000000001,
11.0513704191329));
#16363=CARTESIAN_POINT('Ctrl Pts',(-5.11112998264616,0.891200000000001,
11.0513704191329));
#16364=CARTESIAN_POINT('Ctrl Pts',(-4.94211773226973,-0.208000000000001,
11.1598106424589));
#16365=CARTESIAN_POINT('Ctrl Pts',(-4.94211773226973,0.891200000000001,
11.1598106424589));
#16366=CARTESIAN_POINT('Ctrl Pts',(-4.77596612414951,-0.208000000000001,
11.2768795166235));
#16367=CARTESIAN_POINT('Ctrl Pts',(-4.77596612414951,0.891200000000001,
11.2768795166235));
#16368=CARTESIAN_POINT('Ctrl Pts',(-4.61532593596946,-0.208000000000001,
11.4029224160731));
#16369=CARTESIAN_POINT('Ctrl Pts',(-4.61532593596946,0.891200000000001,
11.4029224160731));
#16370=CARTESIAN_POINT('Ctrl Pts',(-4.46255574628757,-0.208000000000001,
11.5373242211527));
#16371=CARTESIAN_POINT('Ctrl Pts',(-4.46255574628757,0.891200000000001,
11.5373242211527));
#16372=CARTESIAN_POINT('Ctrl Pts',(-4.31893584999241,-0.208000000000001,
11.6776492463597));
#16373=CARTESIAN_POINT('Ctrl Pts',(-4.31893584999241,0.891200000000001,
11.6776492463597));
#16374=CARTESIAN_POINT('Ctrl Pts',(-4.18369962429796,-0.208000000000001,
11.8183570873721));
#16375=CARTESIAN_POINT('Ctrl Pts',(-4.18369962429796,0.891200000000001,
11.8183570873721));
#16376=CARTESIAN_POINT('Ctrl Pts',(-4.05395481372655,-0.208000000000001,
11.9514202619522));
#16377=CARTESIAN_POINT('Ctrl Pts',(-4.05395481372655,0.891200000000001,
11.9514202619522));
#16378=CARTESIAN_POINT('Ctrl Pts',(-3.92533033057354,-0.208000000000001,
12.0684942936867));
#16379=CARTESIAN_POINT('Ctrl Pts',(-3.92533033057354,0.891200000000001,
12.0684942936867));
#16380=CARTESIAN_POINT('Ctrl Pts',(-3.79241297762166,-0.208000000000001,
12.1626050652586));
#16381=CARTESIAN_POINT('Ctrl Pts',(-3.79241297762166,0.891200000000001,
12.1626050652586));
#16382=CARTESIAN_POINT('Ctrl Pts',(-3.64927048315908,-0.208000000000001,
12.2301117722809));
#16383=CARTESIAN_POINT('Ctrl Pts',(-3.64927048315908,0.891200000000001,
12.2301117722809));
#16384=CARTESIAN_POINT('Ctrl Pts',(-3.48993681214334,-0.208000000000001,
12.2723364229645));
#16385=CARTESIAN_POINT('Ctrl Pts',(-3.48993681214334,0.891200000000001,
12.2723364229645));
#16386=CARTESIAN_POINT('Ctrl Pts',(-3.30884480305534,-0.208000000000001,
12.2938762651139));
#16387=CARTESIAN_POINT('Ctrl Pts',(-3.30884480305534,0.891200000000001,
12.2938762651139));
#16388=CARTESIAN_POINT('Ctrl Pts',(-3.10127560868576,-0.208000000000001,
12.3010487961981));
#16389=CARTESIAN_POINT('Ctrl Pts',(-3.10127560868576,0.891200000000001,
12.3010487961981));
#16390=CARTESIAN_POINT('Ctrl Pts',(-2.86376302967345,-0.208000000000001,
12.300400839059));
#16391=CARTESIAN_POINT('Ctrl Pts',(-2.86376302967345,0.891200000000001,
12.300400839059));
#16392=CARTESIAN_POINT('Ctrl Pts',(-2.59461297443094,-0.208000000000001,
12.2969132923574));
#16393=CARTESIAN_POINT('Ctrl Pts',(-2.59461297443094,0.891200000000001,
12.2969132923574));
#16394=CARTESIAN_POINT('Ctrl Pts',(-2.29394197380209,-0.208000000000001,
12.2935845551224));
#16395=CARTESIAN_POINT('Ctrl Pts',(-2.29394197380209,0.891200000000001,
12.2935845551224));
#16396=CARTESIAN_POINT('Ctrl Pts',(-1.96338745719135,-0.208000000000001,
12.2919684497906));
#16397=CARTESIAN_POINT('Ctrl Pts',(-1.96338745719135,0.891200000000001,
12.2919684497906));
#16398=CARTESIAN_POINT('Ctrl Pts',(-1.60591558979456,-0.208000000000001,
12.2924280531798));
#16399=CARTESIAN_POINT('Ctrl Pts',(-1.60591558979456,0.891200000000001,
12.2924280531798));
#16400=CARTESIAN_POINT('Ctrl Pts',(-1.22558901314075,-0.208000000000001,
12.2945066442122));
#16401=CARTESIAN_POINT('Ctrl Pts',(-1.22558901314075,0.891200000000001,
12.2945066442122));
#16402=CARTESIAN_POINT('Ctrl Pts',(-0.827351903312651,-0.208000000000001,
12.2972483292773));
#16403=CARTESIAN_POINT('Ctrl Pts',(-0.827351903312651,0.891200000000001,
12.2972483292773));
#16404=CARTESIAN_POINT('Ctrl Pts',(-0.498916532526571,-0.208000000000001,
12.299081889758));
#16405=CARTESIAN_POINT('Ctrl Pts',(-0.498916532526571,0.891200000000001,
12.299081889758));
#16406=CARTESIAN_POINT('Ctrl Pts',(-0.249771440080693,-0.208000000000001,
12.2998330708668));
#16407=CARTESIAN_POINT('Ctrl Pts',(-0.249771440080693,0.891200000000001,
12.2998330708668));
#16408=CARTESIAN_POINT('Ctrl Pts',(-0.0832571466935557,-0.208000000000001,
12.2999999999989));
#16409=CARTESIAN_POINT('Ctrl Pts',(-0.0832571466935557,0.891200000000001,
12.2999999999989));
#16410=CARTESIAN_POINT('Ctrl Pts',(0.,-0.208000000000001,12.3));
#16411=CARTESIAN_POINT('Ctrl Pts',(0.,0.891200000000001,12.3));
#16412=CARTESIAN_POINT('Ctrl Pts',(0.0832571466935396,-0.208000000000001,
12.3000000000011));
#16413=CARTESIAN_POINT('Ctrl Pts',(0.0832571466935396,0.891200000000001,
12.3000000000011));
#16414=CARTESIAN_POINT('Ctrl Pts',(0.24977144008061,-0.208000000000001,
12.2998330708736));
#16415=CARTESIAN_POINT('Ctrl Pts',(0.24977144008061,0.891200000000001,12.2998330708736));
#16416=CARTESIAN_POINT('Ctrl Pts',(0.498916532526534,-0.208000000000001,
12.2990818897713));
#16417=CARTESIAN_POINT('Ctrl Pts',(0.498916532526534,0.891200000000001,
12.2990818897713));
#16418=CARTESIAN_POINT('Ctrl Pts',(0.827351903312438,-0.208000000000001,
12.2972483292974));
#16419=CARTESIAN_POINT('Ctrl Pts',(0.827351903312438,0.891200000000001,
12.2972483292974));
#16420=CARTESIAN_POINT('Ctrl Pts',(1.22558901314046,-0.208000000000001,
12.2945066442369));
#16421=CARTESIAN_POINT('Ctrl Pts',(1.22558901314046,0.891200000000001,12.2945066442369));
#16422=CARTESIAN_POINT('Ctrl Pts',(1.60591558979418,-0.208000000000001,
12.2924280532047));
#16423=CARTESIAN_POINT('Ctrl Pts',(1.60591558979418,0.891200000000001,12.2924280532047));
#16424=CARTESIAN_POINT('Ctrl Pts',(1.96338745719096,-0.208000000000001,
12.291968449812));
#16425=CARTESIAN_POINT('Ctrl Pts',(1.96338745719096,0.891200000000001,12.291968449812));
#16426=CARTESIAN_POINT('Ctrl Pts',(2.29394197380175,-0.208000000000001,
12.2935845551378));
#16427=CARTESIAN_POINT('Ctrl Pts',(2.29394197380175,0.891200000000001,12.2935845551378));
#16428=CARTESIAN_POINT('Ctrl Pts',(2.59461297443069,-0.208000000000001,
12.2969132923658));
#16429=CARTESIAN_POINT('Ctrl Pts',(2.59461297443069,0.891200000000001,12.2969132923658));
#16430=CARTESIAN_POINT('Ctrl Pts',(2.86376302967335,-0.208000000000001,
12.3004008390612));
#16431=CARTESIAN_POINT('Ctrl Pts',(2.86376302967335,0.891200000000001,12.3004008390612));
#16432=CARTESIAN_POINT('Ctrl Pts',(3.10127560868576,-0.208000000000001,
12.3010487961961));
#16433=CARTESIAN_POINT('Ctrl Pts',(3.10127560868576,0.891200000000001,12.3010487961961));
#16434=CARTESIAN_POINT('Ctrl Pts',(3.30884480305537,-0.208000000000001,
12.2938762651102));
#16435=CARTESIAN_POINT('Ctrl Pts',(3.30884480305537,0.891200000000001,12.2938762651102));
#16436=CARTESIAN_POINT('Ctrl Pts',(3.48993681214337,-0.208000000000001,
12.2723364229612));
#16437=CARTESIAN_POINT('Ctrl Pts',(3.48993681214337,0.891200000000001,12.2723364229612));
#16438=CARTESIAN_POINT('Ctrl Pts',(3.64927048315907,-0.208000000000001,
12.2301117722792));
#16439=CARTESIAN_POINT('Ctrl Pts',(3.64927048315907,0.891200000000001,12.2301117722792));
#16440=CARTESIAN_POINT('Ctrl Pts',(3.79241297762162,-0.208000000000001,
12.1626050652587));
#16441=CARTESIAN_POINT('Ctrl Pts',(3.79241297762162,0.891200000000001,12.1626050652587));
#16442=CARTESIAN_POINT('Ctrl Pts',(3.92533033057351,-0.208000000000001,
12.0684942936878));
#16443=CARTESIAN_POINT('Ctrl Pts',(3.92533033057351,0.891200000000001,12.0684942936878));
#16444=CARTESIAN_POINT('Ctrl Pts',(4.05395481372655,-0.208000000000001,
11.9514202619535));
#16445=CARTESIAN_POINT('Ctrl Pts',(4.05395481372655,0.891200000000001,11.9514202619535));
#16446=CARTESIAN_POINT('Ctrl Pts',(4.18369962429796,-0.208000000000001,
11.8183570873731));
#16447=CARTESIAN_POINT('Ctrl Pts',(4.18369962429796,0.891200000000001,11.8183570873731));
#16448=CARTESIAN_POINT('Ctrl Pts',(4.3189358499924,-0.208000000000001,11.67764924636));
#16449=CARTESIAN_POINT('Ctrl Pts',(4.3189358499924,0.891200000000001,11.67764924636));
#16450=CARTESIAN_POINT('Ctrl Pts',(4.46255574628753,-0.208000000000001,
11.5373242211525));
#16451=CARTESIAN_POINT('Ctrl Pts',(4.46255574628753,0.891200000000001,11.5373242211525));
#16452=CARTESIAN_POINT('Ctrl Pts',(4.61532593596939,-0.208000000000001,
11.4029224160728));
#16453=CARTESIAN_POINT('Ctrl Pts',(4.61532593596939,0.891200000000001,11.4029224160728));
#16454=CARTESIAN_POINT('Ctrl Pts',(4.77596612414944,-0.208000000000001,
11.2768795166233));
#16455=CARTESIAN_POINT('Ctrl Pts',(4.77596612414944,0.891200000000001,11.2768795166233));
#16456=CARTESIAN_POINT('Ctrl Pts',(4.94211773226968,-0.208000000000001,
11.1598106424589));
#16457=CARTESIAN_POINT('Ctrl Pts',(4.94211773226968,0.891200000000001,11.1598106424589));
#16458=CARTESIAN_POINT('Ctrl Pts',(5.11112998264613,-0.208000000000001,
11.051370419133));
#16459=CARTESIAN_POINT('Ctrl Pts',(5.11112998264613,0.891200000000001,11.051370419133));
#16460=CARTESIAN_POINT('Ctrl Pts',(5.28082876351925,-0.208000000000001,
10.9511663773825));
#16461=CARTESIAN_POINT('Ctrl Pts',(5.28082876351925,0.891200000000001,10.9511663773825));
#16462=CARTESIAN_POINT('Ctrl Pts',(5.45051506148977,-0.208000000000001,
10.8599381259735));
#16463=CARTESIAN_POINT('Ctrl Pts',(5.45051506148977,0.891200000000001,10.8599381259735));
#16464=CARTESIAN_POINT('Ctrl Pts',(5.62101499943423,-0.208000000000001,
10.7795199127532));
#16465=CARTESIAN_POINT('Ctrl Pts',(5.62101499943423,0.891200000000001,10.7795199127532));
#16466=CARTESIAN_POINT('Ctrl Pts',(5.7936769541502,-0.208000000000001,10.7114411549111));
#16467=CARTESIAN_POINT('Ctrl Pts',(5.7936769541502,0.891200000000001,10.7114411549111));
#16468=CARTESIAN_POINT('Ctrl Pts',(5.96961932707136,-0.208000000000001,
10.6558377434042));
#16469=CARTESIAN_POINT('Ctrl Pts',(5.96961932707136,0.891200000000001,10.6558377434042));
#16470=CARTESIAN_POINT('Ctrl Pts',(6.14893768388704,-0.208000000000001,
10.6103475969888));
#16471=CARTESIAN_POINT('Ctrl Pts',(6.14893768388704,0.891200000000001,10.6103475969888));
#16472=CARTESIAN_POINT('Ctrl Pts',(6.32976796473819,-0.208000000000001,
10.5687216653907));
#16473=CARTESIAN_POINT('Ctrl Pts',(6.32976796473819,0.891200000000001,10.5687216653907));
#16474=CARTESIAN_POINT('Ctrl Pts',(6.50892555577775,-0.208000000000001,
10.5222908830264));
#16475=CARTESIAN_POINT('Ctrl Pts',(6.50892555577775,0.891200000000001,10.5222908830264));
#16476=CARTESIAN_POINT('Ctrl Pts',(6.68288828293941,-0.208000000000001,
10.462050267878));
#16477=CARTESIAN_POINT('Ctrl Pts',(6.68288828293941,0.891200000000001,10.462050267878));
#16478=CARTESIAN_POINT('Ctrl Pts',(6.84859008776107,-0.208000000000001,
10.3804015453596));
#16479=CARTESIAN_POINT('Ctrl Pts',(6.84859008776107,0.891200000000001,10.3804015453596));
#16480=CARTESIAN_POINT('Ctrl Pts',(7.00445448641038,-0.208000000000001,
10.2733319413005));
#16481=CARTESIAN_POINT('Ctrl Pts',(7.00445448641038,0.891200000000001,10.2733319413005));
#16482=CARTESIAN_POINT('Ctrl Pts',(7.15081550722288,-0.208000000000001,
10.1414720974144));
#16483=CARTESIAN_POINT('Ctrl Pts',(7.15081550722288,0.891200000000001,10.1414720974144));
#16484=CARTESIAN_POINT('Ctrl Pts',(7.28883796912684,-0.208000000000001,
9.98835756998534));
#16485=CARTESIAN_POINT('Ctrl Pts',(7.28883796912684,0.891200000000001,9.98835756998534));
#16486=CARTESIAN_POINT('Ctrl Pts',(7.41967047354988,-0.208000000000001,
9.81917361987377));
#16487=CARTESIAN_POINT('Ctrl Pts',(7.41967047354988,0.891200000000001,9.81917361987377));
#16488=CARTESIAN_POINT('Ctrl Pts',(7.54360573526532,-0.208000000000001,
9.63939026966049));
#16489=CARTESIAN_POINT('Ctrl Pts',(7.54360573526532,0.891200000000001,9.63939026966049));
#16490=CARTESIAN_POINT('Ctrl Pts',(7.6590003866074,-0.208000000000001,9.45324999450471));
#16491=CARTESIAN_POINT('Ctrl Pts',(7.6590003866074,0.891200000000001,9.45324999450471));
#16492=CARTESIAN_POINT('Ctrl Pts',(7.76209282457502,-0.208000000000001,
9.26297089919836));
#16493=CARTESIAN_POINT('Ctrl Pts',(7.76209282457502,0.891200000000001,9.26297089919836));
#16494=CARTESIAN_POINT('Ctrl Pts',(7.84862074946283,-0.208000000000001,
9.06945407017055));
#16495=CARTESIAN_POINT('Ctrl Pts',(7.84862074946283,0.891200000000001,9.06945407017055));
#16496=CARTESIAN_POINT('Ctrl Pts',(7.91508259073031,-0.208000000000001,
8.87266947141857));
#16497=CARTESIAN_POINT('Ctrl Pts',(7.91508259073031,0.891200000000001,8.87266947141857));
#16498=CARTESIAN_POINT('Ctrl Pts',(7.96007609558387,-0.208000000000001,
8.67216210283894));
#16499=CARTESIAN_POINT('Ctrl Pts',(7.96007609558387,0.891200000000001,8.67216210283894));
#16500=CARTESIAN_POINT('Ctrl Pts',(7.98575825096082,-0.208000000000001,
8.46752658699496));
#16501=CARTESIAN_POINT('Ctrl Pts',(7.98575825096082,0.891200000000001,8.46752658699496));
#16502=CARTESIAN_POINT('Ctrl Pts',(7.9987984391963,-0.208000000000001,8.25883677791438));
#16503=CARTESIAN_POINT('Ctrl Pts',(7.9987984391963,0.891200000000001,8.25883677791438));
#16504=CARTESIAN_POINT('Ctrl Pts',(8.00781893805568,-0.208000000000001,
8.04662057355209));
#16505=CARTESIAN_POINT('Ctrl Pts',(8.00781893805568,0.891200000000001,8.04662057355209));
#16506=CARTESIAN_POINT('Ctrl Pts',(8.02124364536257,-0.208000000000001,
7.8318867323277));
#16507=CARTESIAN_POINT('Ctrl Pts',(8.02124364536257,0.891200000000001,7.8318867323277));
#16508=CARTESIAN_POINT('Ctrl Pts',(8.04494633492827,-0.208000000000001,
7.61613341658679));
#16509=CARTESIAN_POINT('Ctrl Pts',(8.04494633492827,0.891200000000001,7.61613341658679));
#16510=CARTESIAN_POINT('Ctrl Pts',(8.08008348678094,-0.208000000000001,
7.40136016279815));
#16511=CARTESIAN_POINT('Ctrl Pts',(8.08008348678094,0.891200000000001,7.40136016279815));
#16512=CARTESIAN_POINT('Ctrl Pts',(8.12057943633426,-0.208000000000001,
7.19009032473197));
#16513=CARTESIAN_POINT('Ctrl Pts',(8.12057943633426,0.891200000000001,7.19009032473197));
#16514=CARTESIAN_POINT('Ctrl Pts',(8.15569042861283,-0.208000000000001,
6.98516923427904));
#16515=CARTESIAN_POINT('Ctrl Pts',(8.15569042861283,0.891200000000001,6.98516923427904));
#16516=CARTESIAN_POINT('Ctrl Pts',(8.17293082304204,-0.208000000000001,
6.78954489191915));
#16517=CARTESIAN_POINT('Ctrl Pts',(8.17293082304204,0.891200000000001,6.78954489191915));
#16518=CARTESIAN_POINT('Ctrl Pts',(8.16089752265956,-0.208000000000001,
6.60605451948904));
#16519=CARTESIAN_POINT('Ctrl Pts',(8.16089752265956,0.891200000000001,6.60605451948904));
#16520=CARTESIAN_POINT('Ctrl Pts',(8.11207116917844,-0.208000000000001,
6.43720976255638));
#16521=CARTESIAN_POINT('Ctrl Pts',(8.11207116917844,0.891200000000001,6.43720976255638));
#16522=CARTESIAN_POINT('Ctrl Pts',(8.02580908828092,-0.208000000000001,
6.28498018271691));
#16523=CARTESIAN_POINT('Ctrl Pts',(8.02580908828092,0.891200000000001,6.28498018271691));
#16524=CARTESIAN_POINT('Ctrl Pts',(7.90644860448881,-0.208000000000001,
6.15052660592943));
#16525=CARTESIAN_POINT('Ctrl Pts',(7.90644860448881,0.891200000000001,6.15052660592943));
#16526=CARTESIAN_POINT('Ctrl Pts',(7.76106756457749,-0.208000000000001,
6.03389995867286));
#16527=CARTESIAN_POINT('Ctrl Pts',(7.76106756457749,0.891200000000001,6.03389995867286));
#16528=CARTESIAN_POINT('Ctrl Pts',(7.59751903688427,-0.208000000000001,
5.93381436957244));
#16529=CARTESIAN_POINT('Ctrl Pts',(7.59751903688427,0.891200000000001,5.93381436957244));
#16530=CARTESIAN_POINT('Ctrl Pts',(7.42198551710643,-0.208000000000001,
5.84723737025948));
#16531=CARTESIAN_POINT('Ctrl Pts',(7.42198551710643,0.891200000000001,5.84723737025948));
#16532=CARTESIAN_POINT('Ctrl Pts',(7.23853768475023,-0.208000000000001,
5.76979878895671));
#16533=CARTESIAN_POINT('Ctrl Pts',(7.23853768475023,0.891200000000001,5.76979878895671));
#16534=CARTESIAN_POINT('Ctrl Pts',(7.04976847947264,-0.208000000000001,
5.69662713609756));
#16535=CARTESIAN_POINT('Ctrl Pts',(7.04976847947264,0.891200000000001,5.69662713609756));
#16536=CARTESIAN_POINT('Ctrl Pts',(6.85709976037512,-0.208000000000001,
5.62308582598972));
#16537=CARTESIAN_POINT('Ctrl Pts',(6.85709976037512,0.891200000000001,5.62308582598972));
#16538=CARTESIAN_POINT('Ctrl Pts',(6.66121503090593,-0.208000000000001,
5.54547963906641));
#16539=CARTESIAN_POINT('Ctrl Pts',(6.66121503090593,0.891200000000001,5.54547963906641));
#16540=CARTESIAN_POINT('Ctrl Pts',(6.46246210121974,-0.208000000000001,
5.46195513100458));
#16541=CARTESIAN_POINT('Ctrl Pts',(6.46246210121974,0.891200000000001,5.46195513100458));
#16542=CARTESIAN_POINT('Ctrl Pts',(6.26112587698791,-0.208000000000001,
5.37226655127806));
#16543=CARTESIAN_POINT('Ctrl Pts',(6.26112587698791,0.891200000000001,5.37226655127806));
#16544=CARTESIAN_POINT('Ctrl Pts',(6.05762450882876,-0.208000000000001,
5.27709955371581));
#16545=CARTESIAN_POINT('Ctrl Pts',(6.05762450882876,0.891200000000001,5.27709955371581));
#16546=CARTESIAN_POINT('Ctrl Pts',(5.85274048349253,-0.208000000000001,
5.17752467829117));
#16547=CARTESIAN_POINT('Ctrl Pts',(5.85274048349253,0.891200000000001,5.17752467829117));
#16548=CARTESIAN_POINT('Ctrl Pts',(5.6478173738032,-0.208000000000001,5.07442896098936));
#16549=CARTESIAN_POINT('Ctrl Pts',(5.6478173738032,0.891200000000001,5.07442896098936));
#16550=CARTESIAN_POINT('Ctrl Pts',(5.44501860313336,-0.208000000000001,
4.96787993373722));
#16551=CARTESIAN_POINT('Ctrl Pts',(5.44501860313336,0.891200000000001,4.96787993373722));
#16552=CARTESIAN_POINT('Ctrl Pts',(5.24741086000008,-0.208000000000001,
4.85676111532844));
#16553=CARTESIAN_POINT('Ctrl Pts',(5.24741086000008,0.891200000000001,4.85676111532844));
#16554=CARTESIAN_POINT('Ctrl Pts',(5.05850630701875,-0.208000000000001,
4.73929437247794));
#16555=CARTESIAN_POINT('Ctrl Pts',(5.05850630701875,0.891200000000001,4.73929437247794));
#16556=CARTESIAN_POINT('Ctrl Pts',(4.88190185104846,-0.208000000000001,
4.61340315498245));
#16557=CARTESIAN_POINT('Ctrl Pts',(4.88190185104846,0.891200000000001,4.61340315498245));
#16558=CARTESIAN_POINT('Ctrl Pts',(4.7208720035032,-0.208000000000001,4.47714872481864));
#16559=CARTESIAN_POINT('Ctrl Pts',(4.7208720035032,0.891200000000001,4.47714872481864));
#16560=CARTESIAN_POINT('Ctrl Pts',(4.57800047823784,-0.208000000000001,
4.32911151507775));
#16561=CARTESIAN_POINT('Ctrl Pts',(4.57800047823784,0.891200000000001,4.32911151507775));
#16562=CARTESIAN_POINT('Ctrl Pts',(4.4547451964031,-0.208000000000001,4.16885849319143));
#16563=CARTESIAN_POINT('Ctrl Pts',(4.4547451964031,0.891200000000001,4.16885849319143));
#16564=CARTESIAN_POINT('Ctrl Pts',(4.35148411330737,-0.208000000000001,
3.99681013615577));
#16565=CARTESIAN_POINT('Ctrl Pts',(4.35148411330737,0.891200000000001,3.99681013615577));
#16566=CARTESIAN_POINT('Ctrl Pts',(4.26765207024408,-0.208000000000001,
3.81399668859083));
#16567=CARTESIAN_POINT('Ctrl Pts',(4.26765207024408,0.891200000000001,3.81399668859083));
#16568=CARTESIAN_POINT('Ctrl Pts',(4.20184334854117,-0.208000000000001,
3.62185203209172));
#16569=CARTESIAN_POINT('Ctrl Pts',(4.20184334854117,0.891200000000001,3.62185203209172));
#16570=CARTESIAN_POINT('Ctrl Pts',(4.15193466045737,-0.208000000000001,
3.42199345348454));
#16571=CARTESIAN_POINT('Ctrl Pts',(4.15193466045737,0.891200000000001,3.42199345348454));
#16572=CARTESIAN_POINT('Ctrl Pts',(4.11518318246501,-0.208000000000001,
3.21600287470933));
#16573=CARTESIAN_POINT('Ctrl Pts',(4.11518318246501,0.891200000000001,3.21600287470933));
#16574=CARTESIAN_POINT('Ctrl Pts',(4.08854433447712,-0.208000000000001,
3.00529120729351));
#16575=CARTESIAN_POINT('Ctrl Pts',(4.08854433447712,0.891200000000001,3.00529120729351));
#16576=CARTESIAN_POINT('Ctrl Pts',(4.06899962712481,-0.208000000000001,
2.7909834104826));
#16577=CARTESIAN_POINT('Ctrl Pts',(4.06899962712481,0.891200000000001,2.7909834104826));
#16578=CARTESIAN_POINT('Ctrl Pts',(4.05390260344518,-0.208000000000001,
2.57377631141663));
#16579=CARTESIAN_POINT('Ctrl Pts',(4.05390260344518,0.891200000000001,2.57377631141663));
#16580=CARTESIAN_POINT('Ctrl Pts',(4.04126813644791,-0.208000000000001,
2.35385258470204));
#16581=CARTESIAN_POINT('Ctrl Pts',(4.04126813644791,0.891200000000001,2.35385258470204));
#16582=CARTESIAN_POINT('Ctrl Pts',(4.03021014446877,-0.208000000000001,
2.13065748555701));
#16583=CARTESIAN_POINT('Ctrl Pts',(4.03021014446877,0.891200000000001,2.13065748555701));
#16584=CARTESIAN_POINT('Ctrl Pts',(4.02110299519686,-0.208000000000001,
1.91370945705801));
#16585=CARTESIAN_POINT('Ctrl Pts',(4.02110299519686,0.891200000000001,1.91370945705801));
#16586=CARTESIAN_POINT('Ctrl Pts',(4.0150839653859,-0.208000000000001,1.73897559179867));
#16587=CARTESIAN_POINT('Ctrl Pts',(4.0150839653859,0.891200000000001,1.73897559179867));
#16588=CARTESIAN_POINT('Ctrl Pts',(4.01123999191373,-0.208000000000001,
1.60904011456728));
#16589=CARTESIAN_POINT('Ctrl Pts',(4.01123999191373,0.891200000000001,1.60904011456728));
#16590=CARTESIAN_POINT('Ctrl Pts',(4.0089337502854,-0.208000000000001,1.52556315247963));
#16591=CARTESIAN_POINT('Ctrl Pts',(4.0089337502854,0.891200000000001,1.52556315247963));
#16592=CARTESIAN_POINT('Ctrl Pts',(4.00794703095364,-0.208000000000001,
1.48914872207946));
#16593=CARTESIAN_POINT('Ctrl Pts',(4.00794703095364,0.891200000000001,1.48914872207946));
#16594=CARTESIAN_POINT('',(4.,0.5,1.2));
#16595=CARTESIAN_POINT('Ctrl Pts',(3.99628071248376,0.515724022809955,1.08895058147551));
#16596=CARTESIAN_POINT('Ctrl Pts',(3.99695111863745,0.510515400451476,1.10697360799751));
#16597=CARTESIAN_POINT('Ctrl Pts',(3.99759476802297,0.506584394748987,1.12533130577593));
#16598=CARTESIAN_POINT('Ctrl Pts',(3.99821367094827,0.503955544636118,1.14388558371581));
#16599=CARTESIAN_POINT('Ctrl Pts',(3.99883257387358,0.501326694523249,1.16243986165569));
#16600=CARTESIAN_POINT('Ctrl Pts',(3.9994268264293,0.5,1.18119071480602));
#16601=CARTESIAN_POINT('Ctrl Pts',(4.,0.5,1.2));
#16602=CARTESIAN_POINT('',(4.00232316926925,0.5,1.28));
#16603=CARTESIAN_POINT('Ctrl Pts',(4.,0.5,1.2));
#16604=CARTESIAN_POINT('Ctrl Pts',(4.00048648979365,0.5,1.21596466714547));
#16605=CARTESIAN_POINT('Ctrl Pts',(4.00095995114739,0.5,1.23195096410174));
#16606=CARTESIAN_POINT('Ctrl Pts',(4.00142258957318,0.5,1.2479547597375));
#16607=CARTESIAN_POINT('Ctrl Pts',(4.00187639644938,0.5,1.26397226336412));
#16608=CARTESIAN_POINT('Ctrl Pts',(4.00232316926925,0.5,1.28));
#16609=CARTESIAN_POINT('',(4.,0.42,1.2));
#16610=CARTESIAN_POINT('Ctrl Pts',(4.00232316926925,0.5,1.28000000000001));
#16611=CARTESIAN_POINT('Ctrl Pts',(4.00230299966747,0.5,1.2792764262932));
#16612=CARTESIAN_POINT('Ctrl Pts',(4.00228281233137,0.499990182776602,1.27855285870449));
#16613=CARTESIAN_POINT('Ctrl Pts',(4.00214695508649,0.499858141613736,1.27368777894256));
#16614=CARTESIAN_POINT('Ctrl Pts',(4.0020311113454,0.499424139669874,1.26956098182442));
#16615=CARTESIAN_POINT('Ctrl Pts',(4.00163265096412,0.496820195244168,1.25544601244678));
#16616=CARTESIAN_POINT('Ctrl Pts',(4.00135768601021,0.493062784524195,1.24585198650422));
#16617=CARTESIAN_POINT('Ctrl Pts',(4.00086839188745,0.482409927602859,1.22901639363533));
#16618=CARTESIAN_POINT('Ctrl Pts',(4.00065589411436,0.475764975074544,1.22182250919509));
#16619=CARTESIAN_POINT('Ctrl Pts',(4.00029434770309,0.459596631686721,1.20969879529552));
#16620=CARTESIAN_POINT('Ctrl Pts',(4.00015547253981,0.450041622442072,1.20511554604908));
#16621=CARTESIAN_POINT('Ctrl Pts',(4.0000256112516,0.433366702909574,1.20083901694649));
#16622=CARTESIAN_POINT('Ctrl Pts',(4.,0.426689213070844,1.2));
#16623=CARTESIAN_POINT('Ctrl Pts',(4.,0.420000000000006,1.2));
#16624=CARTESIAN_POINT('',(4.,0.08,1.2));
#16625=CARTESIAN_POINT('',(4.,0.,1.2));
#16626=CARTESIAN_POINT('',(4.00232316926925,0.,1.28));
#16627=CARTESIAN_POINT('Ctrl Pts',(4.,0.0799999999999845,1.2));
#16628=CARTESIAN_POINT('Ctrl Pts',(4.,0.0712353307855553,1.2));
#16629=CARTESIAN_POINT('Ctrl Pts',(4.00004401876777,0.0625213699048051,
1.20144045396));
#16630=CARTESIAN_POINT('Ctrl Pts',(4.00022068673853,0.0453965107457132,
1.20727262474139));
#16631=CARTESIAN_POINT('Ctrl Pts',(4.00035699792145,0.0371755072686487,
1.21178919233617));
#16632=CARTESIAN_POINT('Ctrl Pts',(4.00068867210099,0.0232931356215582,
1.22293442282227));
#16633=CARTESIAN_POINT('Ctrl Pts',(4.00087563722023,0.0175589585117979,
1.22927281222884));
#16634=CARTESIAN_POINT('Ctrl Pts',(4.0012611591677,0.00894266831347314,
1.24252529496691));
#16635=CARTESIAN_POINT('Ctrl Pts',(4.00145268528988,0.00581567214900459,
1.24917507680124));
#16636=CARTESIAN_POINT('Ctrl Pts',(4.0018273760135,0.00170830451366606,
1.2623297822669));
#16637=CARTESIAN_POINT('Ctrl Pts',(4.00200757811868,0.000536463326316975,
1.26871413063067));
#16638=CARTESIAN_POINT('Ctrl Pts',(4.00221809264031,8.14663303026943E-5,
1.27623581107857));
#16639=CARTESIAN_POINT('Ctrl Pts',(4.00224792817779,3.83285587785669E-5,
1.27730329002437));
#16640=CARTESIAN_POINT('Ctrl Pts',(4.00229289069437,5.52723888419683E-6,
1.27891413388588));
#16641=CARTESIAN_POINT('Ctrl Pts',(4.00230803498764,-4.43319744566652E-17,
1.27945706571897));
#16642=CARTESIAN_POINT('Ctrl Pts',(4.00232316926925,-2.77555756156289E-17,
1.28));
#16643=CARTESIAN_POINT('',(4.,0.,1.2));
#16644=CARTESIAN_POINT('Ctrl Pts',(4.00232316926925,-5.55111512312578E-17,
1.28));
#16645=CARTESIAN_POINT('Ctrl Pts',(4.00187639644938,-5.55111512312578E-17,
1.26397226336412));
#16646=CARTESIAN_POINT('Ctrl Pts',(4.00142258957318,-5.55111512312578E-17,
1.2479547597375));
#16647=CARTESIAN_POINT('Ctrl Pts',(4.00095995114739,-5.55111512312578E-17,
1.23195096410174));
#16648=CARTESIAN_POINT('Ctrl Pts',(4.00048648979365,-5.55111512312578E-17,
1.21596466714547));
#16649=CARTESIAN_POINT('Ctrl Pts',(4.,-5.55111512312578E-17,1.2));
#16650=CARTESIAN_POINT('Origin',(3.96221895354333,0.899296250818234,1.20115091904051));
#16651=CARTESIAN_POINT('Ctrl Pts',(2.8805419932544,0.136565758583769,0.899998731395832));
#16652=CARTESIAN_POINT('Ctrl Pts',(2.88783884470249,0.181143949322972,0.77752115893973));
#16653=CARTESIAN_POINT('Ctrl Pts',(2.8993736353594,0.270316072740132,0.532522763406263));
#16654=CARTESIAN_POINT('Ctrl Pts',(2.9196026767358,0.376119687828295,0.241829720054866));
#16655=CARTESIAN_POINT('Ctrl Pts',(2.9730125063753,0.451017094008355,0.0360507877994292));
#16656=CARTESIAN_POINT('Ctrl Pts',(3.01389049537916,0.482936356580544,-0.0516466653633009));
#16657=CARTESIAN_POINT('Ctrl Pts',(3.05985159914742,0.506141825662096,-0.115403167672718));
#16658=CARTESIAN_POINT('Ctrl Pts',(3.11058052482755,0.52437488961235,-0.165498099163513));
#16659=CARTESIAN_POINT('Ctrl Pts',(3.21732310712232,0.544182531031752,-0.219919146695976));
#16660=CARTESIAN_POINT('Ctrl Pts',(3.35194656845354,0.548863870554337,-0.232781021327076));
#16661=CARTESIAN_POINT('Ctrl Pts',(3.49778753718399,0.541692651427306,-0.213078258705599));
#16662=CARTESIAN_POINT('Ctrl Pts',(3.6265539989599,0.526408247588463,-0.171084704288551));
#16663=CARTESIAN_POINT('Ctrl Pts',(3.73739288004811,0.503000447457269,-0.10677230198899));
#16664=CARTESIAN_POINT('Ctrl Pts',(3.84808202669468,0.46276591626256,0.00377116395081768));
#16665=CARTESIAN_POINT('Ctrl Pts',(3.9204363567822,0.403359946625806,0.166987724108605));
#16666=CARTESIAN_POINT('Ctrl Pts',(3.96110129343823,0.333991249229589,0.357576653821691));
#16667=CARTESIAN_POINT('Ctrl Pts',(3.98904669612228,0.242194739655562,0.60978549106108));
#16668=CARTESIAN_POINT('Ctrl Pts',(3.99598983762634,0.174461093782049,0.795882153635894));
#16669=CARTESIAN_POINT('Ctrl Pts',(4.,0.129452050955555,0.919543482472952));
#16670=CARTESIAN_POINT('Ctrl Pts',(2.8805419932544,0.114073328609723,0.891812156388963));
#16671=CARTESIAN_POINT('Ctrl Pts',(2.88783872593927,0.158650793796348,0.769336577372186));
#16672=CARTESIAN_POINT('Ctrl Pts',(2.89937600566135,0.247822523947933,0.524339262327005));
#16673=CARTESIAN_POINT('Ctrl Pts',(2.9195545062059,0.353605214767559,0.233703707930933));
#16674=CARTESIAN_POINT('Ctrl Pts',(2.97295217221839,0.428508407704055,0.0279088766928571));
#16675=CARTESIAN_POINT('Ctrl Pts',(3.01382111580078,0.460433630477054,-0.0598049519870154));
#16676=CARTESIAN_POINT('Ctrl Pts',(3.05980698983149,0.483652921552891,-0.123599429913622));
#16677=CARTESIAN_POINT('Ctrl Pts',(3.11055009633998,0.501895319408686,-0.173720006099127));
#16678=CARTESIAN_POINT('Ctrl Pts',(3.21736084446955,0.521716087056444,-0.228177117647598));
#16679=CARTESIAN_POINT('Ctrl Pts',(3.35195992956318,0.526387882971129,-0.241012771431496));
#16680=CARTESIAN_POINT('Ctrl Pts',(3.4978195772253,0.519215743708778,-0.221307480759004));
#16681=CARTESIAN_POINT('Ctrl Pts',(3.62657748910597,0.503928259570136,-0.179305463287815));
#16682=CARTESIAN_POINT('Ctrl Pts',(3.73742854793082,0.480515769664525,-0.114980175938938));
#16683=CARTESIAN_POINT('Ctrl Pts',(3.8481659110119,0.440262093407297,-0.00438410937216693));
#16684=CARTESIAN_POINT('Ctrl Pts',(3.92047099581111,0.380857917917725,0.158827521406752));
#16685=CARTESIAN_POINT('Ctrl Pts',(3.96112079679389,0.311492110423669,0.349408511178906));
#16686=CARTESIAN_POINT('Ctrl Pts',(3.98905963354223,0.219691592626807,0.601628360920028));
#16687=CARTESIAN_POINT('Ctrl Pts',(3.99598979363886,0.151969157512326,0.787694222187545));
#16688=CARTESIAN_POINT('Ctrl Pts',(4.,0.106959620981509,0.911356907466082));
#16689=CARTESIAN_POINT('Ctrl Pts',(2.90060526052275,0.0747531580267383,
0.878696094802245));
#16690=CARTESIAN_POINT('Ctrl Pts',(2.90791147887875,0.11938857342105,0.756061298898396));
#16691=CARTESIAN_POINT('Ctrl Pts',(2.91940548593204,0.208587912033988,0.510988130229062));
#16692=CARTESIAN_POINT('Ctrl Pts',(2.93971734293678,0.313973665333152,0.221443152707394));
#16693=CARTESIAN_POINT('Ctrl Pts',(2.99225360162521,0.387510002496177,0.0194037268425803));
#16694=CARTESIAN_POINT('Ctrl Pts',(3.03182463200544,0.418305990574516,-0.0652075550124495));
#16695=CARTESIAN_POINT('Ctrl Pts',(3.07550932869219,0.440350515088388,-0.125774388336927));
#16696=CARTESIAN_POINT('Ctrl Pts',(3.12310116181815,0.457414736169163,-0.172657950436938));
#16697=CARTESIAN_POINT('Ctrl Pts',(3.22253873842663,0.475909198392738,-0.223471067781167));
#16698=CARTESIAN_POINT('Ctrl Pts',(3.35113610177915,0.480513385154656,-0.236120966944487));
#16699=CARTESIAN_POINT('Ctrl Pts',(3.49306055599084,0.473537376896056,-0.216954541776055));
#16700=CARTESIAN_POINT('Ctrl Pts',(3.61818010203025,0.458676526293589,-0.176124690311888));
#16701=CARTESIAN_POINT('Ctrl Pts',(3.72462733520835,0.436152051570704,-0.114239204625684));
#16702=CARTESIAN_POINT('Ctrl Pts',(3.83038111193484,0.397744836296198,-0.00871624791484828));
#16703=CARTESIAN_POINT('Ctrl Pts',(3.9009685656033,0.340106698388871,0.149643234484944));
#16704=CARTESIAN_POINT('Ctrl Pts',(3.94117885677219,0.271582068768333,0.337913107043865));
#16705=CARTESIAN_POINT('Ctrl Pts',(3.96895833352272,0.180412639324759,0.588399055784644));
#16706=CARTESIAN_POINT('Ctrl Pts',(3.97590794636788,0.112784383202069,0.774206162398828));
#16707=CARTESIAN_POINT('Ctrl Pts',(3.97991463942917,0.0678142790554765,
0.897760508092115));
#16708=CARTESIAN_POINT('Ctrl Pts',(2.94249302709539,0.0602041295977449,
0.875896230734658));
#16709=CARTESIAN_POINT('Ctrl Pts',(2.9498187182991,0.104958509222874,0.752934583292915));
#16710=CARTESIAN_POINT('Ctrl Pts',(2.96122932239305,0.194214391674412,0.507706061703817));
#16711=CARTESIAN_POINT('Ctrl Pts',(2.98167866039825,0.298713075662704,0.220598287083263));
#16712=CARTESIAN_POINT('Ctrl Pts',(3.03238256717175,0.369411850319645,0.0263550001302063));
#16713=CARTESIAN_POINT('Ctrl Pts',(3.06921861113533,0.397866861024811,-0.0518244992525782));
#16714=CARTESIAN_POINT('Ctrl Pts',(3.10816802129538,0.417497270910729,-0.105758607148775));
#16715=CARTESIAN_POINT('Ctrl Pts',(3.14922022130347,0.432127742064011,-0.145955496278401));
#16716=CARTESIAN_POINT('Ctrl Pts',(3.23345429671096,0.44788976904434,-0.189261309491687));
#16717=CARTESIAN_POINT('Ctrl Pts',(3.34945338625923,0.452326189141897,-0.201450273532941));
#16718=CARTESIAN_POINT('Ctrl Pts',(3.48321409508734,0.445757094142106,-0.183401833354763));
#16719=CARTESIAN_POINT('Ctrl Pts',(3.60071367717697,0.431778372428901,-0.144995611094893));
#16720=CARTESIAN_POINT('Ctrl Pts',(3.69800063294054,0.411094803582314,-0.0881679727351601));
#16721=CARTESIAN_POINT('Ctrl Pts',(3.79348421490767,0.376489211798969,0.00691010927644513));
#16722=CARTESIAN_POINT('Ctrl Pts',(3.86034830022832,0.322543181908982,0.15512560826841));
#16723=CARTESIAN_POINT('Ctrl Pts',(3.89959878244922,0.255782808716465,0.338548226129213));
#16724=CARTESIAN_POINT('Ctrl Pts',(3.9270272401522,0.165919778027693,0.585444873790373));
#16725=CARTESIAN_POINT('Ctrl Pts',(3.93398126610095,0.0985194096795488,
0.770625863889823));
#16726=CARTESIAN_POINT('Ctrl Pts',(3.9379807468151,0.0536302550833677,0.893957802521238));
#16727=CARTESIAN_POINT('Ctrl Pts',(2.96041691837963,0.0598609284456541,
0.876839168150358));
#16728=CARTESIAN_POINT('Ctrl Pts',(2.96775093160951,0.104666149296221,0.753737835589749));
#16729=CARTESIAN_POINT('Ctrl Pts',(2.97912606655434,0.193946192378553,0.508442933213105));
#16730=CARTESIAN_POINT('Ctrl Pts',(2.99962978200786,0.298063454185075,0.22238310742424));
#16731=CARTESIAN_POINT('Ctrl Pts',(3.04954854909233,0.3675485376204,0.0314744096967656));
#16732=CARTESIAN_POINT('Ctrl Pts',(3.08521348818013,0.395002362532113,-0.0439543543258271));
#16733=CARTESIAN_POINT('Ctrl Pts',(3.12213883760405,0.413600983366687,-0.095053645101818));
#16734=CARTESIAN_POINT('Ctrl Pts',(3.16039395937928,0.427190868210603,-0.132391546843465));
#16735=CARTESIAN_POINT('Ctrl Pts',(3.23812841779038,0.441784834591999,-0.172488139936633));
#16736=CARTESIAN_POINT('Ctrl Pts',(3.34873452432173,0.446148626378716,-0.184477559333837));
#16737=CARTESIAN_POINT('Ctrl Pts',(3.47900358892302,0.439753569654038,-0.166907285386653));
#16738=CARTESIAN_POINT('Ctrl Pts',(3.59324181436642,0.426152042057545,-0.129537395445201));
#16739=CARTESIAN_POINT('Ctrl Pts',(3.68661013453806,0.406255788910909,-0.074872889193063));
#16740=CARTESIAN_POINT('Ctrl Pts',(3.77770331808059,0.373275236268507,0.0157404344730694));
#16741=CARTESIAN_POINT('Ctrl Pts',(3.84296982682103,0.320909227628625,0.15961486075811));
#16742=CARTESIAN_POINT('Ctrl Pts',(3.88180827116063,0.254904039155253,0.340962625655547));
#16743=CARTESIAN_POINT('Ctrl Pts',(3.90908594858962,0.165599667112526,0.586324371301513));
#16744=CARTESIAN_POINT('Ctrl Pts',(3.91604071966527,0.0982977998881255,
0.771234731787688));
#16745=CARTESIAN_POINT('Ctrl Pts',(3.92003711807002,0.053443240348906,0.894471621281276));
#16746=CARTESIAN_POINT('',(2.96041691837963,0.0598609284456542,0.876839168150358));
#16747=CARTESIAN_POINT('Ctrl Pts',(3.91996278980377,0.0542766424889417,
0.892181867720203));
#16748=CARTESIAN_POINT('Ctrl Pts',(3.91598305831422,0.098853560185636,0.769707792919649));
#16749=CARTESIAN_POINT('Ctrl Pts',(3.90900147842788,0.165876213955253,0.585564565095701));
#16750=CARTESIAN_POINT('Ctrl Pts',(3.8818082711687,0.25490403915566,0.340962625654429));
#16751=CARTESIAN_POINT('Ctrl Pts',(3.84296982682819,0.320909227629314,0.159614860756216));
#16752=CARTESIAN_POINT('Ctrl Pts',(3.77770331808652,0.373275236269741,0.0157404344696786));
#16753=CARTESIAN_POINT('Ctrl Pts',(3.68661013454203,0.406255788912611,-0.0748728891977425));
#16754=CARTESIAN_POINT('Ctrl Pts',(3.59324181436885,0.426152042059393,-0.129537395450278));
#16755=CARTESIAN_POINT('Ctrl Pts',(3.47900358892426,0.439753569655855,-0.166907285391647));
#16756=CARTESIAN_POINT('Ctrl Pts',(3.34873452432189,0.446148626380414,-0.184477559338504));
#16757=CARTESIAN_POINT('Ctrl Pts',(3.23812841778915,0.441784834593533,-0.172488139940845));
#16758=CARTESIAN_POINT('Ctrl Pts',(3.16039395937664,0.42719086821175,-0.132391546846618));
#16759=CARTESIAN_POINT('Ctrl Pts',(3.12213883760094,0.413600983367549,-0.0950536451041868));
#16760=CARTESIAN_POINT('Ctrl Pts',(3.0852134881768,0.395002362532705,-0.0439543543274574));
#16761=CARTESIAN_POINT('Ctrl Pts',(3.04954854908906,0.367548537620745,0.0314744096958174));
#16762=CARTESIAN_POINT('Ctrl Pts',(2.99962978200522,0.298063454185146,0.222383107424044));
#16763=CARTESIAN_POINT('Ctrl Pts',(2.97912606655288,0.193946192378579,0.508442933213033));
#16764=CARTESIAN_POINT('Ctrl Pts',(2.96775093160902,0.10466614929623,0.753737835589723));
#16765=CARTESIAN_POINT('Ctrl Pts',(2.96041691837963,0.0598609284456542,
0.876839168150358));
#16766=CARTESIAN_POINT('',(2.88054198318953,0.136565694403419,0.899998899355773));
#16767=CARTESIAN_POINT('Origin',(2.96041691837963,0.135036338108527,0.904200779616412));
#16768=CARTESIAN_POINT('Ctrl Pts',(2.8805419932544,0.136565756430656,0.899998730612164));
#16769=CARTESIAN_POINT('Ctrl Pts',(2.88284752702291,0.150650807367472,0.86130037131219));
#16770=CARTESIAN_POINT('Ctrl Pts',(2.88498553892976,0.164719389055088,0.822647260902508));
#16771=CARTESIAN_POINT('Ctrl Pts',(2.88704880814836,0.178807167502167,0.783941407829676));
#16772=CARTESIAN_POINT('Ctrl Pts',(2.88896759991875,0.19190846960258,0.747945876237076));
#16773=CARTESIAN_POINT('Ctrl Pts',(2.89082106771812,0.205026680469038,0.711903888191579));
#16774=CARTESIAN_POINT('Ctrl Pts',(2.89270923333433,0.218175254353227,0.675778478440476));
#16775=CARTESIAN_POINT('Ctrl Pts',(2.8943613782485,0.229680256501893,0.644168744908261));
#16776=CARTESIAN_POINT('Ctrl Pts',(2.8960399023492,0.241208574106251,0.612494952688007));
#16777=CARTESIAN_POINT('Ctrl Pts',(2.89783714020707,0.252754941297751,0.58077156963465));
#16778=CARTESIAN_POINT('Ctrl Pts',(2.89864412818268,0.25793944119282,0.566527273278611));
#16779=CARTESIAN_POINT('Ctrl Pts',(2.89947544083931,0.263127363552645,0.552273573777938));
#16780=CARTESIAN_POINT('Ctrl Pts',(2.90034147758514,0.268317099136106,0.538014892486267));
#16781=CARTESIAN_POINT('Ctrl Pts',(2.9008098570909,0.271123868940463,0.530303355847108));
#16782=CARTESIAN_POINT('Ctrl Pts',(2.9012883190563,0.273930533419183,0.522592108587758));
#16783=CARTESIAN_POINT('Ctrl Pts',(2.90177824359068,0.276734477144718,0.514888336536346));
#16784=CARTESIAN_POINT('Ctrl Pts',(2.90336905113846,0.285839011678269,0.489873833555445));
#16785=CARTESIAN_POINT('Ctrl Pts',(2.90508092831803,0.294927759204885,0.464902705019619));
#16786=CARTESIAN_POINT('Ctrl Pts',(2.9069985081457,0.304047491932523,0.439846445343648));
#16787=CARTESIAN_POINT('Ctrl Pts',(2.90873365103152,0.312299580911864,0.417174017268099));
#16788=CARTESIAN_POINT('Ctrl Pts',(2.91063698175396,0.320577156553037,0.39443156516467));
#16789=CARTESIAN_POINT('Ctrl Pts',(2.91279212081837,0.328903729190399,0.371554494920593));
#16790=CARTESIAN_POINT('Ctrl Pts',(2.91480972174193,0.336698910912354,0.350137409213762));
#16791=CARTESIAN_POINT('Ctrl Pts',(2.91704780723451,0.344537153750784,0.328602014061762));
#16792=CARTESIAN_POINT('Ctrl Pts',(2.91959741789068,0.352425801447324,0.306928132700273));
#16793=CARTESIAN_POINT('Ctrl Pts',(2.92200870659192,0.359886472751267,0.286430106810531));
#16794=CARTESIAN_POINT('Ctrl Pts',(2.92469846160555,0.367392338442971,0.265807910360929));
#16795=CARTESIAN_POINT('Ctrl Pts',(2.92776715496281,0.374936938954671,0.245079290868043));
#16796=CARTESIAN_POINT('Ctrl Pts',(2.93069401968964,0.382132843707919,0.225308705095369));
#16797=CARTESIAN_POINT('Ctrl Pts',(2.93396547545055,0.389364082820534,0.205441038968201));
#16798=CARTESIAN_POINT('Ctrl Pts',(2.9376928277366,0.39661170582491,0.18552835846838));
#16799=CARTESIAN_POINT('Ctrl Pts',(2.93958647111764,0.400293786904793,0.175411923869907));
#16800=CARTESIAN_POINT('Ctrl Pts',(2.94159818848892,0.403979870729996,0.165284491819052));
#16801=CARTESIAN_POINT('Ctrl Pts',(2.94374529812117,0.407665924548674,0.155157142210448));
#16802=CARTESIAN_POINT('Ctrl Pts',(2.94585156221408,0.411281856723828,0.145222450233562));
#16803=CARTESIAN_POINT('Ctrl Pts',(2.94808951946978,0.414900689447676,0.135279789064636));
#16804=CARTESIAN_POINT('Ctrl Pts',(2.9504855759059,0.418527466733358,0.125315300391463));
#16805=CARTESIAN_POINT('Ctrl Pts',(2.95400177923571,0.423849748035309,0.11069245273051));
#16806=CARTESIAN_POINT('Ctrl Pts',(2.95785705464788,0.429189653995361,0.0960211817194013));
#16807=CARTESIAN_POINT('Ctrl Pts',(2.96215449172343,0.434550976790958,0.0812910684362362));
#16808=CARTESIAN_POINT('Ctrl Pts',(2.96625355726838,0.439664818636796,0.067240903472608));
#16809=CARTESIAN_POINT('Ctrl Pts',(2.97075478982208,0.444798246534775,0.0531369262729893));
#16810=CARTESIAN_POINT('Ctrl Pts',(2.97577209874859,0.449940564089527,0.0390085249421184));
#16811=CARTESIAN_POINT('Ctrl Pts',(2.97918365263398,0.453437118455781,0.0294018207983813));
#16812=CARTESIAN_POINT('Ctrl Pts',(2.9828331038583,0.456936448561027,0.0197874903744428));
#16813=CARTESIAN_POINT('Ctrl Pts',(2.98676781952857,0.460434520497467,0.0101766167408878));
#16814=CARTESIAN_POINT('Ctrl Pts',(2.99149133630772,0.46463385861261,-0.00136096987898278));
#16815=CARTESIAN_POINT('Ctrl Pts',(2.99662739646606,0.468834248967704,-0.012901447504355));
#16816=CARTESIAN_POINT('Ctrl Pts',(3.00229038497435,0.473028530998255,-0.0244251426459792));
#16817=CARTESIAN_POINT('Ctrl Pts',(3.00781030054253,0.477116846318673,-0.0356576966450058));
#16818=CARTESIAN_POINT('Ctrl Pts',(3.01383080706225,0.481199452809662,-0.0468745657640879));
#16819=CARTESIAN_POINT('Ctrl Pts',(3.02048134180172,0.485255100567417,-0.058017366372349));
#16820=CARTESIAN_POINT('Ctrl Pts',(3.0267482302952,0.489076792094842,-0.0685173775222242));
#16821=CARTESIAN_POINT('Ctrl Pts',(3.03357181695739,0.492873280426181,-0.0789481434599518));
#16822=CARTESIAN_POINT('Ctrl Pts',(3.04109585537297,0.49662045126684,-0.0892434107056537));
#16823=CARTESIAN_POINT('Ctrl Pts',(3.04486925792249,0.498499705893495,-0.0944066203448309));
#16824=CARTESIAN_POINT('Ctrl Pts',(3.04881908834144,0.500366209445059,-0.0995347966931213));
#16825=CARTESIAN_POINT('Ctrl Pts',(3.05296508290757,0.502214984022785,-0.104614263086121));
#16826=CARTESIAN_POINT('Ctrl Pts',(3.060391064349,0.505526364557563,-0.113712206309427));
#16827=CARTESIAN_POINT('Ctrl Pts',(3.06845132453832,0.508780407076342,-0.122652614628499));
#16828=CARTESIAN_POINT('Ctrl Pts',(3.07713855153503,0.511902111536166,-0.131229427118859));
#16829=CARTESIAN_POINT('Ctrl Pts',(3.08491334356286,0.514695937800484,-0.138905401673171));
#16830=CARTESIAN_POINT('Ctrl Pts',(3.09319019714925,0.517383779610739,-0.146290186333133));
#16831=CARTESIAN_POINT('Ctrl Pts',(3.10194077335529,0.51992284141446,-0.153266201284675));
#16832=CARTESIAN_POINT('Ctrl Pts',(3.10852358399233,0.521832905695494,-0.158514059750891));
#16833=CARTESIAN_POINT('Ctrl Pts',(3.11537464890556,0.523659162604978,-0.16353165935619));
#16834=CARTESIAN_POINT('Ctrl Pts',(3.12247262936851,0.525387979268932,-0.168281544087149));
#16835=CARTESIAN_POINT('Ctrl Pts',(3.1307377782938,0.527401076834736,-0.173812484174152));
#16836=CARTESIAN_POINT('Ctrl Pts',(3.13933120153844,0.529279332314368,-0.178972948674204));
#16837=CARTESIAN_POINT('Ctrl Pts',(3.14814690854809,0.5310009427641,-0.183703034491738));
#16838=CARTESIAN_POINT('Ctrl Pts',(3.15731996650597,0.532792339916818,-0.188624857699165));
#16839=CARTESIAN_POINT('Ctrl Pts',(3.16673349682595,0.534414126214741,-0.19308067891295));
#16840=CARTESIAN_POINT('Ctrl Pts',(3.17624049743953,0.535859067329586,-0.197050621979487));
#16841=CARTESIAN_POINT('Ctrl Pts',(3.18104129060916,0.5365887257904,-0.199055342114923));
#16842=CARTESIAN_POINT('Ctrl Pts',(3.18586550820414,0.537273559539332,-0.200936907366632));
#16843=CARTESIAN_POINT('Ctrl Pts',(3.19069207830152,0.537914163621228,-0.202696952606885));
#16844=CARTESIAN_POINT('Ctrl Pts',(3.20477225839308,0.539782948422546,-0.207831396622426));
#16845=CARTESIAN_POINT('Ctrl Pts',(3.21888668941886,0.541279553722331,-0.211943285861518));
#16846=CARTESIAN_POINT('Ctrl Pts',(3.232951619864,0.542478223729469,-0.215236604611607));
#16847=CARTESIAN_POINT('Ctrl Pts',(3.24728773102728,0.543700004849358,-0.218593420621578));
#16848=CARTESIAN_POINT('Ctrl Pts',(3.26157252361816,0.544612257958954,-0.22109981541258));
#16849=CARTESIAN_POINT('Ctrl Pts',(3.27574767618657,0.545277946538929,-0.222928779726012));
#16850=CARTESIAN_POINT('Ctrl Pts',(3.29045467092517,0.545968611305745,-0.224826365547746));
#16851=CARTESIAN_POINT('Ctrl Pts',(3.30504387474672,0.546393830448175,-0.225994645510384));
#16852=CARTESIAN_POINT('Ctrl Pts',(3.31947992236691,0.546607405586862,-0.226581438351777));
#16853=CARTESIAN_POINT('Ctrl Pts',(3.32858799458099,0.546742155612456,-0.226951660985751));
#16854=CARTESIAN_POINT('Ctrl Pts',(3.33763568635411,0.54679232725762,-0.22708950642932));
#16855=CARTESIAN_POINT('Ctrl Pts',(3.34661911478556,0.546768383881266,-0.227023722524826));
#16856=CARTESIAN_POINT('Ctrl Pts',(3.35530982102777,0.546745220692298,-0.226960082168163));
#16857=CARTESIAN_POINT('Ctrl Pts',(3.36393308913914,0.546652688354262,-0.22670585164083));
#16858=CARTESIAN_POINT('Ctrl Pts',(3.37248678968118,0.546498757350756,-0.226282929666532));
#16859=CARTESIAN_POINT('Ctrl Pts',(3.38746886531583,0.5462291423548,-0.225542168521652));
#16860=CARTESIAN_POINT('Ctrl Pts',(3.40224291180634,0.545772076519649,-0.224286390428826));
#16861=CARTESIAN_POINT('Ctrl Pts',(3.41684838029837,0.545155788972577,-0.222593154277811));
#16862=CARTESIAN_POINT('Ctrl Pts',(3.43217875145474,0.544508913670987,-0.220815878960379));
#16863=CARTESIAN_POINT('Ctrl Pts',(3.44732409536616,0.543686565379946,-0.218556495566705));
#16864=CARTESIAN_POINT('Ctrl Pts',(3.46234328791778,0.542702696012868,-0.215853336663856));
#16865=CARTESIAN_POINT('Ctrl Pts',(3.47471047134688,0.541892553064698,-0.213627487179962));
#16866=CARTESIAN_POINT('Ctrl Pts',(3.48699354766808,0.540972452748603,-0.211099532310594));
#16867=CARTESIAN_POINT('Ctrl Pts',(3.4992235181442,0.539941812764334,-0.208267872198965));
#16868=CARTESIAN_POINT('Ctrl Pts',(3.51606259294448,0.538522755880987,-0.20436904541751));
#16869=CARTESIAN_POINT('Ctrl Pts',(3.53278579816242,0.536895749242862,-0.19989888138042));
#16870=CARTESIAN_POINT('Ctrl Pts',(3.54937570118406,0.535050013825628,-0.194827764961743));
#16871=CARTESIAN_POINT('Ctrl Pts',(3.56588793090174,0.533212920072418,-0.189780391320013));
#16872=CARTESIAN_POINT('Ctrl Pts',(3.58226861273737,0.531159094717761,-0.184137552497226));
#16873=CARTESIAN_POINT('Ctrl Pts',(3.59849464287997,0.528860502418511,-0.17782222202114));
#16874=CARTESIAN_POINT('Ctrl Pts',(3.61188615228933,0.526963450574455,-0.172610114885227));
#16875=CARTESIAN_POINT('Ctrl Pts',(3.62517276692824,0.524899303618216,-0.166938917701686));
#16876=CARTESIAN_POINT('Ctrl Pts',(3.6383336937211,0.522643621255268,-0.160741481313188));
#16877=CARTESIAN_POINT('Ctrl Pts',(3.65581519087164,0.519647426122431,-0.15250950280048));
#16878=CARTESIAN_POINT('Ctrl Pts',(3.67305736175662,0.516313909635384,-0.143350741483978));
#16879=CARTESIAN_POINT('Ctrl Pts',(3.68980508007049,0.512617597665949,-0.133195207771734));
#16880=CARTESIAN_POINT('Ctrl Pts',(3.70149620034588,0.510037304219394,-0.126105909763166));
#16881=CARTESIAN_POINT('Ctrl Pts',(3.71294709160308,0.507280253568292,-0.118530975326379));
#16882=CARTESIAN_POINT('Ctrl Pts',(3.72408551786322,0.504340318645617,-0.11045357048307));
#16883=CARTESIAN_POINT('Ctrl Pts',(3.73141197837736,0.502406534049653,-0.105140540952761));
#16884=CARTESIAN_POINT('Ctrl Pts',(3.73860597392585,0.500392914616266,-0.0996081670093482));
#16885=CARTESIAN_POINT('Ctrl Pts',(3.74564087975467,0.498301423080776,-0.0938618412238027));
#16886=CARTESIAN_POINT('Ctrl Pts',(3.7558814748348,0.495256873736462,-0.0854970106205085));
#16887=CARTESIAN_POINT('Ctrl Pts',(3.76577710849098,0.49204828623515,-0.0766814888849327));
#16888=CARTESIAN_POINT('Ctrl Pts',(3.77523378380848,0.488702069947446,-0.0674878351664772));
#16889=CARTESIAN_POINT('Ctrl Pts',(3.78430306882689,0.485492930558862,-0.0586707971342026));
#16890=CARTESIAN_POINT('Ctrl Pts',(3.79296886515126,0.482157211977029,-0.0495059856267071));
#16891=CARTESIAN_POINT('Ctrl Pts',(3.8011755061435,0.478730534395561,-0.0400912663216156));
#16892=CARTESIAN_POINT('Ctrl Pts',(3.80703355753486,0.476284508866618,-0.0333708663946939));
#16893=CARTESIAN_POINT('Ctrl Pts',(3.81265712292028,0.473792923732884,-0.0265252924823697));
#16894=CARTESIAN_POINT('Ctrl Pts',(3.81803733335002,0.471271007296339,-0.0195963840004684));
#16895=CARTESIAN_POINT('Ctrl Pts',(3.83298840477383,0.464262851526213,-0.000341634217944583));
#16896=CARTESIAN_POINT('Ctrl Pts',(3.84610260970866,0.457005364869118,0.0195981465464975));
#16897=CARTESIAN_POINT('Ctrl Pts',(3.85774603965601,0.449598868493433,0.0399473281480481));
#16898=CARTESIAN_POINT('Ctrl Pts',(3.86822850312385,0.442930873921912,0.0582674927132378));
#16899=CARTESIAN_POINT('Ctrl Pts',(3.87751904506637,0.43614275421269,0.0769176983817686));
#16900=CARTESIAN_POINT('Ctrl Pts',(3.8858524605855,0.429301526663394,0.0957138166416987));
#16901=CARTESIAN_POINT('Ctrl Pts',(3.89358602033688,0.422952744233937,0.113156953051177));
#16902=CARTESIAN_POINT('Ctrl Pts',(3.90049500946549,0.416558315606917,0.130725501357744));
#16903=CARTESIAN_POINT('Ctrl Pts',(3.90673917358546,0.410161791821601,0.148299806064416));
#16904=CARTESIAN_POINT('Ctrl Pts',(3.91218759686158,0.404580425219352,0.163634484811763));
#16905=CARTESIAN_POINT('Ctrl Pts',(3.91712836591243,0.398998754805198,0.178969998275458));
#16906=CARTESIAN_POINT('Ctrl Pts',(3.92165664060923,0.393431214595175,0.19426668932237));
#16907=CARTESIAN_POINT('Ctrl Pts',(3.92700398270312,0.386856626232525,0.212330222435795));
#16908=CARTESIAN_POINT('Ctrl Pts',(3.93177725325759,0.380301392122174,0.230340580178059));
#16909=CARTESIAN_POINT('Ctrl Pts',(3.93610473145847,0.373771682027175,0.24828081126449));
#16910=CARTESIAN_POINT('Ctrl Pts',(3.94061484429769,0.366966395444824,0.266978182529147));
#16911=CARTESIAN_POINT('Ctrl Pts',(3.94464053769894,0.360188774116983,0.285599544131731));
#16912=CARTESIAN_POINT('Ctrl Pts',(3.94829463739126,0.353429038225082,0.304171765902933));
#16913=CARTESIAN_POINT('Ctrl Pts',(3.95132569513222,0.34782187051561,0.319577332610564));
#16914=CARTESIAN_POINT('Ctrl Pts',(3.95410037541624,0.342226650443178,0.334950073455211));
#16915=CARTESIAN_POINT('Ctrl Pts',(3.95666897647058,0.336630239649571,0.3503260857794));
#16916=CARTESIAN_POINT('Ctrl Pts',(3.95905101066503,0.33144031657685,0.364585282266353));
#16917=CARTESIAN_POINT('Ctrl Pts',(3.9612551996362,0.32624922422557,0.378847691319743));
#16918=CARTESIAN_POINT('Ctrl Pts',(3.96330637589166,0.321063603501971,0.393095067199633));
#16919=CARTESIAN_POINT('Ctrl Pts',(3.96691882338176,0.311930900976914,0.418186961229127));
#16920=CARTESIAN_POINT('Ctrl Pts',(3.97005955397289,0.302813398031445,0.443237094756921));
#16921=CARTESIAN_POINT('Ctrl Pts',(3.97284569678751,0.293717730509341,0.468227235952075));
#16922=CARTESIAN_POINT('Ctrl Pts',(3.97543099278593,0.285277749355281,0.491415893652218));
#16923=CARTESIAN_POINT('Ctrl Pts',(3.97771036641322,0.276856252186037,0.514553767021461));
#16924=CARTESIAN_POINT('Ctrl Pts',(3.97975648063729,0.268447161865253,0.537657552854712));
#16925=CARTESIAN_POINT('Ctrl Pts',(3.98161738897013,0.260799228008218,0.558670078485823));
#16926=CARTESIAN_POINT('Ctrl Pts',(3.98328556717928,0.253158069280994,0.579663989600761));
#16927=CARTESIAN_POINT('Ctrl Pts',(3.98480166079054,0.245527014801487,0.600630139523244));
#16928=CARTESIAN_POINT('Ctrl Pts',(3.98708880152943,0.234014997699602,0.632259146643622));
#16929=CARTESIAN_POINT('Ctrl Pts',(3.98903054474691,0.222528738766917,0.663817383775745));
#16930=CARTESIAN_POINT('Ctrl Pts',(3.99073668214014,0.211074767458993,0.695286911387915));
#16931=CARTESIAN_POINT('Ctrl Pts',(3.99252654604435,0.199058707155059,0.728300765828298));
#16932=CARTESIAN_POINT('Ctrl Pts',(3.99405681992494,0.187078032354012,0.761217399398529));
#16933=CARTESIAN_POINT('Ctrl Pts',(3.99542341045194,0.175123022359742,0.794063519491691));
#16934=CARTESIAN_POINT('Ctrl Pts',(3.99689014952689,0.162291907293772,0.829316718492614));
#16935=CARTESIAN_POINT('Ctrl Pts',(3.99816813525302,0.149490243752837,0.864489000093564));
#16936=CARTESIAN_POINT('Ctrl Pts',(3.99934516717317,0.136688680681622,0.899661005656283));
#16937=CARTESIAN_POINT('Ctrl Pts',(3.99956694488036,0.134276595454529,0.906288155368636));
#16938=CARTESIAN_POINT('Ctrl Pts',(3.99978506111859,0.13186447030226,0.912915414774516));
#16939=CARTESIAN_POINT('Ctrl Pts',(4.,0.129452050955556,0.919543482472952));
#16940=CARTESIAN_POINT('Ctrl Pts',(2.80364725095274,0.0799999999984753,
1.19999999979367));
#16941=CARTESIAN_POINT('Ctrl Pts',(2.81754102919364,0.0799999999984752,
1.19999900193533));
#16942=CARTESIAN_POINT('Ctrl Pts',(2.84544455850609,0.0799999999992679,
1.19257285603888));
#16943=CARTESIAN_POINT('Ctrl Pts',(2.86597664848058,0.08,1.17203236493386));
#16944=CARTESIAN_POINT('Ctrl Pts',(2.87292353761413,0.08,1.16));
#16945=CARTESIAN_POINT('Ctrl Pts',(2.80364725095274,0.0560640559714148,
1.19999999979413));
#16946=CARTESIAN_POINT('Ctrl Pts',(2.81749662686061,0.0560640559714148,
1.19999900512479));
#16947=CARTESIAN_POINT('Ctrl Pts',(2.84542227433267,0.0560640559720564,
1.19253372046443));
#16948=CARTESIAN_POINT('Ctrl Pts',(2.86599884964717,0.0560640559726492,
1.17199391138533));
#16949=CARTESIAN_POINT('Ctrl Pts',(2.87292353761413,0.0560640559726492,
1.16));
#16950=CARTESIAN_POINT('Ctrl Pts',(2.80364869399581,0.0146264256801572,
1.22009235108497));
#16951=CARTESIAN_POINT('Ctrl Pts',(2.82104450402995,0.0146264256801572,
1.22009110170889));
#16952=CARTESIAN_POINT('Ctrl Pts',(2.85594987654874,0.0146264256803497,
1.21081090750893));
#16953=CARTESIAN_POINT('Ctrl Pts',(2.88162611926498,0.0146264256805277,
1.18511138910848));
#16954=CARTESIAN_POINT('Ctrl Pts',(2.8903240242984,0.0146264256805276,1.17004617567119));
#16955=CARTESIAN_POINT('Ctrl Pts',(2.80365170727521,-4.27466544297813E-18,
1.26204804161335));
#16956=CARTESIAN_POINT('Ctrl Pts',(2.8283278847973,-1.21341104992333E-18,
1.26204626935751));
#16957=CARTESIAN_POINT('Ctrl Pts',(2.87787022921565,-1.44254953221807E-16,
1.24886602237777));
#16958=CARTESIAN_POINT('Ctrl Pts',(2.91432062943914,-1.3683229200899E-16,
1.21239421763245));
#16959=CARTESIAN_POINT('Ctrl Pts',(2.92665871822345,-1.79312001105175E-16,
1.19102402098974));
#16960=CARTESIAN_POINT('Ctrl Pts',(2.80365299659412,9.71445146547012E-17,
1.27999999958735));
#16961=CARTESIAN_POINT('Ctrl Pts',(2.8314405530759,1.0015366995025E-16,
1.27999800387066));
#16962=CARTESIAN_POINT('Ctrl Pts',(2.88724761170081,-9.28783814262485E-17,
1.26514571207777));
#16963=CARTESIAN_POINT('Ctrl Pts',(2.92831179164978,-1.37991962040859E-16,
1.22406472986772));
#16964=CARTESIAN_POINT('Ctrl Pts',(2.94220556991688,-1.80411241501588E-16,
1.2));
#16965=CARTESIAN_POINT('',(2.80365299659412,3.70074341541719E-17,1.27999999977075));
#16966=CARTESIAN_POINT('',(2.80364725095274,0.0800000000002712,1.2));
#16967=CARTESIAN_POINT('Origin',(2.80365299155732,0.0800000001034236,1.27999999989746));
#16968=CARTESIAN_POINT('',(2.87292353761412,0.08,1.16));
#16969=CARTESIAN_POINT('Origin',(2.80364150531137,0.08,1.12));
#16970=CARTESIAN_POINT('',(2.94220556991688,0.,1.2));
#16971=CARTESIAN_POINT('Origin',(2.94220556991688,0.08,1.2));
#16972=CARTESIAN_POINT('Ctrl Pts',(2.94220556991688,-1.80411241501588E-16,
1.2));
#16973=CARTESIAN_POINT('Ctrl Pts',(2.92831179164978,-1.37991962040859E-16,
1.22406472986772));
#16974=CARTESIAN_POINT('Ctrl Pts',(2.88724761170081,-9.28783814262485E-17,
1.26514571207777));
#16975=CARTESIAN_POINT('Ctrl Pts',(2.8314405530759,1.0015366995025E-16,
1.27999800387066));
#16976=CARTESIAN_POINT('Ctrl Pts',(2.80365299659412,9.71445146547012E-17,
1.27999999958735));
#16977=CARTESIAN_POINT('Ctrl Pts',(2.97150805818412,0.0370740550288554,
0.944346301619442));
#16978=CARTESIAN_POINT('Ctrl Pts',(2.96893696336745,0.0199732893870456,
1.00206772104214));
#16979=CARTESIAN_POINT('Ctrl Pts',(2.96630502643548,0.00868534462510511,
1.06150700206698));
#16980=CARTESIAN_POINT('Ctrl Pts',(2.96341860243339,0.00343337974894797,
1.12146150337824));
#16981=CARTESIAN_POINT('Ctrl Pts',(2.94780950688205,0.0373896078982158,
0.943281193781355));
#16982=CARTESIAN_POINT('Ctrl Pts',(2.94518931216128,0.0202159191784814,
1.00097915593662));
#16983=CARTESIAN_POINT('Ctrl Pts',(2.94251940811176,0.00887573436834648,
1.06032244794287));
#16984=CARTESIAN_POINT('Ctrl Pts',(2.93958582132594,0.00354285648585825,
1.12021175717441));
#16985=CARTESIAN_POINT('Ctrl Pts',(2.90676713760894,0.0568417110754077,
0.947037633415512));
#16986=CARTESIAN_POINT('Ctrl Pts',(2.90406861189144,0.0400195254220902,
1.00340948853811));
#16987=CARTESIAN_POINT('Ctrl Pts',(2.90132962478988,0.0288803134333534,
1.06138518563746));
#16988=CARTESIAN_POINT('Ctrl Pts',(2.89832135056208,0.0236236998222968,
1.11979038686856));
#16989=CARTESIAN_POINT('Ctrl Pts',(2.89185002996796,0.0967164840794545,
0.958121804096728));
#16990=CARTESIAN_POINT('Ctrl Pts',(2.88922085401446,0.0807642369419484,
1.01185984132483));
#16991=CARTESIAN_POINT('Ctrl Pts',(2.88654630615169,0.0702230541962401,
1.06707171515406));
#16992=CARTESIAN_POINT('Ctrl Pts',(2.88361236102833,0.0652969522996504,
1.1226636989333));
#16993=CARTESIAN_POINT('Ctrl Pts',(2.89160349189832,0.113778583470735,0.963164633118633));
#16994=CARTESIAN_POINT('Ctrl Pts',(2.88903135432334,0.0981978858859783,
1.01577658887176));
#16995=CARTESIAN_POINT('Ctrl Pts',(2.88640501551798,0.0879133139917624,
1.06981306289243));
#16996=CARTESIAN_POINT('Ctrl Pts',(2.8835300538724,0.0831281904379304,1.12422135153853));
#16997=CARTESIAN_POINT('',(2.96341860243339,0.00343337974894797,1.12146150337824));
#16998=CARTESIAN_POINT('',(2.88353005387238,0.0831281904379304,1.12422135153898));
#16999=CARTESIAN_POINT('Origin',(2.96341860243339,0.0831281904379304,1.12844270307795));
#17000=CARTESIAN_POINT('',(2.89160351335905,0.11377873136113,0.96316419414885));
#17001=CARTESIAN_POINT('Ctrl Pts',(2.8835300538724,0.0831281904379304,1.12422135153853));
#17002=CARTESIAN_POINT('Ctrl Pts',(2.88640501551798,0.0879133139917624,
1.06981306289243));
#17003=CARTESIAN_POINT('Ctrl Pts',(2.88903135432334,0.0981978858859783,
1.01577658887176));
#17004=CARTESIAN_POINT('Ctrl Pts',(2.89160349189832,0.113778583470735,0.963164633118633));
#17005=CARTESIAN_POINT('',(2.97150807857098,0.0370741994904978,0.944345814008723));
#17006=CARTESIAN_POINT('Origin',(2.97150805818412,0.113778583470735,0.967071074808825));
#17007=CARTESIAN_POINT('Ctrl Pts',(2.97150805818412,0.0370740550288554,
0.944346301619442));
#17008=CARTESIAN_POINT('Ctrl Pts',(2.96893696336745,0.0199732893870456,
1.00206772104214));
#17009=CARTESIAN_POINT('Ctrl Pts',(2.96630502643548,0.00868534462510511,
1.06150700206698));
#17010=CARTESIAN_POINT('Ctrl Pts',(2.96341860243339,0.00343337974894797,
1.12146150337824));
#17011=CARTESIAN_POINT('Ctrl Pts',(2.89160353535339,0.113778846700823,0.963163744264181));
#17012=CARTESIAN_POINT('Ctrl Pts',(2.89200309459449,0.115874999468036,0.954990934520135));
#17013=CARTESIAN_POINT('Ctrl Pts',(2.89105241294694,0.118516767083136,0.946926805316735));
#17014=CARTESIAN_POINT('Ctrl Pts',(2.8887998347044,0.12151892108873,0.939367876351702));
#17015=CARTESIAN_POINT('Ctrl Pts',(2.89193225405221,0.091029389236732,0.956439946820171));
#17016=CARTESIAN_POINT('Ctrl Pts',(2.89244979273278,0.0933382871392351,
0.947816425216694));
#17017=CARTESIAN_POINT('Ctrl Pts',(2.89143805103303,0.0961424440727286,
0.939168089922756));
#17018=CARTESIAN_POINT('Ctrl Pts',(2.88899324581141,0.0991663031639316,
0.931175208977201));
#17019=CARTESIAN_POINT('Ctrl Pts',(2.91219550748833,0.0516302792459275,
0.945758016401462));
#17020=CARTESIAN_POINT('Ctrl Pts',(2.91287652263897,0.0549833683958626,
0.934311081329529));
#17021=CARTESIAN_POINT('Ctrl Pts',(2.91159668209949,0.0586720092836598,
0.922844854319782));
#17022=CARTESIAN_POINT('Ctrl Pts',(2.90847135897849,0.0624299397708595,
0.91206627137828));
#17023=CARTESIAN_POINT('Ctrl Pts',(2.95373418875325,0.0373110094222872,
0.943546496072754));
#17024=CARTESIAN_POINT('Ctrl Pts',(2.95449085000615,0.0420466727985156,
0.927625463037334));
#17025=CARTESIAN_POINT('Ctrl Pts',(2.95277547249147,0.0472656493538997,
0.911724687618538));
#17026=CARTESIAN_POINT('Ctrl Pts',(2.94868907631857,0.0526474168866845,
0.89665812635227));
#17027=CARTESIAN_POINT('Ctrl Pts',(2.97150810162045,0.0370743439314857,
0.944345326468057));
#17028=CARTESIAN_POINT('Ctrl Pts',(2.97229749829158,0.0423247695708639,
0.926623268322567));
#17029=CARTESIAN_POINT('Ctrl Pts',(2.97039533243128,0.0481773468294725,
0.90893953762639));
#17030=CARTESIAN_POINT('Ctrl Pts',(2.96589752617094,0.0542766837559666,
0.892181754340009));
#17031=CARTESIAN_POINT('',(2.88879983479628,0.121518920962533,0.939367876658545));
#17032=CARTESIAN_POINT('',(2.96589753208429,0.0542766627970602,0.892181811924114));
#17033=CARTESIAN_POINT('Origin',(2.96589752635434,0.129452089417722,0.919543376799038));
#17034=CARTESIAN_POINT('Ctrl Pts',(2.96589754105586,0.0542766635709679,
0.892181809797819));
#17035=CARTESIAN_POINT('Ctrl Pts',(2.97039533662793,0.0481773339172204,
0.908939576641134));
#17036=CARTESIAN_POINT('Ctrl Pts',(2.97229749742078,0.0423247637789863,
0.926623287872219));
#17037=CARTESIAN_POINT('Ctrl Pts',(2.97150810162045,0.0370743439314857,
0.944345326468057));
#17038=CARTESIAN_POINT('Ctrl Pts',(2.89160353535339,0.113778846700823,0.963163744264181));
#17039=CARTESIAN_POINT('Ctrl Pts',(2.89200309458905,0.115874999439544,0.954990934631221));
#17040=CARTESIAN_POINT('Ctrl Pts',(2.89105241297279,0.118516767011321,0.946926805535954));
#17041=CARTESIAN_POINT('Ctrl Pts',(2.88879983479625,0.121518920966312,0.93936787665993));
#17042=CARTESIAN_POINT('Ctrl Pts',(2.87292353761413,0.08,1.16));
#17043=CARTESIAN_POINT('Ctrl Pts',(2.87920815162899,0.0800000000000001,
1.14911472922029));
#17044=CARTESIAN_POINT('Ctrl Pts',(2.88286933791013,0.0809375160872416,
1.13672531827616));
#17045=CARTESIAN_POINT('Ctrl Pts',(2.88353005387235,0.0831281904378509,
1.12422135153943));
#17046=CARTESIAN_POINT('Ctrl Pts',(2.87292353761413,0.0560640559726493,
1.16));
#17047=CARTESIAN_POINT('Ctrl Pts',(2.87947165153049,0.0562707216725976,
1.14867500509237));
#17048=CARTESIAN_POINT('Ctrl Pts',(2.88327482610756,0.057283711013126,1.1353889478833));
#17049=CARTESIAN_POINT('Ctrl Pts',(2.88363979674692,0.0593532062534744,
1.12214448139916));
#17050=CARTESIAN_POINT('Ctrl Pts',(2.89032400439417,0.0146263981036585,
1.17004616417948));
#17051=CARTESIAN_POINT('Ctrl Pts',(2.89862998177407,0.015162040564682,1.15493509506255));
#17052=CARTESIAN_POINT('Ctrl Pts',(2.90339459648587,0.0163044774309504,
1.13733803743769));
#17053=CARTESIAN_POINT('Ctrl Pts',(2.90376961212187,0.0181889922805759,
1.11960219988233));
#17054=CARTESIAN_POINT('Ctrl Pts',(2.92665871822345,1.04444016743217E-16,
1.19102402098974));
#17055=CARTESIAN_POINT('Ctrl Pts',(2.93795081424088,0.000240558124196419,
1.16964064866978));
#17056=CARTESIAN_POINT('Ctrl Pts',(2.94450524794608,0.00132703835077383,
1.14520540513807));
#17057=CARTESIAN_POINT('Ctrl Pts',(2.94554401660275,0.0035154873015423,
1.12052419372636));
#17058=CARTESIAN_POINT('Ctrl Pts',(2.94220556991688,5.55111512312578E-17,
1.2));
#17059=CARTESIAN_POINT('Ctrl Pts',(2.95477479794662,1.89492314713005E-16,
1.17610550316648));
#17060=CARTESIAN_POINT('Ctrl Pts',(2.96209717050889,0.00102898107136256,
1.14890923524034));
#17061=CARTESIAN_POINT('Ctrl Pts',(2.96341860243333,0.00343337974886057,
1.12146150337924));
#17062=CARTESIAN_POINT('Ctrl Pts',(2.96341860243333,0.00343337974886057,
1.12146150337924));
#17063=CARTESIAN_POINT('Ctrl Pts',(2.96209717050889,0.00102898107136256,
1.14890923524034));
#17064=CARTESIAN_POINT('Ctrl Pts',(2.95477479794662,1.89492314713005E-16,
1.17610550316648));
#17065=CARTESIAN_POINT('Ctrl Pts',(2.94220556991688,5.55111512312578E-17,
1.2));
#17066=CARTESIAN_POINT('Ctrl Pts',(2.8729150760721,0.08,1.1599951409471));
#17067=CARTESIAN_POINT('Ctrl Pts',(2.87917356064383,0.0800000000000001,
1.14909663226456));
#17068=CARTESIAN_POINT('Ctrl Pts',(2.88286933791013,0.0809375160872416,
1.13672531827616));
#17069=CARTESIAN_POINT('Ctrl Pts',(2.88353005387235,0.0831281904378509,
1.12422135153943));
#17070=CARTESIAN_POINT('Ctrl Pts',(2.88879983479625,0.121518920966305,0.939367876659928));
#17071=CARTESIAN_POINT('Ctrl Pts',(2.8880324319677,0.122541686734965,0.936792718960852));
#17072=CARTESIAN_POINT('Ctrl Pts',(2.8871159230781,0.123551627030471,0.934256686681854));
#17073=CARTESIAN_POINT('Ctrl Pts',(2.88605564938321,0.124542858554496,0.931774551486074));
#17074=CARTESIAN_POINT('Ctrl Pts',(2.88899324674614,0.0991663025264055,
0.931175212345719));
#17075=CARTESIAN_POINT('Ctrl Pts',(2.88820270097191,0.100171613150583,0.928602454646129));
#17076=CARTESIAN_POINT('Ctrl Pts',(2.887256914194,0.101172190427294,0.926046640793733));
#17077=CARTESIAN_POINT('Ctrl Pts',(2.88617479048184,0.102143858159124,0.923571684284616));
#17078=CARTESIAN_POINT('Ctrl Pts',(2.90847130245117,0.0624298642422617,
0.91206627056425));
#17079=CARTESIAN_POINT('Ctrl Pts',(2.90747172794183,0.0636341682311426,
0.908814316971422));
#17080=CARTESIAN_POINT('Ctrl Pts',(2.90628712830328,0.0648169887234241,
0.905621914364158));
#17081=CARTESIAN_POINT('Ctrl Pts',(2.90492140034315,0.0659768590565696,
0.902493719598966));
#17082=CARTESIAN_POINT('Ctrl Pts',(2.94868907688287,0.0526474135734431,
0.89665813737666));
#17083=CARTESIAN_POINT('Ctrl Pts',(2.94731633955782,0.0543286937237626,
0.892038265656662));
#17084=CARTESIAN_POINT('Ctrl Pts',(2.94567970499161,0.0559838108192925,
0.887492074720039));
#17085=CARTESIAN_POINT('Ctrl Pts',(2.9437870193114,0.0576045375805993,0.883038551101561));
#17086=CARTESIAN_POINT('Ctrl Pts',(2.96589752635434,0.054276679754843,0.892181765332982));
#17087=CARTESIAN_POINT('Ctrl Pts',(2.96436522474194,0.0561698833733057,
0.886980231140826));
#17088=CARTESIAN_POINT('Ctrl Pts',(2.96253475240426,0.0580349143566106,
0.881856100627612));
#17089=CARTESIAN_POINT('Ctrl Pts',(2.96041677700223,0.059860909263175,0.876839220853787));
#17090=CARTESIAN_POINT('',(2.88605571002765,0.124542801858886,0.931774693457122));
#17091=CARTESIAN_POINT('Origin',(2.96041689814401,0.135036214484351,0.904201119271044));
#17092=CARTESIAN_POINT('Origin',(2.81153837945173,0.0396614298686474,0.932336834374758));
#17093=CARTESIAN_POINT('Origin',(2.83103982275571,0.116960654826865,0.953478215069898));
#17094=CARTESIAN_POINT('Origin',(2.96041689814401,0.135036214484351,0.904201119271044));
#17095=CARTESIAN_POINT('Origin',(2.96041689814401,0.135036214484351,0.904201119271044));
#17096=CARTESIAN_POINT('Origin',(3.43968169690401,0.263987455675949,0.316006143873433));
#17097=CARTESIAN_POINT('',(-4.5,0.0542766412926824,0.892181871006898));
#17098=CARTESIAN_POINT('Ctrl Pts',(4.,0.0542766412926824,0.892181871006898));
#17099=CARTESIAN_POINT('Ctrl Pts',(4.,0.618092213764235,1.0973939570023));
#17100=CARTESIAN_POINT('Ctrl Pts',(3.99999413894399,0.0543424242950403,
0.892001133693336));
#17101=CARTESIAN_POINT('Ctrl Pts',(3.99999413894399,0.618157996766593,1.09721321968874));
#17102=CARTESIAN_POINT('Ctrl Pts',(3.99855414331412,0.0704990924696518,
0.84761105270997));
#17103=CARTESIAN_POINT('Ctrl Pts',(3.99855414331412,0.634314664941205,1.05282313870537));
#17104=CARTESIAN_POINT('Ctrl Pts',(3.99545186687381,0.102617065619348,0.759367646722529));
#17105=CARTESIAN_POINT('Ctrl Pts',(3.99545186687381,0.666432638090901,0.96457973271793));
#17106=CARTESIAN_POINT('Ctrl Pts',(3.98977740850449,0.150154761706454,0.628758900150308));
#17107=CARTESIAN_POINT('Ctrl Pts',(3.98977740850449,0.713970334178007,0.833970986145709));
#17108=CARTESIAN_POINT('Ctrl Pts',(3.97841403016118,0.21121967143493,0.460984439550287));
#17109=CARTESIAN_POINT('Ctrl Pts',(3.97841403016118,0.775035243906483,0.666196525545688));
#17110=CARTESIAN_POINT('Ctrl Pts',(3.95259200169988,0.280544576017307,0.270515829604361));
#17111=CARTESIAN_POINT('Ctrl Pts',(3.95259200169988,0.84436014848886,0.475727915599762));
#17112=CARTESIAN_POINT('Ctrl Pts',(3.90986572419832,0.340085651878976,0.10692806814439));
#17113=CARTESIAN_POINT('Ctrl Pts',(3.90986572419832,0.903901224350529,0.312140154139791));
#17114=CARTESIAN_POINT('Ctrl Pts',(3.84598208672298,0.387862727674237,-0.024338368770661));
#17115=CARTESIAN_POINT('Ctrl Pts',(3.84598208672298,0.95167830014579,0.18087371722474));
#17116=CARTESIAN_POINT('Ctrl Pts',(3.75872318140661,0.423488332610525,-0.122218913887524));
#17117=CARTESIAN_POINT('Ctrl Pts',(3.75872318140661,0.987303905082078,0.0829931721078771));
#17118=CARTESIAN_POINT('Ctrl Pts',(3.64881642260075,0.448607387242674,-0.1912329492874));
#17119=CARTESIAN_POINT('Ctrl Pts',(3.64881642260075,1.01242295971423,0.0139791367080011));
#17120=CARTESIAN_POINT('Ctrl Pts',(3.52045328348988,0.465105650196583,-0.236561554213491));
#17121=CARTESIAN_POINT('Ctrl Pts',(3.52045328348988,1.02892122266814,-0.0313494682180899));
#17122=CARTESIAN_POINT('Ctrl Pts',(3.3816469894381,0.473698270059216,-0.260169583260034));
#17123=CARTESIAN_POINT('Ctrl Pts',(3.3816469894381,1.03751384253077,-0.0549574972646329));
#17124=CARTESIAN_POINT('Ctrl Pts',(3.2451100102617,0.472026186036982,-0.255575570165513));
#17125=CARTESIAN_POINT('Ctrl Pts',(3.2451100102617,1.03584175850854,-0.0503634841701119));
#17126=CARTESIAN_POINT('Ctrl Pts',(3.12452733970665,0.456428987719484,-0.212722619981431));
#17127=CARTESIAN_POINT('Ctrl Pts',(3.12452733970665,1.02024456019104,-0.00751053398602988));
#17128=CARTESIAN_POINT('Ctrl Pts',(3.03063129752059,0.423994474883979,-0.12360952835487));
#17129=CARTESIAN_POINT('Ctrl Pts',(3.03063129752059,0.987810047355532,0.0816025576405311));
#17130=CARTESIAN_POINT('Ctrl Pts',(2.96639254265844,0.374982215648855,0.0110505471700891));
#17131=CARTESIAN_POINT('Ctrl Pts',(2.96639254265844,0.938797788120408,0.21626263316549));
#17132=CARTESIAN_POINT('Ctrl Pts',(2.92780415844446,0.3125142105656,0.182679980574709));
#17133=CARTESIAN_POINT('Ctrl Pts',(2.92780415844446,0.876329783037153,0.38789206657011));
#17134=CARTESIAN_POINT('Ctrl Pts',(2.90717911786689,0.241012720183584,0.379128710856649));
#17135=CARTESIAN_POINT('Ctrl Pts',(2.90717911786689,0.804828292655137,0.58434079685205));
#17136=CARTESIAN_POINT('Ctrl Pts',(2.89676647174986,0.173526397310964,0.564545859071197));
#17137=CARTESIAN_POINT('Ctrl Pts',(2.89676647174986,0.737341969782517,0.769757945066598));
#17138=CARTESIAN_POINT('Ctrl Pts',(2.88965455295895,0.120639229722747,0.709852157798736));
#17139=CARTESIAN_POINT('Ctrl Pts',(2.88965455295895,0.6844548021943,0.915064243794137));
#17140=CARTESIAN_POINT('Ctrl Pts',(2.88410012960048,0.0831761921549105,
0.812781007580546));
#17141=CARTESIAN_POINT('Ctrl Pts',(2.88410012960048,0.646991764626463,1.01799309357595));
#17142=CARTESIAN_POINT('Ctrl Pts',(2.88050601962429,0.0610892789569565,
0.873464302857379));
#17143=CARTESIAN_POINT('Ctrl Pts',(2.88050601962429,0.624904851428509,1.07867638885278));
#17144=CARTESIAN_POINT('Ctrl Pts',(2.87936339380802,0.0542766412926821,
0.892181871006899));
#17145=CARTESIAN_POINT('Ctrl Pts',(2.87936339380802,0.618092213764235,1.0973939570023));
#17146=CARTESIAN_POINT('',(2.88019546786692,0.529127141944176,1.04944304294295));
#17147=CARTESIAN_POINT('Ctrl Pts',(2.88019546787498,0.529127141999364,1.04944304281375));
#17148=CARTESIAN_POINT('Ctrl Pts',(2.88033620447493,0.398430560163569,0.999217108032501));
#17149=CARTESIAN_POINT('Ctrl Pts',(2.88044239084245,0.267517984580123,0.949554742349327));
#17150=CARTESIAN_POINT('Ctrl Pts',(2.88054197312457,0.13656563129969,0.899999067707368));
#17151=CARTESIAN_POINT('Ctrl Pts',(4.,0.524122951685637,1.06319194266973));
#17152=CARTESIAN_POINT('Ctrl Pts',(3.99999413894399,0.524188734687995,1.06301120535617));
#17153=CARTESIAN_POINT('Ctrl Pts',(3.99855414331412,0.540345402862606,1.0186211243728));
#17154=CARTESIAN_POINT('Ctrl Pts',(3.99545186687381,0.572463376012303,0.930377718385363));
#17155=CARTESIAN_POINT('Ctrl Pts',(3.98977740850449,0.620001072099409,0.799768971813143));
#17156=CARTESIAN_POINT('Ctrl Pts',(3.97841403016118,0.681065981827884,0.631994511213121));
#17157=CARTESIAN_POINT('Ctrl Pts',(3.95259200169988,0.750390886410261,0.441525901267195));
#17158=CARTESIAN_POINT('Ctrl Pts',(3.90986572419832,0.80993196227193,0.277938139807224));
#17159=CARTESIAN_POINT('Ctrl Pts',(3.84598208672298,0.857709038067191,0.146671702892173));
#17160=CARTESIAN_POINT('Ctrl Pts',(3.75872318140661,0.893334643003479,0.0487911577753098));
#17161=CARTESIAN_POINT('Ctrl Pts',(3.64881642260075,0.918453697635628,-0.0202228776245657));
#17162=CARTESIAN_POINT('Ctrl Pts',(3.52045328348988,0.934951960589537,-0.0655514825506567));
#17163=CARTESIAN_POINT('Ctrl Pts',(3.3816469894381,0.943544580452171,-0.0891595115971992));
#17164=CARTESIAN_POINT('Ctrl Pts',(3.2451100102617,0.941872496429936,-0.0845654985026787));
#17165=CARTESIAN_POINT('Ctrl Pts',(3.12452733970665,0.926275298112438,-0.041712548318597));
#17166=CARTESIAN_POINT('Ctrl Pts',(3.03063129752059,0.893840785276933,0.0474005433079645));
#17167=CARTESIAN_POINT('Ctrl Pts',(2.96639254265844,0.844828526041809,0.182060618832923));
#17168=CARTESIAN_POINT('Ctrl Pts',(2.92780415844446,0.782360520958554,0.353690052237544));
#17169=CARTESIAN_POINT('Ctrl Pts',(2.90717911786689,0.710859030576538,0.550138782519483));
#17170=CARTESIAN_POINT('Ctrl Pts',(2.89692008845523,0.644368326537099,0.732820490471484));
#17171=CARTESIAN_POINT('Ctrl Pts',(2.88992562590405,0.59249855766718,0.875331509193915));
#17172=CARTESIAN_POINT('Ctrl Pts',(2.88454584060419,0.556036094594039,0.975511303145068));
#17173=CARTESIAN_POINT('Ctrl Pts',(2.88115416462358,0.534942607774809,1.03346518187847));
#17174=CARTESIAN_POINT('Ctrl Pts',(2.88019546785078,0.529127141844543,1.04944304320548));
#17175=CARTESIAN_POINT('Ctrl Pts',(2.88605571006501,0.12454279754309,0.931774691915435));
#17176=CARTESIAN_POINT('Ctrl Pts',(2.88491303328969,0.256571286428345,0.978937914242353));
#17177=CARTESIAN_POINT('Ctrl Pts',(2.88378009846091,0.388637587381446,1.02596265267948));
#17178=CARTESIAN_POINT('Ctrl Pts',(2.8826071904062,0.520860744120384,1.07251108028126));
#17179=CARTESIAN_POINT('Ctrl Pts',(2.88179136985247,0.128344716275584,0.921721359700738));
#17180=CARTESIAN_POINT('Ctrl Pts',(2.88137748969615,0.260125811446042,0.969562560736564));
#17181=CARTESIAN_POINT('Ctrl Pts',(2.88096557603236,0.391911191572128,1.01736709873619));
#17182=CARTESIAN_POINT('Ctrl Pts',(2.88054812086471,0.523720986413769,1.06506475118311));
#17183=CARTESIAN_POINT('Ctrl Pts',(2.87989567979058,0.132478313274208,0.910796512238404));
#17184=CARTESIAN_POINT('Ctrl Pts',(2.8798498458325,0.263928703639433,0.959537410055039));
#17185=CARTESIAN_POINT('Ctrl Pts',(2.87979494426834,0.39536106646766,1.00831406088685));
#17186=CARTESIAN_POINT('Ctrl Pts',(2.87973121518385,0.526696991648902,1.05732078078704));
#17187=CARTESIAN_POINT('Ctrl Pts',(2.88054197312457,0.13656563129969,0.899999067707368));
#17188=CARTESIAN_POINT('Ctrl Pts',(2.88044225836535,0.267692194169797,0.949620667653677));
#17189=CARTESIAN_POINT('Ctrl Pts',(2.88033592193784,0.398778873437746,0.999349242698191));
#17190=CARTESIAN_POINT('Ctrl Pts',(2.88019490601393,0.529648748841403,1.04964349671765));
#17191=CARTESIAN_POINT('',(2.88260719040209,0.52086074410776,1.07251108032045));
#17192=CARTESIAN_POINT('Ctrl Pts',(2.88605571002765,0.124542801858885,0.931774693457124));
#17193=CARTESIAN_POINT('Ctrl Pts',(2.884913033265,0.256571289306366,0.978937915267128));
#17194=CARTESIAN_POINT('Ctrl Pts',(2.88378009844813,0.388637588822166,1.02596265318668));
#17195=CARTESIAN_POINT('Ctrl Pts',(2.8826071904062,0.520860744120384,1.07251108028126));
#17196=CARTESIAN_POINT('',(2.88071362092342,0.524122953967611,1.06319194136119));
#17197=CARTESIAN_POINT('Origin',(2.95737828760701,0.541322246857939,1.05905796302752));
#17198=CARTESIAN_POINT('Ctrl Pts',(2.88071362118334,0.524122952384465,1.06319194074971));
#17199=CARTESIAN_POINT('Ctrl Pts',(2.88040468271156,0.524951973935425,1.06091422275821));
#17200=CARTESIAN_POINT('Ctrl Pts',(2.88020636536677,0.525785827271151,1.05862322954717));
#17201=CARTESIAN_POINT('Ctrl Pts',(2.88003298245609,0.527456219186867,1.0540338654771));
#17202=CARTESIAN_POINT('Ctrl Pts',(2.88005791438801,0.528292751084348,1.05173551297811));
#17203=CARTESIAN_POINT('Ctrl Pts',(2.88019546787499,0.529127141988623,1.04944304280962));
#17204=CARTESIAN_POINT('Ctrl Pts',(2.88602210209193,0.123730872767436,0.931375362419385));
#17205=CARTESIAN_POINT('Ctrl Pts',(2.88489031580204,0.256137405346913,0.978701308463558));
#17206=CARTESIAN_POINT('Ctrl Pts',(2.88377139476759,0.388593451583146,1.0259100078282));
#17207=CARTESIAN_POINT('Ctrl Pts',(2.8826044419187,0.521173013031435,1.07262110155611));
#17208=CARTESIAN_POINT('Ctrl Pts',(2.89021809451686,0.120434537356878,0.941383776987583));
#17209=CARTESIAN_POINT('Ctrl Pts',(2.88835152335579,0.253090597695893,0.9880121068955));
#17210=CARTESIAN_POINT('Ctrl Pts',(2.88651642325475,0.385832990043375,1.03444765358277));
#17211=CARTESIAN_POINT('Ctrl Pts',(2.8846060092736,0.518831485782303,1.08003438801855));
#17212=CARTESIAN_POINT('Ctrl Pts',(2.89213808672452,0.116817760728715,0.952233907678371));
#17213=CARTESIAN_POINT('Ctrl Pts',(2.88989822816684,0.249806253739155,0.997944196331249));
#17214=CARTESIAN_POINT('Ctrl Pts',(2.88769856407366,0.382904634727536,1.04342082167946));
#17215=CARTESIAN_POINT('Ctrl Pts',(2.88542850388851,0.516380034734364,1.08773011616922));
#17216=CARTESIAN_POINT('Ctrl Pts',(2.89161299367911,0.113199040068761,0.962970280062921));
#17217=CARTESIAN_POINT('Ctrl Pts',(2.88942220836743,0.246520922365427,1.00778095469082));
#17218=CARTESIAN_POINT('Ctrl Pts',(2.88725277180458,0.379975622201312,1.05231434239752));
#17219=CARTESIAN_POINT('Ctrl Pts',(2.885035153377,0.513928253868178,1.09536424252732));
#17220=CARTESIAN_POINT('',(2.88503519983007,0.513928543448632,1.09536334085845));
#17221=CARTESIAN_POINT('Ctrl Pts',(2.89160353474128,0.113778879042689,0.963163755874196));
#17222=CARTESIAN_POINT('Ctrl Pts',(2.88941597895361,0.246907970065613,1.00790881681038));
#17223=CARTESIAN_POINT('Ctrl Pts',(2.88724961188406,0.380170018768777,1.0523756565061));
#17224=CARTESIAN_POINT('Ctrl Pts',(2.88503519983007,0.513928543448632,1.09536334085845));
#17225=CARTESIAN_POINT('Ctrl Pts',(2.88503519983007,0.513928543448631,1.09536334085845));
#17226=CARTESIAN_POINT('Ctrl Pts',(2.88532122676486,0.515433447174265,1.08981078998296));
#17227=CARTESIAN_POINT('Ctrl Pts',(2.88498244688731,0.517061672225632,1.0842825322267));
#17228=CARTESIAN_POINT('Ctrl Pts',(2.88402831182171,0.518781812731824,1.07886904595466));
#17229=CARTESIAN_POINT('Ctrl Pts',(2.88365018585186,0.519463508458812,1.07672366861689));
#17230=CARTESIAN_POINT('Ctrl Pts',(2.88317616630465,0.520157484227229,1.07460257154214));
#17231=CARTESIAN_POINT('Ctrl Pts',(2.88260719039372,0.520860744100385,1.07251108040514));
#17232=CARTESIAN_POINT('Ctrl Pts',(4.,-0.208000000000001,1.2));
#17233=CARTESIAN_POINT('Ctrl Pts',(4.,0.670547542022765,1.2));
#17234=CARTESIAN_POINT('Ctrl Pts',(3.99999413894399,-0.208000000000001,
1.19980766336825));
#17235=CARTESIAN_POINT('Ctrl Pts',(3.99999413894399,0.670547542022765,1.19980766336825));
#17236=CARTESIAN_POINT('Ctrl Pts',(3.99855414331412,-0.208000000000001,
1.15256872586735));
#17237=CARTESIAN_POINT('Ctrl Pts',(3.99855414331412,0.670547542022765,1.15256872586735));
#17238=CARTESIAN_POINT('Ctrl Pts',(3.99545186687381,-0.208000000000001,
1.05866205464794));
#17239=CARTESIAN_POINT('Ctrl Pts',(3.99545186687381,0.670547542022765,1.05866205464794));
#17240=CARTESIAN_POINT('Ctrl Pts',(3.98977740850449,-0.208000000000001,
0.919671129654847));
#17241=CARTESIAN_POINT('Ctrl Pts',(3.98977740850449,0.670547542022765,0.919671129654847));
#17242=CARTESIAN_POINT('Ctrl Pts',(3.97841403016118,-0.208000000000001,
0.741129277895168));
#17243=CARTESIAN_POINT('Ctrl Pts',(3.97841403016118,0.670547542022765,0.741129277895168));
#17244=CARTESIAN_POINT('Ctrl Pts',(3.95259200169988,-0.208000000000001,
0.538436816836329));
#17245=CARTESIAN_POINT('Ctrl Pts',(3.95259200169988,0.670547542022765,0.538436816836329));
#17246=CARTESIAN_POINT('Ctrl Pts',(3.90986572419832,-0.208000000000001,
0.364350357241537));
#17247=CARTESIAN_POINT('Ctrl Pts',(3.90986572419832,0.670547542022765,0.364350357241537));
#17248=CARTESIAN_POINT('Ctrl Pts',(3.84598208672298,-0.208000000000001,
0.224659532804428));
#17249=CARTESIAN_POINT('Ctrl Pts',(3.84598208672298,0.670547542022765,0.224659532804428));
#17250=CARTESIAN_POINT('Ctrl Pts',(3.75872318140661,-0.208000000000001,
0.120497232333236));
#17251=CARTESIAN_POINT('Ctrl Pts',(3.75872318140661,0.670547542022765,0.120497232333236));
#17252=CARTESIAN_POINT('Ctrl Pts',(3.64881642260075,-0.208000000000001,
0.0470540298718229));
#17253=CARTESIAN_POINT('Ctrl Pts',(3.64881642260075,0.670547542022765,0.0470540298718229));
#17254=CARTESIAN_POINT('Ctrl Pts',(3.52045328348988,-0.208000000000001,
-0.00118366394786523));
#17255=CARTESIAN_POINT('Ctrl Pts',(3.52045328348988,0.670547542022765,-0.00118366394786523));
#17256=CARTESIAN_POINT('Ctrl Pts',(3.3816469894381,-0.208000000000001,-0.0263068037111615));
#17257=CARTESIAN_POINT('Ctrl Pts',(3.3816469894381,0.670547542022765,-0.0263068037111615));
#17258=CARTESIAN_POINT('Ctrl Pts',(3.2451100102617,-0.208000000000001,-0.0214179570895094));
#17259=CARTESIAN_POINT('Ctrl Pts',(3.2451100102617,0.670547542022765,-0.0214179570895094));
#17260=CARTESIAN_POINT('Ctrl Pts',(3.12452733970665,-0.208000000000001,
0.0241851999814078));
#17261=CARTESIAN_POINT('Ctrl Pts',(3.12452733970665,0.670547542022765,0.0241851999814078));
#17262=CARTESIAN_POINT('Ctrl Pts',(3.03063129752059,-0.208000000000001,
0.119017371327004));
#17263=CARTESIAN_POINT('Ctrl Pts',(3.03063129752059,0.670547542022765,0.119017371327004));
#17264=CARTESIAN_POINT('Ctrl Pts',(2.96639254265844,-0.208000000000001,
0.262319630540593));
#17265=CARTESIAN_POINT('Ctrl Pts',(2.96639254265844,0.670547542022765,0.262319630540593));
#17266=CARTESIAN_POINT('Ctrl Pts',(2.92780415844446,-0.208000000000001,
0.444963858672424));
#17267=CARTESIAN_POINT('Ctrl Pts',(2.92780415844446,0.670547542022765,0.444963858672424));
#17268=CARTESIAN_POINT('Ctrl Pts',(2.90717911786689,-0.208000000000001,
0.65402023086958));
#17269=CARTESIAN_POINT('Ctrl Pts',(2.90717911786689,0.670547542022765,0.65402023086958));
#17270=CARTESIAN_POINT('Ctrl Pts',(2.89547076625581,-0.208000000000001,
0.875890304828918));
#17271=CARTESIAN_POINT('Ctrl Pts',(2.89547076625581,0.670547542022765,0.875890304828918));
#17272=CARTESIAN_POINT('Ctrl Pts',(2.88537704766906,-0.208000000000001,
1.10060381648398));
#17273=CARTESIAN_POINT('Ctrl Pts',(2.88537704766906,0.670547542022765,1.10060381648398));
#17274=CARTESIAN_POINT('Ctrl Pts',(2.8728456296504,-0.208000000000001,1.32371934078733));
#17275=CARTESIAN_POINT('Ctrl Pts',(2.8728456296504,0.670547542022765,1.32371934078733));
#17276=CARTESIAN_POINT('Ctrl Pts',(2.85578261679345,-0.208000000000001,
1.54401727992264));
#17277=CARTESIAN_POINT('Ctrl Pts',(2.85578261679345,0.670547542022765,1.54401727992264));
#17278=CARTESIAN_POINT('Ctrl Pts',(2.83335686249019,-0.208000000000001,
1.76209503442146));
#17279=CARTESIAN_POINT('Ctrl Pts',(2.83335686249019,0.670547542022765,1.76209503442146));
#17280=CARTESIAN_POINT('Ctrl Pts',(2.80505146480345,-0.208000000000001,
1.97856787413951));
#17281=CARTESIAN_POINT('Ctrl Pts',(2.80505146480345,0.670547542022765,1.97856787413951));
#17282=CARTESIAN_POINT('Ctrl Pts',(2.76985908233915,-0.208000000000001,
2.19251877196071));
#17283=CARTESIAN_POINT('Ctrl Pts',(2.76985908233915,0.670547542022765,2.19251877196071));
#17284=CARTESIAN_POINT('Ctrl Pts',(2.72531955636536,-0.208000000000001,
2.39962532458029));
#17285=CARTESIAN_POINT('Ctrl Pts',(2.72531955636536,0.670547542022765,2.39962532458029));
#17286=CARTESIAN_POINT('Ctrl Pts',(2.66797634363184,-0.208000000000001,
2.59347738935741));
#17287=CARTESIAN_POINT('Ctrl Pts',(2.66797634363184,0.670547542022765,2.59347738935741));
#17288=CARTESIAN_POINT('Ctrl Pts',(2.59397540849171,-0.208000000000001,
2.7672283971178));
#17289=CARTESIAN_POINT('Ctrl Pts',(2.59397540849171,0.670547542022765,2.7672283971178));
#17290=CARTESIAN_POINT('Ctrl Pts',(2.49960870420485,-0.208000000000001,
2.91510580081997));
#17291=CARTESIAN_POINT('Ctrl Pts',(2.49960870420485,0.670547542022765,2.91510580081997));
#17292=CARTESIAN_POINT('Ctrl Pts',(2.38189256086504,-0.208000000000001,
3.03403241435618));
#17293=CARTESIAN_POINT('Ctrl Pts',(2.38189256086504,0.670547542022765,3.03403241435618));
#17294=CARTESIAN_POINT('Ctrl Pts',(2.23909845280558,-0.208000000000001,
3.12505646843308));
#17295=CARTESIAN_POINT('Ctrl Pts',(2.23909845280558,0.670547542022765,3.12505646843308));
#17296=CARTESIAN_POINT('Ctrl Pts',(2.07061055216582,-0.208000000000001,
3.19196918412265));
#17297=CARTESIAN_POINT('Ctrl Pts',(2.07061055216582,0.670547542022765,3.19196918412265));
#17298=CARTESIAN_POINT('Ctrl Pts',(1.87681490437036,-0.208000000000001,
3.24001322621211));
#17299=CARTESIAN_POINT('Ctrl Pts',(1.87681490437036,0.670547542022765,3.24001322621211));
#17300=CARTESIAN_POINT('Ctrl Pts',(1.65897747541321,-0.208000000000001,
3.27464765209773));
#17301=CARTESIAN_POINT('Ctrl Pts',(1.65897747541321,0.670547542022765,3.27464765209773));
#17302=CARTESIAN_POINT('Ctrl Pts',(1.4191255439272,-0.208000000000001,3.30006519349576));
#17303=CARTESIAN_POINT('Ctrl Pts',(1.4191255439272,0.670547542022765,3.30006519349576));
#17304=CARTESIAN_POINT('Ctrl Pts',(1.15993538533448,-0.208000000000001,
3.31897283641381));
#17305=CARTESIAN_POINT('Ctrl Pts',(1.15993538533448,0.670547542022765,3.31897283641381));
#17306=CARTESIAN_POINT('Ctrl Pts',(0.884625090385968,-0.208000000000001,
3.33300441174764));
#17307=CARTESIAN_POINT('Ctrl Pts',(0.884625090385968,0.670547542022765,
3.33300441174764));
#17308=CARTESIAN_POINT('Ctrl Pts',(0.596845720618978,-0.208000000000001,
3.34293392264922));
#17309=CARTESIAN_POINT('Ctrl Pts',(0.596845720618978,0.670547542022765,
3.34293392264922));
#17310=CARTESIAN_POINT('Ctrl Pts',(0.30057321210183,-0.208000000000001,
3.34897162637417));
#17311=CARTESIAN_POINT('Ctrl Pts',(0.30057321210183,0.670547542022765,3.34897162637417));
#17312=CARTESIAN_POINT('Ctrl Pts',(1.66741620510891E-14,-0.208000000000001,
3.35102435732185));
#17313=CARTESIAN_POINT('Ctrl Pts',(1.66741620510891E-14,0.670547542022765,
3.35102435732185));
#17314=CARTESIAN_POINT('Ctrl Pts',(-0.300573212101791,-0.208000000000001,
3.34897162637426));
#17315=CARTESIAN_POINT('Ctrl Pts',(-0.300573212101791,0.670547542022765,
3.34897162637426));
#17316=CARTESIAN_POINT('Ctrl Pts',(-0.596845720618908,-0.208000000000001,
3.34293392264938));
#17317=CARTESIAN_POINT('Ctrl Pts',(-0.596845720618908,0.670547542022765,
3.34293392264938));
#17318=CARTESIAN_POINT('Ctrl Pts',(-0.884625090385886,-0.208000000000001,
3.33300441174785));
#17319=CARTESIAN_POINT('Ctrl Pts',(-0.884625090385886,0.670547542022765,
3.33300441174785));
#17320=CARTESIAN_POINT('Ctrl Pts',(-1.15993538533442,-0.208000000000001,
3.31897283641402));
#17321=CARTESIAN_POINT('Ctrl Pts',(-1.15993538533442,0.670547542022765,
3.31897283641402));
#17322=CARTESIAN_POINT('Ctrl Pts',(-1.41912554392716,-0.208000000000001,
3.30006519349591));
#17323=CARTESIAN_POINT('Ctrl Pts',(-1.41912554392716,0.670547542022765,
3.30006519349591));
#17324=CARTESIAN_POINT('Ctrl Pts',(-1.65897747541319,-0.208000000000001,
3.27464765209779));
#17325=CARTESIAN_POINT('Ctrl Pts',(-1.65897747541319,0.670547542022765,
3.27464765209779));
#17326=CARTESIAN_POINT('Ctrl Pts',(-1.87681490437034,-0.208000000000001,
3.24001322621208));
#17327=CARTESIAN_POINT('Ctrl Pts',(-1.87681490437034,0.670547542022765,
3.24001322621208));
#17328=CARTESIAN_POINT('Ctrl Pts',(-2.07061055216576,-0.208000000000001,
3.19196918412254));
#17329=CARTESIAN_POINT('Ctrl Pts',(-2.07061055216576,0.670547542022765,
3.19196918412254));
#17330=CARTESIAN_POINT('Ctrl Pts',(-2.23909845280547,-0.208000000000001,
3.12505646843295));
#17331=CARTESIAN_POINT('Ctrl Pts',(-2.23909845280547,0.670547542022765,
3.12505646843295));
#17332=CARTESIAN_POINT('Ctrl Pts',(-2.38189256086493,-0.208000000000001,
3.03403241435609));
#17333=CARTESIAN_POINT('Ctrl Pts',(-2.38189256086493,0.670547542022765,
3.03403241435609));
#17334=CARTESIAN_POINT('Ctrl Pts',(-2.49960870420481,-0.208000000000001,
2.91510580081997));
#17335=CARTESIAN_POINT('Ctrl Pts',(-2.49960870420481,0.670547542022765,
2.91510580081997));
#17336=CARTESIAN_POINT('Ctrl Pts',(-2.59397540849182,-0.208000000000001,
2.76722839711793));
#17337=CARTESIAN_POINT('Ctrl Pts',(-2.59397540849182,0.670547542022765,
2.76722839711793));
#17338=CARTESIAN_POINT('Ctrl Pts',(-2.66797634363209,-0.208000000000001,
2.59347738935767));
#17339=CARTESIAN_POINT('Ctrl Pts',(-2.66797634363209,0.670547542022765,
2.59347738935767));
#17340=CARTESIAN_POINT('Ctrl Pts',(-2.72531955636566,-0.208000000000001,
2.39962532458057));
#17341=CARTESIAN_POINT('Ctrl Pts',(-2.72531955636566,0.670547542022765,
2.39962532458057));
#17342=CARTESIAN_POINT('Ctrl Pts',(-2.76985908233936,-0.208000000000001,
2.19251877196088));
#17343=CARTESIAN_POINT('Ctrl Pts',(-2.76985908233936,0.670547542022765,
2.19251877196088));
#17344=CARTESIAN_POINT('Ctrl Pts',(-2.80505146480344,-0.208000000000001,
1.97856787413951));
#17345=CARTESIAN_POINT('Ctrl Pts',(-2.80505146480344,0.670547542022765,
1.97856787413951));
#17346=CARTESIAN_POINT('Ctrl Pts',(-2.8333568624899,-0.208000000000001,
1.76209503442131));
#17347=CARTESIAN_POINT('Ctrl Pts',(-2.8333568624899,0.670547542022765,1.76209503442131));
#17348=CARTESIAN_POINT('Ctrl Pts',(-2.85578261679294,-0.208000000000001,
1.54401727992238));
#17349=CARTESIAN_POINT('Ctrl Pts',(-2.85578261679294,0.670547542022765,
1.54401727992238));
#17350=CARTESIAN_POINT('Ctrl Pts',(-2.87284562964987,-0.208000000000001,
1.32371934078708));
#17351=CARTESIAN_POINT('Ctrl Pts',(-2.87284562964987,0.670547542022765,
1.32371934078708));
#17352=CARTESIAN_POINT('Ctrl Pts',(-2.88537704766869,-0.208000000000001,
1.10060381648384));
#17353=CARTESIAN_POINT('Ctrl Pts',(-2.88537704766869,0.670547542022765,
1.10060381648384));
#17354=CARTESIAN_POINT('Ctrl Pts',(-2.89547076625573,-0.208000000000001,
0.875890304828914));
#17355=CARTESIAN_POINT('Ctrl Pts',(-2.89547076625573,0.670547542022765,
0.875890304828914));
#17356=CARTESIAN_POINT('Ctrl Pts',(-2.90717911786707,-0.208000000000001,
0.654020230869684));
#17357=CARTESIAN_POINT('Ctrl Pts',(-2.90717911786707,0.670547542022765,
0.654020230869684));
#17358=CARTESIAN_POINT('Ctrl Pts',(-2.92780415844476,-0.208000000000001,
0.444963858672577));
#17359=CARTESIAN_POINT('Ctrl Pts',(-2.92780415844476,0.670547542022765,
0.444963858672577));
#17360=CARTESIAN_POINT('Ctrl Pts',(-2.96639254265869,-0.208000000000001,
0.262319630540737));
#17361=CARTESIAN_POINT('Ctrl Pts',(-2.96639254265869,0.670547542022765,
0.262319630540737));
#17362=CARTESIAN_POINT('Ctrl Pts',(-3.03063129752067,-0.208000000000001,
0.11901737132707));
#17363=CARTESIAN_POINT('Ctrl Pts',(-3.03063129752067,0.670547542022765,
0.11901737132707));
#17364=CARTESIAN_POINT('Ctrl Pts',(-3.12452733970658,-0.208000000000001,
0.0241851999813871));
#17365=CARTESIAN_POINT('Ctrl Pts',(-3.12452733970658,0.670547542022765,
0.0241851999813871));
#17366=CARTESIAN_POINT('Ctrl Pts',(-3.24511001026157,-0.208000000000001,
-0.0214179570895714));
#17367=CARTESIAN_POINT('Ctrl Pts',(-3.24511001026157,0.670547542022765,
-0.0214179570895714));
#17368=CARTESIAN_POINT('Ctrl Pts',(-3.38164698943802,-0.208000000000001,
-0.0263068037112043));
#17369=CARTESIAN_POINT('Ctrl Pts',(-3.38164698943802,0.670547542022765,
-0.0263068037112043));
#17370=CARTESIAN_POINT('Ctrl Pts',(-3.52045328348989,-0.208000000000001,
-0.00118366394785932));
#17371=CARTESIAN_POINT('Ctrl Pts',(-3.52045328348989,0.670547542022765,
-0.00118366394785932));
#17372=CARTESIAN_POINT('Ctrl Pts',(-3.64881642260079,-0.208000000000001,
0.0470540298718583));
#17373=CARTESIAN_POINT('Ctrl Pts',(-3.64881642260079,0.670547542022765,
0.0470540298718583));
#17374=CARTESIAN_POINT('Ctrl Pts',(-3.75872318140663,-0.208000000000001,
0.120497232333251));
#17375=CARTESIAN_POINT('Ctrl Pts',(-3.75872318140663,0.670547542022765,
0.120497232333251));
#17376=CARTESIAN_POINT('Ctrl Pts',(-3.84598208672296,-0.208000000000001,
0.224659532804408));
#17377=CARTESIAN_POINT('Ctrl Pts',(-3.84598208672296,0.670547542022765,
0.224659532804408));
#17378=CARTESIAN_POINT('Ctrl Pts',(-3.9098657241983,-0.208000000000001,
0.364350357241515));
#17379=CARTESIAN_POINT('Ctrl Pts',(-3.9098657241983,0.670547542022765,0.364350357241515));
#17380=CARTESIAN_POINT('Ctrl Pts',(-3.9525920016999,-0.208000000000001,
0.538436816836325));
#17381=CARTESIAN_POINT('Ctrl Pts',(-3.9525920016999,0.670547542022765,0.538436816836325));
#17382=CARTESIAN_POINT('Ctrl Pts',(-3.97841403016126,-0.208000000000001,
0.741129277895169));
#17383=CARTESIAN_POINT('Ctrl Pts',(-3.97841403016126,0.670547542022765,
0.741129277895169));
#17384=CARTESIAN_POINT('Ctrl Pts',(-3.99260375067011,-0.208000000000001,
0.964078729991154));
#17385=CARTESIAN_POINT('Ctrl Pts',(-3.99260375067011,0.670547542022765,
0.964078729991154));
#17386=CARTESIAN_POINT('Ctrl Pts',(-4.00047520099045,-0.208000000000001,
1.1981954227983));
#17387=CARTESIAN_POINT('Ctrl Pts',(-4.00047520099045,0.670547542022765,
1.1981954227983));
#17388=CARTESIAN_POINT('Ctrl Pts',(-4.00639322616607,-0.208000000000001,
1.43558101932923));
#17389=CARTESIAN_POINT('Ctrl Pts',(-4.00639322616607,0.670547542022765,
1.43558101932923));
#17390=CARTESIAN_POINT('Ctrl Pts',(-4.01278239926574,-0.208000000000001,
1.67142113207667));
#17391=CARTESIAN_POINT('Ctrl Pts',(-4.01278239926574,0.670547542022765,
1.67142113207667));
#17392=CARTESIAN_POINT('Ctrl Pts',(-4.02066709528487,-0.208000000000001,
1.90332556813333));
#17393=CARTESIAN_POINT('Ctrl Pts',(-4.02066709528487,0.670547542022765,
1.90332556813333));
#17394=CARTESIAN_POINT('Ctrl Pts',(-4.0302101444685,-0.208000000000001,
2.130657485557));
#17395=CARTESIAN_POINT('Ctrl Pts',(-4.0302101444685,0.670547542022765,2.130657485557));
#17396=CARTESIAN_POINT('Ctrl Pts',(-4.04126813644779,-0.208000000000001,
2.35385258470204));
#17397=CARTESIAN_POINT('Ctrl Pts',(-4.04126813644779,0.670547542022765,
2.35385258470204));
#17398=CARTESIAN_POINT('Ctrl Pts',(-4.05390260344525,-0.208000000000001,
2.57377631141659));
#17399=CARTESIAN_POINT('Ctrl Pts',(-4.05390260344525,0.670547542022765,
2.57377631141659));
#17400=CARTESIAN_POINT('Ctrl Pts',(-4.06899962712502,-0.208000000000001,
2.7909834104825));
#17401=CARTESIAN_POINT('Ctrl Pts',(-4.06899962712502,0.670547542022765,
2.7909834104825));
#17402=CARTESIAN_POINT('Ctrl Pts',(-4.08854433447739,-0.208000000000001,
3.00529120729338));
#17403=CARTESIAN_POINT('Ctrl Pts',(-4.08854433447739,0.670547542022765,
3.00529120729338));
#17404=CARTESIAN_POINT('Ctrl Pts',(-4.11518318246524,-0.208000000000001,
3.21600287470921));
#17405=CARTESIAN_POINT('Ctrl Pts',(-4.11518318246524,0.670547542022765,
3.21600287470921));
#17406=CARTESIAN_POINT('Ctrl Pts',(-4.15193466045748,-0.208000000000001,
3.42199345348447));
#17407=CARTESIAN_POINT('Ctrl Pts',(-4.15193466045748,0.670547542022765,
3.42199345348447));
#17408=CARTESIAN_POINT('Ctrl Pts',(-4.20184334854115,-0.208000000000001,
3.62185203209171));
#17409=CARTESIAN_POINT('Ctrl Pts',(-4.20184334854115,0.670547542022765,
3.62185203209171));
#17410=CARTESIAN_POINT('Ctrl Pts',(-4.26765207024395,-0.208000000000001,
3.81399668859083));
#17411=CARTESIAN_POINT('Ctrl Pts',(-4.26765207024395,0.670547542022765,
3.81399668859083));
#17412=CARTESIAN_POINT('Ctrl Pts',(-4.35148411330718,-0.208000000000001,
3.99681013615577));
#17413=CARTESIAN_POINT('Ctrl Pts',(-4.35148411330718,0.670547542022765,
3.99681013615577));
#17414=CARTESIAN_POINT('Ctrl Pts',(-4.45474519640294,-0.208000000000001,
4.16885849319142));
#17415=CARTESIAN_POINT('Ctrl Pts',(-4.45474519640294,0.670547542022765,
4.16885849319142));
#17416=CARTESIAN_POINT('Ctrl Pts',(-4.57800047823775,-0.208000000000001,
4.32911151507774));
#17417=CARTESIAN_POINT('Ctrl Pts',(-4.57800047823775,0.670547542022765,
4.32911151507774));
#17418=CARTESIAN_POINT('Ctrl Pts',(-4.7208720035032,-0.208000000000001,
4.47714872481861));
#17419=CARTESIAN_POINT('Ctrl Pts',(-4.7208720035032,0.670547542022765,4.47714872481861));
#17420=CARTESIAN_POINT('Ctrl Pts',(-4.88190185104852,-0.208000000000001,
4.61340315498244));
#17421=CARTESIAN_POINT('Ctrl Pts',(-4.88190185104852,0.670547542022765,
4.61340315498244));
#17422=CARTESIAN_POINT('Ctrl Pts',(-5.05850630701885,-0.208000000000001,
4.73929437247796));
#17423=CARTESIAN_POINT('Ctrl Pts',(-5.05850630701885,0.670547542022765,
4.73929437247796));
#17424=CARTESIAN_POINT('Ctrl Pts',(-5.24741086000019,-0.208000000000001,
4.8567611153285));
#17425=CARTESIAN_POINT('Ctrl Pts',(-5.24741086000019,0.670547542022765,
4.8567611153285));
#17426=CARTESIAN_POINT('Ctrl Pts',(-5.44501860313342,-0.208000000000001,
4.96787993373728));
#17427=CARTESIAN_POINT('Ctrl Pts',(-5.44501860313342,0.670547542022765,
4.96787993373728));
#17428=CARTESIAN_POINT('Ctrl Pts',(-5.64781737380319,-0.208000000000001,
5.07442896098937));
#17429=CARTESIAN_POINT('Ctrl Pts',(-5.64781737380319,0.670547542022765,
5.07442896098937));
#17430=CARTESIAN_POINT('Ctrl Pts',(-5.85274048349242,-0.208000000000001,
5.17752467829109));
#17431=CARTESIAN_POINT('Ctrl Pts',(-5.85274048349242,0.670547542022765,
5.17752467829109));
#17432=CARTESIAN_POINT('Ctrl Pts',(-6.05762450882858,-0.208000000000001,
5.27709955371564));
#17433=CARTESIAN_POINT('Ctrl Pts',(-6.05762450882858,0.670547542022765,
5.27709955371564));
#17434=CARTESIAN_POINT('Ctrl Pts',(-6.26112587698772,-0.208000000000001,
5.37226655127787));
#17435=CARTESIAN_POINT('Ctrl Pts',(-6.26112587698772,0.670547542022765,
5.37226655127787));
#17436=CARTESIAN_POINT('Ctrl Pts',(-6.46246210121964,-0.208000000000001,
5.46195513100446));
#17437=CARTESIAN_POINT('Ctrl Pts',(-6.46246210121964,0.670547542022765,
5.46195513100446));
#17438=CARTESIAN_POINT('Ctrl Pts',(-6.66121503090592,-0.208000000000001,
5.54547963906637));
#17439=CARTESIAN_POINT('Ctrl Pts',(-6.66121503090592,0.670547542022765,
5.54547963906637));
#17440=CARTESIAN_POINT('Ctrl Pts',(-6.8570997603751,-0.208000000000001,
5.62308582598972));
#17441=CARTESIAN_POINT('Ctrl Pts',(-6.8570997603751,0.670547542022765,5.62308582598972));
#17442=CARTESIAN_POINT('Ctrl Pts',(-7.04976847947249,-0.208000000000001,
5.69662713609756));
#17443=CARTESIAN_POINT('Ctrl Pts',(-7.04976847947249,0.670547542022765,
5.69662713609756));
#17444=CARTESIAN_POINT('Ctrl Pts',(-7.23853768475,-0.208000000000001,5.76979878895672));
#17445=CARTESIAN_POINT('Ctrl Pts',(-7.23853768475,0.670547542022765,5.76979878895672));
#17446=CARTESIAN_POINT('Ctrl Pts',(-7.42198551710617,-0.208000000000001,
5.84723737025949));
#17447=CARTESIAN_POINT('Ctrl Pts',(-7.42198551710617,0.670547542022765,
5.84723737025949));
#17448=CARTESIAN_POINT('Ctrl Pts',(-7.59751903688412,-0.208000000000001,
5.93381436957244));
#17449=CARTESIAN_POINT('Ctrl Pts',(-7.59751903688412,0.670547542022765,
5.93381436957244));
#17450=CARTESIAN_POINT('Ctrl Pts',(-7.76106756457753,-0.208000000000001,
6.03389995867283));
#17451=CARTESIAN_POINT('Ctrl Pts',(-7.76106756457753,0.670547542022765,
6.03389995867283));
#17452=CARTESIAN_POINT('Ctrl Pts',(-7.90644860448901,-0.208000000000001,
6.15052660592937));
#17453=CARTESIAN_POINT('Ctrl Pts',(-7.90644860448901,0.670547542022765,
6.15052660592937));
#17454=CARTESIAN_POINT('Ctrl Pts',(-8.02580908828117,-0.208000000000001,
6.28498018271686));
#17455=CARTESIAN_POINT('Ctrl Pts',(-8.02580908828117,0.670547542022765,
6.28498018271686));
#17456=CARTESIAN_POINT('Ctrl Pts',(-8.11207116917861,-0.208000000000001,
6.43720976255636));
#17457=CARTESIAN_POINT('Ctrl Pts',(-8.11207116917861,0.670547542022765,
6.43720976255636));
#17458=CARTESIAN_POINT('Ctrl Pts',(-8.16089752265956,-0.208000000000001,
6.60605451948903));
#17459=CARTESIAN_POINT('Ctrl Pts',(-8.16089752265956,0.670547542022765,
6.60605451948903));
#17460=CARTESIAN_POINT('Ctrl Pts',(-8.17293082304181,-0.208000000000001,
6.78954489191904));
#17461=CARTESIAN_POINT('Ctrl Pts',(-8.17293082304181,0.670547542022765,
6.78954489191904));
#17462=CARTESIAN_POINT('Ctrl Pts',(-8.15569042861244,-0.208000000000001,
6.9851692342788));
#17463=CARTESIAN_POINT('Ctrl Pts',(-8.15569042861244,0.670547542022765,
6.9851692342788));
#17464=CARTESIAN_POINT('Ctrl Pts',(-8.12057943633387,-0.208000000000001,
7.19009032473164));
#17465=CARTESIAN_POINT('Ctrl Pts',(-8.12057943633387,0.670547542022765,
7.19009032473164));
#17466=CARTESIAN_POINT('Ctrl Pts',(-8.08008348678073,-0.208000000000001,
7.40136016279791));
#17467=CARTESIAN_POINT('Ctrl Pts',(-8.08008348678073,0.670547542022765,
7.40136016279791));
#17468=CARTESIAN_POINT('Ctrl Pts',(-8.04494633492831,-0.208000000000001,
7.61613341658677));
#17469=CARTESIAN_POINT('Ctrl Pts',(-8.04494633492831,0.670547542022765,
7.61613341658677));
#17470=CARTESIAN_POINT('Ctrl Pts',(-8.02124364536279,-0.208000000000001,
7.83188673232793));
#17471=CARTESIAN_POINT('Ctrl Pts',(-8.02124364536279,0.670547542022765,
7.83188673232793));
#17472=CARTESIAN_POINT('Ctrl Pts',(-8.007818938056,-0.208000000000001,8.04662057355248));
#17473=CARTESIAN_POINT('Ctrl Pts',(-8.007818938056,0.670547542022765,8.04662057355248));
#17474=CARTESIAN_POINT('Ctrl Pts',(-7.99879843919661,-0.208000000000001,
8.25883677791483));
#17475=CARTESIAN_POINT('Ctrl Pts',(-7.99879843919661,0.670547542022765,
8.25883677791483));
#17476=CARTESIAN_POINT('Ctrl Pts',(-7.98575825096101,-0.208000000000001,
8.46752658699528));
#17477=CARTESIAN_POINT('Ctrl Pts',(-7.98575825096101,0.670547542022765,
8.46752658699528));
#17478=CARTESIAN_POINT('Ctrl Pts',(-7.96007609558389,-0.208000000000001,
8.67216210283896));
#17479=CARTESIAN_POINT('Ctrl Pts',(-7.96007609558389,0.670547542022765,
8.67216210283896));
#17480=CARTESIAN_POINT('Ctrl Pts',(-7.91508259073019,-0.208000000000001,
8.87266947141823));
#17481=CARTESIAN_POINT('Ctrl Pts',(-7.91508259073019,0.670547542022765,
8.87266947141823));
#17482=CARTESIAN_POINT('Ctrl Pts',(-7.84862074946261,-0.208000000000001,
9.06945407016992));
#17483=CARTESIAN_POINT('Ctrl Pts',(-7.84862074946261,0.670547542022765,
9.06945407016992));
#17484=CARTESIAN_POINT('Ctrl Pts',(-7.76209282457479,-0.208000000000001,
9.26297089919765));
#17485=CARTESIAN_POINT('Ctrl Pts',(-7.76209282457479,0.670547542022765,
9.26297089919765));
#17486=CARTESIAN_POINT('Ctrl Pts',(-7.65900038660722,-0.208000000000001,
9.4532499945042));
#17487=CARTESIAN_POINT('Ctrl Pts',(-7.65900038660722,0.670547542022765,
9.4532499945042));
#17488=CARTESIAN_POINT('Ctrl Pts',(-7.5436057352653,-0.208000000000001,
9.63939026966035));
#17489=CARTESIAN_POINT('Ctrl Pts',(-7.5436057352653,0.670547542022765,9.63939026966035));
#17490=CARTESIAN_POINT('Ctrl Pts',(-7.41967047355001,-0.208000000000001,
9.81917361987397));
#17491=CARTESIAN_POINT('Ctrl Pts',(-7.41967047355001,0.670547542022765,
9.81917361987397));
#17492=CARTESIAN_POINT('Ctrl Pts',(-7.28883796912703,-0.208000000000001,
9.98835756998572));
#17493=CARTESIAN_POINT('Ctrl Pts',(-7.28883796912703,0.670547542022765,
9.98835756998572));
#17494=CARTESIAN_POINT('Ctrl Pts',(-7.15081550722306,-0.208000000000001,
10.1414720974148));
#17495=CARTESIAN_POINT('Ctrl Pts',(-7.15081550722306,0.670547542022765,
10.1414720974148));
#17496=CARTESIAN_POINT('Ctrl Pts',(-7.0044544864105,-0.208000000000001,
10.2733319413008));
#17497=CARTESIAN_POINT('Ctrl Pts',(-7.0044544864105,0.670547542022765,10.2733319413008));
#17498=CARTESIAN_POINT('Ctrl Pts',(-6.84859008776113,-0.208000000000001,
10.3804015453596));
#17499=CARTESIAN_POINT('Ctrl Pts',(-6.84859008776113,0.670547542022765,
10.3804015453596));
#17500=CARTESIAN_POINT('Ctrl Pts',(-6.68288828293938,-0.208000000000001,
10.4620502678778));
#17501=CARTESIAN_POINT('Ctrl Pts',(-6.68288828293938,0.670547542022765,
10.4620502678778));
#17502=CARTESIAN_POINT('Ctrl Pts',(-6.50892555577766,-0.208000000000001,
10.522290883026));
#17503=CARTESIAN_POINT('Ctrl Pts',(-6.50892555577766,0.670547542022765,
10.522290883026));
#17504=CARTESIAN_POINT('Ctrl Pts',(-6.32976796473811,-0.208000000000001,
10.5687216653902));
#17505=CARTESIAN_POINT('Ctrl Pts',(-6.32976796473811,0.670547542022765,
10.5687216653902));
#17506=CARTESIAN_POINT('Ctrl Pts',(-6.14893768388701,-0.208000000000001,
10.6103475969885));
#17507=CARTESIAN_POINT('Ctrl Pts',(-6.14893768388701,0.670547542022765,
10.6103475969885));
#17508=CARTESIAN_POINT('Ctrl Pts',(-5.96961932707142,-0.208000000000001,
10.6558377434043));
#17509=CARTESIAN_POINT('Ctrl Pts',(-5.96961932707142,0.670547542022765,
10.6558377434043));
#17510=CARTESIAN_POINT('Ctrl Pts',(-5.79367695415031,-0.208000000000001,
10.7114411549114));
#17511=CARTESIAN_POINT('Ctrl Pts',(-5.79367695415031,0.670547542022765,
10.7114411549114));
#17512=CARTESIAN_POINT('Ctrl Pts',(-5.62101499943431,-0.208000000000001,
10.7795199127535));
#17513=CARTESIAN_POINT('Ctrl Pts',(-5.62101499943431,0.670547542022765,
10.7795199127535));
#17514=CARTESIAN_POINT('Ctrl Pts',(-5.45051506148982,-0.208000000000001,
10.8599381259737));
#17515=CARTESIAN_POINT('Ctrl Pts',(-5.45051506148982,0.670547542022765,
10.8599381259737));
#17516=CARTESIAN_POINT('Ctrl Pts',(-5.28082876351929,-0.208000000000001,
10.9511663773826));
#17517=CARTESIAN_POINT('Ctrl Pts',(-5.28082876351929,0.670547542022765,
10.9511663773826));
#17518=CARTESIAN_POINT('Ctrl Pts',(-5.11112998264616,-0.208000000000001,
11.0513704191329));
#17519=CARTESIAN_POINT('Ctrl Pts',(-5.11112998264616,0.670547542022765,
11.0513704191329));
#17520=CARTESIAN_POINT('Ctrl Pts',(-4.94211773226973,-0.208000000000001,
11.1598106424589));
#17521=CARTESIAN_POINT('Ctrl Pts',(-4.94211773226973,0.670547542022765,
11.1598106424589));
#17522=CARTESIAN_POINT('Ctrl Pts',(-4.77596612414951,-0.208000000000001,
11.2768795166235));
#17523=CARTESIAN_POINT('Ctrl Pts',(-4.77596612414951,0.670547542022765,
11.2768795166235));
#17524=CARTESIAN_POINT('Ctrl Pts',(-4.61532593596946,-0.208000000000001,
11.4029224160731));
#17525=CARTESIAN_POINT('Ctrl Pts',(-4.61532593596946,0.670547542022765,
11.4029224160731));
#17526=CARTESIAN_POINT('Ctrl Pts',(-4.46255574628757,-0.208000000000001,
11.5373242211527));
#17527=CARTESIAN_POINT('Ctrl Pts',(-4.46255574628757,0.670547542022765,
11.5373242211527));
#17528=CARTESIAN_POINT('Ctrl Pts',(-4.31893584999241,-0.208000000000001,
11.6776492463597));
#17529=CARTESIAN_POINT('Ctrl Pts',(-4.31893584999241,0.670547542022765,
11.6776492463597));
#17530=CARTESIAN_POINT('Ctrl Pts',(-4.18369962429796,-0.208000000000001,
11.8183570873721));
#17531=CARTESIAN_POINT('Ctrl Pts',(-4.18369962429796,0.670547542022765,
11.8183570873721));
#17532=CARTESIAN_POINT('Ctrl Pts',(-4.05395481372655,-0.208000000000001,
11.9514202619522));
#17533=CARTESIAN_POINT('Ctrl Pts',(-4.05395481372655,0.670547542022765,
11.9514202619522));
#17534=CARTESIAN_POINT('Ctrl Pts',(-3.92533033057354,-0.208000000000001,
12.0684942936867));
#17535=CARTESIAN_POINT('Ctrl Pts',(-3.92533033057354,0.670547542022765,
12.0684942936867));
#17536=CARTESIAN_POINT('Ctrl Pts',(-3.79241297762166,-0.208000000000001,
12.1626050652586));
#17537=CARTESIAN_POINT('Ctrl Pts',(-3.79241297762166,0.670547542022765,
12.1626050652586));
#17538=CARTESIAN_POINT('Ctrl Pts',(-3.64927048315908,-0.208000000000001,
12.2301117722809));
#17539=CARTESIAN_POINT('Ctrl Pts',(-3.64927048315908,0.670547542022765,
12.2301117722809));
#17540=CARTESIAN_POINT('Ctrl Pts',(-3.48993681214334,-0.208000000000001,
12.2723364229645));
#17541=CARTESIAN_POINT('Ctrl Pts',(-3.48993681214334,0.670547542022765,
12.2723364229645));
#17542=CARTESIAN_POINT('Ctrl Pts',(-3.30884480305534,-0.208000000000001,
12.2938762651139));
#17543=CARTESIAN_POINT('Ctrl Pts',(-3.30884480305534,0.670547542022765,
12.2938762651139));
#17544=CARTESIAN_POINT('Ctrl Pts',(-3.10127560868576,-0.208000000000001,
12.3010487961981));
#17545=CARTESIAN_POINT('Ctrl Pts',(-3.10127560868576,0.670547542022765,
12.3010487961981));
#17546=CARTESIAN_POINT('Ctrl Pts',(-2.86376302967345,-0.208000000000001,
12.300400839059));
#17547=CARTESIAN_POINT('Ctrl Pts',(-2.86376302967345,0.670547542022765,
12.300400839059));
#17548=CARTESIAN_POINT('Ctrl Pts',(-2.59461297443094,-0.208000000000001,
12.2969132923574));
#17549=CARTESIAN_POINT('Ctrl Pts',(-2.59461297443094,0.670547542022765,
12.2969132923574));
#17550=CARTESIAN_POINT('Ctrl Pts',(-2.29394197380209,-0.208000000000001,
12.2935845551224));
#17551=CARTESIAN_POINT('Ctrl Pts',(-2.29394197380209,0.670547542022765,
12.2935845551224));
#17552=CARTESIAN_POINT('Ctrl Pts',(-1.96338745719135,-0.208000000000001,
12.2919684497906));
#17553=CARTESIAN_POINT('Ctrl Pts',(-1.96338745719135,0.670547542022765,
12.2919684497906));
#17554=CARTESIAN_POINT('Ctrl Pts',(-1.60591558979456,-0.208000000000001,
12.2924280531798));
#17555=CARTESIAN_POINT('Ctrl Pts',(-1.60591558979456,0.670547542022765,
12.2924280531798));
#17556=CARTESIAN_POINT('Ctrl Pts',(-1.22558901314075,-0.208000000000001,
12.2945066442122));
#17557=CARTESIAN_POINT('Ctrl Pts',(-1.22558901314075,0.670547542022765,
12.2945066442122));
#17558=CARTESIAN_POINT('Ctrl Pts',(-0.827351903312651,-0.208000000000001,
12.2972483292773));
#17559=CARTESIAN_POINT('Ctrl Pts',(-0.827351903312651,0.670547542022765,
12.2972483292773));
#17560=CARTESIAN_POINT('Ctrl Pts',(-0.498916532526571,-0.208000000000001,
12.299081889758));
#17561=CARTESIAN_POINT('Ctrl Pts',(-0.498916532526571,0.670547542022765,
12.299081889758));
#17562=CARTESIAN_POINT('Ctrl Pts',(-0.249771440080693,-0.208000000000001,
12.2998330708668));
#17563=CARTESIAN_POINT('Ctrl Pts',(-0.249771440080693,0.670547542022765,
12.2998330708668));
#17564=CARTESIAN_POINT('Ctrl Pts',(-0.0832571466935557,-0.208000000000001,
12.2999999999989));
#17565=CARTESIAN_POINT('Ctrl Pts',(-0.0832571466935557,0.670547542022765,
12.2999999999989));
#17566=CARTESIAN_POINT('Ctrl Pts',(0.,-0.208000000000001,12.3));
#17567=CARTESIAN_POINT('Ctrl Pts',(0.,0.670547542022765,12.3));
#17568=CARTESIAN_POINT('Ctrl Pts',(0.0832571466935396,-0.208000000000001,
12.3000000000011));
#17569=CARTESIAN_POINT('Ctrl Pts',(0.0832571466935396,0.670547542022765,
12.3000000000011));
#17570=CARTESIAN_POINT('Ctrl Pts',(0.24977144008061,-0.208000000000001,
12.2998330708736));
#17571=CARTESIAN_POINT('Ctrl Pts',(0.24977144008061,0.670547542022765,12.2998330708736));
#17572=CARTESIAN_POINT('Ctrl Pts',(0.498916532526534,-0.208000000000001,
12.2990818897713));
#17573=CARTESIAN_POINT('Ctrl Pts',(0.498916532526534,0.670547542022765,
12.2990818897713));
#17574=CARTESIAN_POINT('Ctrl Pts',(0.827351903312438,-0.208000000000001,
12.2972483292974));
#17575=CARTESIAN_POINT('Ctrl Pts',(0.827351903312438,0.670547542022765,
12.2972483292974));
#17576=CARTESIAN_POINT('Ctrl Pts',(1.22558901314046,-0.208000000000001,
12.2945066442369));
#17577=CARTESIAN_POINT('Ctrl Pts',(1.22558901314046,0.670547542022765,12.2945066442369));
#17578=CARTESIAN_POINT('Ctrl Pts',(1.60591558979418,-0.208000000000001,
12.2924280532047));
#17579=CARTESIAN_POINT('Ctrl Pts',(1.60591558979418,0.670547542022765,12.2924280532047));
#17580=CARTESIAN_POINT('Ctrl Pts',(1.96338745719096,-0.208000000000001,
12.291968449812));
#17581=CARTESIAN_POINT('Ctrl Pts',(1.96338745719096,0.670547542022765,12.291968449812));
#17582=CARTESIAN_POINT('Ctrl Pts',(2.29394197380175,-0.208000000000001,
12.2935845551378));
#17583=CARTESIAN_POINT('Ctrl Pts',(2.29394197380175,0.670547542022765,12.2935845551378));
#17584=CARTESIAN_POINT('Ctrl Pts',(2.59461297443069,-0.208000000000001,
12.2969132923658));
#17585=CARTESIAN_POINT('Ctrl Pts',(2.59461297443069,0.670547542022765,12.2969132923658));
#17586=CARTESIAN_POINT('Ctrl Pts',(2.86376302967335,-0.208000000000001,
12.3004008390612));
#17587=CARTESIAN_POINT('Ctrl Pts',(2.86376302967335,0.670547542022765,12.3004008390612));
#17588=CARTESIAN_POINT('Ctrl Pts',(3.10127560868576,-0.208000000000001,
12.3010487961961));
#17589=CARTESIAN_POINT('Ctrl Pts',(3.10127560868576,0.670547542022765,12.3010487961961));
#17590=CARTESIAN_POINT('Ctrl Pts',(3.30884480305537,-0.208000000000001,
12.2938762651102));
#17591=CARTESIAN_POINT('Ctrl Pts',(3.30884480305537,0.670547542022765,12.2938762651102));
#17592=CARTESIAN_POINT('Ctrl Pts',(3.48993681214337,-0.208000000000001,
12.2723364229612));
#17593=CARTESIAN_POINT('Ctrl Pts',(3.48993681214337,0.670547542022765,12.2723364229612));
#17594=CARTESIAN_POINT('Ctrl Pts',(3.64927048315907,-0.208000000000001,
12.2301117722792));
#17595=CARTESIAN_POINT('Ctrl Pts',(3.64927048315907,0.670547542022765,12.2301117722792));
#17596=CARTESIAN_POINT('Ctrl Pts',(3.79241297762162,-0.208000000000001,
12.1626050652587));
#17597=CARTESIAN_POINT('Ctrl Pts',(3.79241297762162,0.670547542022765,12.1626050652587));
#17598=CARTESIAN_POINT('Ctrl Pts',(3.92533033057351,-0.208000000000001,
12.0684942936878));
#17599=CARTESIAN_POINT('Ctrl Pts',(3.92533033057351,0.670547542022765,12.0684942936878));
#17600=CARTESIAN_POINT('Ctrl Pts',(4.05395481372655,-0.208000000000001,
11.9514202619535));
#17601=CARTESIAN_POINT('Ctrl Pts',(4.05395481372655,0.670547542022765,11.9514202619535));
#17602=CARTESIAN_POINT('Ctrl Pts',(4.18369962429796,-0.208000000000001,
11.8183570873731));
#17603=CARTESIAN_POINT('Ctrl Pts',(4.18369962429796,0.670547542022765,11.8183570873731));
#17604=CARTESIAN_POINT('Ctrl Pts',(4.3189358499924,-0.208000000000001,11.67764924636));
#17605=CARTESIAN_POINT('Ctrl Pts',(4.3189358499924,0.670547542022765,11.67764924636));
#17606=CARTESIAN_POINT('Ctrl Pts',(4.46255574628753,-0.208000000000001,
11.5373242211525));
#17607=CARTESIAN_POINT('Ctrl Pts',(4.46255574628753,0.670547542022765,11.5373242211525));
#17608=CARTESIAN_POINT('Ctrl Pts',(4.61532593596939,-0.208000000000001,
11.4029224160728));
#17609=CARTESIAN_POINT('Ctrl Pts',(4.61532593596939,0.670547542022765,11.4029224160728));
#17610=CARTESIAN_POINT('Ctrl Pts',(4.77596612414944,-0.208000000000001,
11.2768795166233));
#17611=CARTESIAN_POINT('Ctrl Pts',(4.77596612414944,0.670547542022765,11.2768795166233));
#17612=CARTESIAN_POINT('Ctrl Pts',(4.94211773226968,-0.208000000000001,
11.1598106424589));
#17613=CARTESIAN_POINT('Ctrl Pts',(4.94211773226968,0.670547542022765,11.1598106424589));
#17614=CARTESIAN_POINT('Ctrl Pts',(5.11112998264613,-0.208000000000001,
11.051370419133));
#17615=CARTESIAN_POINT('Ctrl Pts',(5.11112998264613,0.670547542022765,11.051370419133));
#17616=CARTESIAN_POINT('Ctrl Pts',(5.28082876351925,-0.208000000000001,
10.9511663773825));
#17617=CARTESIAN_POINT('Ctrl Pts',(5.28082876351925,0.670547542022765,10.9511663773825));
#17618=CARTESIAN_POINT('Ctrl Pts',(5.45051506148977,-0.208000000000001,
10.8599381259735));
#17619=CARTESIAN_POINT('Ctrl Pts',(5.45051506148977,0.670547542022765,10.8599381259735));
#17620=CARTESIAN_POINT('Ctrl Pts',(5.62101499943423,-0.208000000000001,
10.7795199127532));
#17621=CARTESIAN_POINT('Ctrl Pts',(5.62101499943423,0.670547542022765,10.7795199127532));
#17622=CARTESIAN_POINT('Ctrl Pts',(5.7936769541502,-0.208000000000001,10.7114411549111));
#17623=CARTESIAN_POINT('Ctrl Pts',(5.7936769541502,0.670547542022765,10.7114411549111));
#17624=CARTESIAN_POINT('Ctrl Pts',(5.96961932707136,-0.208000000000001,
10.6558377434042));
#17625=CARTESIAN_POINT('Ctrl Pts',(5.96961932707136,0.670547542022765,10.6558377434042));
#17626=CARTESIAN_POINT('Ctrl Pts',(6.14893768388704,-0.208000000000001,
10.6103475969888));
#17627=CARTESIAN_POINT('Ctrl Pts',(6.14893768388704,0.670547542022765,10.6103475969888));
#17628=CARTESIAN_POINT('Ctrl Pts',(6.32976796473819,-0.208000000000001,
10.5687216653907));
#17629=CARTESIAN_POINT('Ctrl Pts',(6.32976796473819,0.670547542022765,10.5687216653907));
#17630=CARTESIAN_POINT('Ctrl Pts',(6.50892555577775,-0.208000000000001,
10.5222908830264));
#17631=CARTESIAN_POINT('Ctrl Pts',(6.50892555577775,0.670547542022765,10.5222908830264));
#17632=CARTESIAN_POINT('Ctrl Pts',(6.68288828293941,-0.208000000000001,
10.462050267878));
#17633=CARTESIAN_POINT('Ctrl Pts',(6.68288828293941,0.670547542022765,10.462050267878));
#17634=CARTESIAN_POINT('Ctrl Pts',(6.84859008776107,-0.208000000000001,
10.3804015453596));
#17635=CARTESIAN_POINT('Ctrl Pts',(6.84859008776107,0.670547542022765,10.3804015453596));
#17636=CARTESIAN_POINT('Ctrl Pts',(7.00445448641038,-0.208000000000001,
10.2733319413005));
#17637=CARTESIAN_POINT('Ctrl Pts',(7.00445448641038,0.670547542022765,10.2733319413005));
#17638=CARTESIAN_POINT('Ctrl Pts',(7.15081550722288,-0.208000000000001,
10.1414720974144));
#17639=CARTESIAN_POINT('Ctrl Pts',(7.15081550722288,0.670547542022765,10.1414720974144));
#17640=CARTESIAN_POINT('Ctrl Pts',(7.28883796912684,-0.208000000000001,
9.98835756998534));
#17641=CARTESIAN_POINT('Ctrl Pts',(7.28883796912684,0.670547542022765,9.98835756998534));
#17642=CARTESIAN_POINT('Ctrl Pts',(7.41967047354988,-0.208000000000001,
9.81917361987377));
#17643=CARTESIAN_POINT('Ctrl Pts',(7.41967047354988,0.670547542022765,9.81917361987377));
#17644=CARTESIAN_POINT('Ctrl Pts',(7.54360573526532,-0.208000000000001,
9.63939026966049));
#17645=CARTESIAN_POINT('Ctrl Pts',(7.54360573526532,0.670547542022765,9.63939026966049));
#17646=CARTESIAN_POINT('Ctrl Pts',(7.6590003866074,-0.208000000000001,9.45324999450471));
#17647=CARTESIAN_POINT('Ctrl Pts',(7.6590003866074,0.670547542022765,9.45324999450471));
#17648=CARTESIAN_POINT('Ctrl Pts',(7.76209282457502,-0.208000000000001,
9.26297089919836));
#17649=CARTESIAN_POINT('Ctrl Pts',(7.76209282457502,0.670547542022765,9.26297089919836));
#17650=CARTESIAN_POINT('Ctrl Pts',(7.84862074946283,-0.208000000000001,
9.06945407017055));
#17651=CARTESIAN_POINT('Ctrl Pts',(7.84862074946283,0.670547542022765,9.06945407017055));
#17652=CARTESIAN_POINT('Ctrl Pts',(7.91508259073031,-0.208000000000001,
8.87266947141857));
#17653=CARTESIAN_POINT('Ctrl Pts',(7.91508259073031,0.670547542022765,8.87266947141857));
#17654=CARTESIAN_POINT('Ctrl Pts',(7.96007609558387,-0.208000000000001,
8.67216210283894));
#17655=CARTESIAN_POINT('Ctrl Pts',(7.96007609558387,0.670547542022765,8.67216210283894));
#17656=CARTESIAN_POINT('Ctrl Pts',(7.98575825096082,-0.208000000000001,
8.46752658699496));
#17657=CARTESIAN_POINT('Ctrl Pts',(7.98575825096082,0.670547542022765,8.46752658699496));
#17658=CARTESIAN_POINT('Ctrl Pts',(7.9987984391963,-0.208000000000001,8.25883677791438));
#17659=CARTESIAN_POINT('Ctrl Pts',(7.9987984391963,0.670547542022765,8.25883677791438));
#17660=CARTESIAN_POINT('Ctrl Pts',(8.00781893805568,-0.208000000000001,
8.04662057355209));
#17661=CARTESIAN_POINT('Ctrl Pts',(8.00781893805568,0.670547542022765,8.04662057355209));
#17662=CARTESIAN_POINT('Ctrl Pts',(8.02124364536257,-0.208000000000001,
7.8318867323277));
#17663=CARTESIAN_POINT('Ctrl Pts',(8.02124364536257,0.670547542022765,7.8318867323277));
#17664=CARTESIAN_POINT('Ctrl Pts',(8.04494633492827,-0.208000000000001,
7.61613341658679));
#17665=CARTESIAN_POINT('Ctrl Pts',(8.04494633492827,0.670547542022765,7.61613341658679));
#17666=CARTESIAN_POINT('Ctrl Pts',(8.08008348678094,-0.208000000000001,
7.40136016279815));
#17667=CARTESIAN_POINT('Ctrl Pts',(8.08008348678094,0.670547542022765,7.40136016279815));
#17668=CARTESIAN_POINT('Ctrl Pts',(8.12057943633426,-0.208000000000001,
7.19009032473197));
#17669=CARTESIAN_POINT('Ctrl Pts',(8.12057943633426,0.670547542022765,7.19009032473197));
#17670=CARTESIAN_POINT('Ctrl Pts',(8.15569042861283,-0.208000000000001,
6.98516923427904));
#17671=CARTESIAN_POINT('Ctrl Pts',(8.15569042861283,0.670547542022765,6.98516923427904));
#17672=CARTESIAN_POINT('Ctrl Pts',(8.17293082304204,-0.208000000000001,
6.78954489191915));
#17673=CARTESIAN_POINT('Ctrl Pts',(8.17293082304204,0.670547542022765,6.78954489191915));
#17674=CARTESIAN_POINT('Ctrl Pts',(8.16089752265956,-0.208000000000001,
6.60605451948904));
#17675=CARTESIAN_POINT('Ctrl Pts',(8.16089752265956,0.670547542022765,6.60605451948904));
#17676=CARTESIAN_POINT('Ctrl Pts',(8.11207116917844,-0.208000000000001,
6.43720976255638));
#17677=CARTESIAN_POINT('Ctrl Pts',(8.11207116917844,0.670547542022765,6.43720976255638));
#17678=CARTESIAN_POINT('Ctrl Pts',(8.02580908828092,-0.208000000000001,
6.28498018271691));
#17679=CARTESIAN_POINT('Ctrl Pts',(8.02580908828092,0.670547542022765,6.28498018271691));
#17680=CARTESIAN_POINT('Ctrl Pts',(7.90644860448881,-0.208000000000001,
6.15052660592943));
#17681=CARTESIAN_POINT('Ctrl Pts',(7.90644860448881,0.670547542022765,6.15052660592943));
#17682=CARTESIAN_POINT('Ctrl Pts',(7.76106756457749,-0.208000000000001,
6.03389995867286));
#17683=CARTESIAN_POINT('Ctrl Pts',(7.76106756457749,0.670547542022765,6.03389995867286));
#17684=CARTESIAN_POINT('Ctrl Pts',(7.59751903688427,-0.208000000000001,
5.93381436957244));
#17685=CARTESIAN_POINT('Ctrl Pts',(7.59751903688427,0.670547542022765,5.93381436957244));
#17686=CARTESIAN_POINT('Ctrl Pts',(7.42198551710643,-0.208000000000001,
5.84723737025948));
#17687=CARTESIAN_POINT('Ctrl Pts',(7.42198551710643,0.670547542022765,5.84723737025948));
#17688=CARTESIAN_POINT('Ctrl Pts',(7.23853768475023,-0.208000000000001,
5.76979878895671));
#17689=CARTESIAN_POINT('Ctrl Pts',(7.23853768475023,0.670547542022765,5.76979878895671));
#17690=CARTESIAN_POINT('Ctrl Pts',(7.04976847947264,-0.208000000000001,
5.69662713609756));
#17691=CARTESIAN_POINT('Ctrl Pts',(7.04976847947264,0.670547542022765,5.69662713609756));
#17692=CARTESIAN_POINT('Ctrl Pts',(6.85709976037512,-0.208000000000001,
5.62308582598972));
#17693=CARTESIAN_POINT('Ctrl Pts',(6.85709976037512,0.670547542022765,5.62308582598972));
#17694=CARTESIAN_POINT('Ctrl Pts',(6.66121503090593,-0.208000000000001,
5.54547963906641));
#17695=CARTESIAN_POINT('Ctrl Pts',(6.66121503090593,0.670547542022765,5.54547963906641));
#17696=CARTESIAN_POINT('Ctrl Pts',(6.46246210121974,-0.208000000000001,
5.46195513100458));
#17697=CARTESIAN_POINT('Ctrl Pts',(6.46246210121974,0.670547542022765,5.46195513100458));
#17698=CARTESIAN_POINT('Ctrl Pts',(6.26112587698791,-0.208000000000001,
5.37226655127806));
#17699=CARTESIAN_POINT('Ctrl Pts',(6.26112587698791,0.670547542022765,5.37226655127806));
#17700=CARTESIAN_POINT('Ctrl Pts',(6.05762450882876,-0.208000000000001,
5.27709955371581));
#17701=CARTESIAN_POINT('Ctrl Pts',(6.05762450882876,0.670547542022765,5.27709955371581));
#17702=CARTESIAN_POINT('Ctrl Pts',(5.85274048349253,-0.208000000000001,
5.17752467829117));
#17703=CARTESIAN_POINT('Ctrl Pts',(5.85274048349253,0.670547542022765,5.17752467829117));
#17704=CARTESIAN_POINT('Ctrl Pts',(5.6478173738032,-0.208000000000001,5.07442896098936));
#17705=CARTESIAN_POINT('Ctrl Pts',(5.6478173738032,0.670547542022765,5.07442896098936));
#17706=CARTESIAN_POINT('Ctrl Pts',(5.44501860313336,-0.208000000000001,
4.96787993373722));
#17707=CARTESIAN_POINT('Ctrl Pts',(5.44501860313336,0.670547542022765,4.96787993373722));
#17708=CARTESIAN_POINT('Ctrl Pts',(5.24741086000008,-0.208000000000001,
4.85676111532844));
#17709=CARTESIAN_POINT('Ctrl Pts',(5.24741086000008,0.670547542022765,4.85676111532844));
#17710=CARTESIAN_POINT('Ctrl Pts',(5.05850630701875,-0.208000000000001,
4.73929437247794));
#17711=CARTESIAN_POINT('Ctrl Pts',(5.05850630701875,0.670547542022765,4.73929437247794));
#17712=CARTESIAN_POINT('Ctrl Pts',(4.88190185104846,-0.208000000000001,
4.61340315498245));
#17713=CARTESIAN_POINT('Ctrl Pts',(4.88190185104846,0.670547542022765,4.61340315498245));
#17714=CARTESIAN_POINT('Ctrl Pts',(4.7208720035032,-0.208000000000001,4.47714872481864));
#17715=CARTESIAN_POINT('Ctrl Pts',(4.7208720035032,0.670547542022765,4.47714872481864));
#17716=CARTESIAN_POINT('Ctrl Pts',(4.57800047823784,-0.208000000000001,
4.32911151507775));
#17717=CARTESIAN_POINT('Ctrl Pts',(4.57800047823784,0.670547542022765,4.32911151507775));
#17718=CARTESIAN_POINT('Ctrl Pts',(4.4547451964031,-0.208000000000001,4.16885849319143));
#17719=CARTESIAN_POINT('Ctrl Pts',(4.4547451964031,0.670547542022765,4.16885849319143));
#17720=CARTESIAN_POINT('Ctrl Pts',(4.35148411330737,-0.208000000000001,
3.99681013615577));
#17721=CARTESIAN_POINT('Ctrl Pts',(4.35148411330737,0.670547542022765,3.99681013615577));
#17722=CARTESIAN_POINT('Ctrl Pts',(4.26765207024408,-0.208000000000001,
3.81399668859083));
#17723=CARTESIAN_POINT('Ctrl Pts',(4.26765207024408,0.670547542022765,3.81399668859083));
#17724=CARTESIAN_POINT('Ctrl Pts',(4.20184334854117,-0.208000000000001,
3.62185203209172));
#17725=CARTESIAN_POINT('Ctrl Pts',(4.20184334854117,0.670547542022765,3.62185203209172));
#17726=CARTESIAN_POINT('Ctrl Pts',(4.15193466045737,-0.208000000000001,
3.42199345348454));
#17727=CARTESIAN_POINT('Ctrl Pts',(4.15193466045737,0.670547542022765,3.42199345348454));
#17728=CARTESIAN_POINT('Ctrl Pts',(4.11518318246501,-0.208000000000001,
3.21600287470933));
#17729=CARTESIAN_POINT('Ctrl Pts',(4.11518318246501,0.670547542022765,3.21600287470933));
#17730=CARTESIAN_POINT('Ctrl Pts',(4.08854433447712,-0.208000000000001,
3.00529120729351));
#17731=CARTESIAN_POINT('Ctrl Pts',(4.08854433447712,0.670547542022765,3.00529120729351));
#17732=CARTESIAN_POINT('Ctrl Pts',(4.06899962712481,-0.208000000000001,
2.7909834104826));
#17733=CARTESIAN_POINT('Ctrl Pts',(4.06899962712481,0.670547542022765,2.7909834104826));
#17734=CARTESIAN_POINT('Ctrl Pts',(4.05390260344518,-0.208000000000001,
2.57377631141663));
#17735=CARTESIAN_POINT('Ctrl Pts',(4.05390260344518,0.670547542022765,2.57377631141663));
#17736=CARTESIAN_POINT('Ctrl Pts',(4.04126813644791,-0.208000000000001,
2.35385258470204));
#17737=CARTESIAN_POINT('Ctrl Pts',(4.04126813644791,0.670547542022765,2.35385258470204));
#17738=CARTESIAN_POINT('Ctrl Pts',(4.03021014446877,-0.208000000000001,
2.13065748555701));
#17739=CARTESIAN_POINT('Ctrl Pts',(4.03021014446877,0.670547542022765,2.13065748555701));
#17740=CARTESIAN_POINT('Ctrl Pts',(4.02066709528519,-0.208000000000001,
1.9033255681334));
#17741=CARTESIAN_POINT('Ctrl Pts',(4.02066709528519,0.670547542022765,1.9033255681334));
#17742=CARTESIAN_POINT('Ctrl Pts',(4.01278884602726,-0.208000000000001,
1.67161074402007));
#17743=CARTESIAN_POINT('Ctrl Pts',(4.01278884602726,0.670547542022765,1.67161074402007));
#17744=CARTESIAN_POINT('Ctrl Pts',(4.00768150999064,-0.208000000000001,
1.4831346983285));
#17745=CARTESIAN_POINT('Ctrl Pts',(4.00768150999064,0.670547542022765,1.4831346983285));
#17746=CARTESIAN_POINT('Ctrl Pts',(4.00406437985138,-0.208000000000001,
1.34113083543346));
#17747=CARTESIAN_POINT('Ctrl Pts',(4.00406437985138,0.670547542022765,1.34113083543346));
#17748=CARTESIAN_POINT('Ctrl Pts',(4.00142780906472,-0.208000000000001,
1.24685503532231));
#17749=CARTESIAN_POINT('Ctrl Pts',(4.00142780906472,0.670547542022765,1.24685503532231));
#17750=CARTESIAN_POINT('Ctrl Pts',(4.,-0.208000000000001,1.2));
#17751=CARTESIAN_POINT('Ctrl Pts',(4.,0.670547542022765,1.2));
#17752=CARTESIAN_POINT('',(2.88353005387235,0.507243591474958,1.12422135153943));
#17753=CARTESIAN_POINT('',(2.88353005387235,0.507243591474958,1.12422135153943));
#17754=CARTESIAN_POINT('Origin',(2.87260862269811,0.9008070635013,1.19957807558011));
#17755=CARTESIAN_POINT('Origin',(3.2,0.9,1.2));
#17756=CARTESIAN_POINT('',(-4.5,0.,1.2));
#17757=CARTESIAN_POINT('Ctrl Pts',(2.80364150531137,0.507243591474958,1.2));
#17758=CARTESIAN_POINT('Ctrl Pts',(2.80364150531137,-0.00544871829499161,
1.2));
#17759=CARTESIAN_POINT('Ctrl Pts',(2.82677300877721,0.507243591474958,1.2));
#17760=CARTESIAN_POINT('Ctrl Pts',(2.82677300877721,-0.00544871829499161,
1.2));
#17761=CARTESIAN_POINT('Ctrl Pts',(2.86687234890104,0.507243591474958,1.18130982994417));
#17762=CARTESIAN_POINT('Ctrl Pts',(2.86687234890104,-0.00544871829499161,
1.18130982994417));
#17763=CARTESIAN_POINT('Ctrl Pts',(2.88261462067456,0.507243591474958,1.14154581001993));
#17764=CARTESIAN_POINT('Ctrl Pts',(2.88261462067456,-0.00544871829499161,
1.14154581001993));
#17765=CARTESIAN_POINT('Ctrl Pts',(2.88353005387235,0.507243591474958,1.12422135153943));
#17766=CARTESIAN_POINT('Ctrl Pts',(2.88353005387235,-0.00544871829499161,
1.12422135153943));
#17767=CARTESIAN_POINT('',(2.80364150531137,0.5,1.2));
#17768=CARTESIAN_POINT('',(2.80364150531137,0.08,1.2));
#17769=CARTESIAN_POINT('Ctrl Pts',(2.80364150531137,0.5,1.2));
#17770=CARTESIAN_POINT('Ctrl Pts',(2.81379585169868,0.5,1.2));
#17771=CARTESIAN_POINT('Ctrl Pts',(2.82391024805161,0.499987289115092,1.19794137540632));
#17772=CARTESIAN_POINT('Ctrl Pts',(2.84273358019748,0.500098331041066,1.19035456836199));
#17773=CARTESIAN_POINT('Ctrl Pts',(2.85145390051855,0.500227305282778,1.18482590803764));
#17774=CARTESIAN_POINT('Ctrl Pts',(2.86742097463828,0.501061125385064,1.16977413119873));
#17775=CARTESIAN_POINT('Ctrl Pts',(2.87283116118724,0.501825922612233,1.16103188260708));
#17776=CARTESIAN_POINT('Ctrl Pts',(2.88055159121655,0.503819244531482,1.14408694758658));
#17777=CARTESIAN_POINT('Ctrl Pts',(2.8830040002538,0.505322771788675,1.13417685030768));
#17778=CARTESIAN_POINT('Ctrl Pts',(2.88353005387235,0.507243591474958,1.12422135153943));
#17779=CARTESIAN_POINT('Origin',(-4.18004567262178,-4.54425157915634E-9,
3.08202038908016));
#17780=CARTESIAN_POINT('',(-4.10062628985476,0.500000490290817,3.09201395473891));
#17781=CARTESIAN_POINT('',(-4.1,0.5,3.08202325217327));
#17782=CARTESIAN_POINT('Origin',(-4.1800260995291,0.500109554898197,3.08202161069944));
#17783=CARTESIAN_POINT('',(-4.1,0.5,3.08202325217208));
#17784=CARTESIAN_POINT('',(-4.1006262898548,2.17910572199157E-7,3.09201395473924));
#17785=CARTESIAN_POINT('Ctrl Pts',(-4.07743349288644,-3.,2.87542908850901));
#17786=CARTESIAN_POINT('Ctrl Pts',(-4.07743349288644,4.2,2.87542908850901));
#17787=CARTESIAN_POINT('Ctrl Pts',(-4.07979010068817,-3.,2.90134289838335));
#17788=CARTESIAN_POINT('Ctrl Pts',(-4.07979010068817,4.2,2.90134289838335));
#17789=CARTESIAN_POINT('Ctrl Pts',(-4.08631563412149,-3.,2.97000159076542));
#17790=CARTESIAN_POINT('Ctrl Pts',(-4.08631563412149,4.2,2.97000159076542));
#17791=CARTESIAN_POINT('Ctrl Pts',(-4.09817039437236,-3.,3.08076873096245));
#17792=CARTESIAN_POINT('Ctrl Pts',(-4.09817039437236,4.2,3.08076873096245));
#17793=CARTESIAN_POINT('Ctrl Pts',(-4.11809350439417,-3.,3.23231511387111));
#17794=CARTESIAN_POINT('Ctrl Pts',(-4.11809350439417,4.2,3.23231511387111));
#17795=CARTESIAN_POINT('Ctrl Pts',(-4.15193466045748,-3.,3.42199345348447));
#17796=CARTESIAN_POINT('Ctrl Pts',(-4.15193466045748,4.2,3.42199345348447));
#17797=CARTESIAN_POINT('Ctrl Pts',(-4.20184334854115,-3.,3.62185203209171));
#17798=CARTESIAN_POINT('Ctrl Pts',(-4.20184334854115,4.2,3.62185203209171));
#17799=CARTESIAN_POINT('Ctrl Pts',(-4.26765207024395,-3.,3.81399668859083));
#17800=CARTESIAN_POINT('Ctrl Pts',(-4.26765207024395,4.2,3.81399668859083));
#17801=CARTESIAN_POINT('Ctrl Pts',(-4.35148411330718,-3.,3.99681013615577));
#17802=CARTESIAN_POINT('Ctrl Pts',(-4.35148411330718,4.2,3.99681013615577));
#17803=CARTESIAN_POINT('Ctrl Pts',(-4.45474519640294,-3.,4.16885849319142));
#17804=CARTESIAN_POINT('Ctrl Pts',(-4.45474519640294,4.2,4.16885849319142));
#17805=CARTESIAN_POINT('Ctrl Pts',(-4.57800047823775,-3.,4.32911151507774));
#17806=CARTESIAN_POINT('Ctrl Pts',(-4.57800047823775,4.2,4.32911151507774));
#17807=CARTESIAN_POINT('Ctrl Pts',(-4.7208720035032,-3.,4.47714872481861));
#17808=CARTESIAN_POINT('Ctrl Pts',(-4.7208720035032,4.2,4.47714872481861));
#17809=CARTESIAN_POINT('Ctrl Pts',(-4.88190185104852,-3.,4.61340315498244));
#17810=CARTESIAN_POINT('Ctrl Pts',(-4.88190185104852,4.2,4.61340315498244));
#17811=CARTESIAN_POINT('Ctrl Pts',(-5.05850630701885,-3.,4.73929437247796));
#17812=CARTESIAN_POINT('Ctrl Pts',(-5.05850630701885,4.2,4.73929437247796));
#17813=CARTESIAN_POINT('Ctrl Pts',(-5.24741086000019,-3.,4.8567611153285));
#17814=CARTESIAN_POINT('Ctrl Pts',(-5.24741086000019,4.2,4.8567611153285));
#17815=CARTESIAN_POINT('Ctrl Pts',(-5.44501860313342,-3.,4.96787993373728));
#17816=CARTESIAN_POINT('Ctrl Pts',(-5.44501860313342,4.2,4.96787993373728));
#17817=CARTESIAN_POINT('Ctrl Pts',(-5.64781737380319,-3.,5.07442896098937));
#17818=CARTESIAN_POINT('Ctrl Pts',(-5.64781737380319,4.2,5.07442896098937));
#17819=CARTESIAN_POINT('Ctrl Pts',(-5.85274048349242,-3.,5.17752467829109));
#17820=CARTESIAN_POINT('Ctrl Pts',(-5.85274048349242,4.2,5.17752467829109));
#17821=CARTESIAN_POINT('Ctrl Pts',(-6.05762450882858,-3.,5.27709955371564));
#17822=CARTESIAN_POINT('Ctrl Pts',(-6.05762450882858,4.2,5.27709955371564));
#17823=CARTESIAN_POINT('Ctrl Pts',(-6.26112587698772,-3.,5.37226655127787));
#17824=CARTESIAN_POINT('Ctrl Pts',(-6.26112587698772,4.2,5.37226655127787));
#17825=CARTESIAN_POINT('Ctrl Pts',(-6.46246210121964,-3.,5.46195513100446));
#17826=CARTESIAN_POINT('Ctrl Pts',(-6.46246210121964,4.2,5.46195513100446));
#17827=CARTESIAN_POINT('Ctrl Pts',(-6.66121503090592,-3.,5.54547963906637));
#17828=CARTESIAN_POINT('Ctrl Pts',(-6.66121503090592,4.2,5.54547963906637));
#17829=CARTESIAN_POINT('Ctrl Pts',(-6.8570997603751,-3.,5.62308582598972));
#17830=CARTESIAN_POINT('Ctrl Pts',(-6.8570997603751,4.2,5.62308582598972));
#17831=CARTESIAN_POINT('Ctrl Pts',(-7.04976847947249,-3.,5.69662713609756));
#17832=CARTESIAN_POINT('Ctrl Pts',(-7.04976847947249,4.2,5.69662713609756));
#17833=CARTESIAN_POINT('Ctrl Pts',(-7.23853768475,-3.,5.76979878895672));
#17834=CARTESIAN_POINT('Ctrl Pts',(-7.23853768475,4.2,5.76979878895672));
#17835=CARTESIAN_POINT('Ctrl Pts',(-7.42198551710617,-3.,5.84723737025949));
#17836=CARTESIAN_POINT('Ctrl Pts',(-7.42198551710617,4.2,5.84723737025949));
#17837=CARTESIAN_POINT('Ctrl Pts',(-7.59751903688412,-3.,5.93381436957244));
#17838=CARTESIAN_POINT('Ctrl Pts',(-7.59751903688412,4.2,5.93381436957244));
#17839=CARTESIAN_POINT('Ctrl Pts',(-7.76106756457753,-3.,6.03389995867283));
#17840=CARTESIAN_POINT('Ctrl Pts',(-7.76106756457753,4.2,6.03389995867283));
#17841=CARTESIAN_POINT('Ctrl Pts',(-7.90644860448901,-3.,6.15052660592937));
#17842=CARTESIAN_POINT('Ctrl Pts',(-7.90644860448901,4.2,6.15052660592937));
#17843=CARTESIAN_POINT('Ctrl Pts',(-8.02580908828117,-3.,6.28498018271686));
#17844=CARTESIAN_POINT('Ctrl Pts',(-8.02580908828117,4.2,6.28498018271686));
#17845=CARTESIAN_POINT('Ctrl Pts',(-8.11207116917861,-3.,6.43720976255636));
#17846=CARTESIAN_POINT('Ctrl Pts',(-8.11207116917861,4.2,6.43720976255636));
#17847=CARTESIAN_POINT('Ctrl Pts',(-8.16089752265956,-3.,6.60605451948903));
#17848=CARTESIAN_POINT('Ctrl Pts',(-8.16089752265956,4.2,6.60605451948903));
#17849=CARTESIAN_POINT('Ctrl Pts',(-8.17293082304181,-3.,6.78954489191904));
#17850=CARTESIAN_POINT('Ctrl Pts',(-8.17293082304181,4.2,6.78954489191904));
#17851=CARTESIAN_POINT('Ctrl Pts',(-8.15569042861244,-3.,6.9851692342788));
#17852=CARTESIAN_POINT('Ctrl Pts',(-8.15569042861244,4.2,6.9851692342788));
#17853=CARTESIAN_POINT('Ctrl Pts',(-8.12057943633387,-3.,7.19009032473164));
#17854=CARTESIAN_POINT('Ctrl Pts',(-8.12057943633387,4.2,7.19009032473164));
#17855=CARTESIAN_POINT('Ctrl Pts',(-8.08008348678073,-3.,7.40136016279791));
#17856=CARTESIAN_POINT('Ctrl Pts',(-8.08008348678073,4.2,7.40136016279791));
#17857=CARTESIAN_POINT('Ctrl Pts',(-8.04494633492831,-3.,7.61613341658677));
#17858=CARTESIAN_POINT('Ctrl Pts',(-8.04494633492831,4.2,7.61613341658677));
#17859=CARTESIAN_POINT('Ctrl Pts',(-8.02124364536279,-3.,7.83188673232793));
#17860=CARTESIAN_POINT('Ctrl Pts',(-8.02124364536279,4.2,7.83188673232793));
#17861=CARTESIAN_POINT('Ctrl Pts',(-8.007818938056,-3.,8.04662057355248));
#17862=CARTESIAN_POINT('Ctrl Pts',(-8.007818938056,4.2,8.04662057355248));
#17863=CARTESIAN_POINT('Ctrl Pts',(-7.99879843919661,-3.,8.25883677791483));
#17864=CARTESIAN_POINT('Ctrl Pts',(-7.99879843919661,4.2,8.25883677791483));
#17865=CARTESIAN_POINT('Ctrl Pts',(-7.98575825096101,-3.,8.46752658699528));
#17866=CARTESIAN_POINT('Ctrl Pts',(-7.98575825096101,4.2,8.46752658699528));
#17867=CARTESIAN_POINT('Ctrl Pts',(-7.96007609558389,-3.,8.67216210283896));
#17868=CARTESIAN_POINT('Ctrl Pts',(-7.96007609558389,4.2,8.67216210283896));
#17869=CARTESIAN_POINT('Ctrl Pts',(-7.91508259073019,-3.,8.87266947141823));
#17870=CARTESIAN_POINT('Ctrl Pts',(-7.91508259073019,4.2,8.87266947141823));
#17871=CARTESIAN_POINT('Ctrl Pts',(-7.84862074946261,-3.,9.06945407016992));
#17872=CARTESIAN_POINT('Ctrl Pts',(-7.84862074946261,4.2,9.06945407016992));
#17873=CARTESIAN_POINT('Ctrl Pts',(-7.76209282457479,-3.,9.26297089919765));
#17874=CARTESIAN_POINT('Ctrl Pts',(-7.76209282457479,4.2,9.26297089919765));
#17875=CARTESIAN_POINT('Ctrl Pts',(-7.65900038660722,-3.,9.4532499945042));
#17876=CARTESIAN_POINT('Ctrl Pts',(-7.65900038660722,4.2,9.4532499945042));
#17877=CARTESIAN_POINT('Ctrl Pts',(-7.5436057352653,-3.,9.63939026966035));
#17878=CARTESIAN_POINT('Ctrl Pts',(-7.5436057352653,4.2,9.63939026966035));
#17879=CARTESIAN_POINT('Ctrl Pts',(-7.41967047355001,-3.,9.81917361987397));
#17880=CARTESIAN_POINT('Ctrl Pts',(-7.41967047355001,4.2,9.81917361987397));
#17881=CARTESIAN_POINT('Ctrl Pts',(-7.28883796912703,-3.,9.98835756998572));
#17882=CARTESIAN_POINT('Ctrl Pts',(-7.28883796912703,4.2,9.98835756998572));
#17883=CARTESIAN_POINT('Ctrl Pts',(-7.15081550722306,-3.,10.1414720974148));
#17884=CARTESIAN_POINT('Ctrl Pts',(-7.15081550722306,4.2,10.1414720974148));
#17885=CARTESIAN_POINT('Ctrl Pts',(-7.0044544864105,-3.,10.2733319413008));
#17886=CARTESIAN_POINT('Ctrl Pts',(-7.0044544864105,4.2,10.2733319413008));
#17887=CARTESIAN_POINT('Ctrl Pts',(-6.84859008776113,-3.,10.3804015453596));
#17888=CARTESIAN_POINT('Ctrl Pts',(-6.84859008776113,4.2,10.3804015453596));
#17889=CARTESIAN_POINT('Ctrl Pts',(-6.68288828293938,-3.,10.4620502678778));
#17890=CARTESIAN_POINT('Ctrl Pts',(-6.68288828293938,4.2,10.4620502678778));
#17891=CARTESIAN_POINT('Ctrl Pts',(-6.50892555577766,-3.,10.522290883026));
#17892=CARTESIAN_POINT('Ctrl Pts',(-6.50892555577766,4.2,10.522290883026));
#17893=CARTESIAN_POINT('Ctrl Pts',(-6.32976796473811,-3.,10.5687216653902));
#17894=CARTESIAN_POINT('Ctrl Pts',(-6.32976796473811,4.2,10.5687216653902));
#17895=CARTESIAN_POINT('Ctrl Pts',(-6.14893768388701,-3.,10.6103475969885));
#17896=CARTESIAN_POINT('Ctrl Pts',(-6.14893768388701,4.2,10.6103475969885));
#17897=CARTESIAN_POINT('Ctrl Pts',(-5.96961932707142,-3.,10.6558377434043));
#17898=CARTESIAN_POINT('Ctrl Pts',(-5.96961932707142,4.2,10.6558377434043));
#17899=CARTESIAN_POINT('Ctrl Pts',(-5.79367695415031,-3.,10.7114411549114));
#17900=CARTESIAN_POINT('Ctrl Pts',(-5.79367695415031,4.2,10.7114411549114));
#17901=CARTESIAN_POINT('Ctrl Pts',(-5.62101499943431,-3.,10.7795199127535));
#17902=CARTESIAN_POINT('Ctrl Pts',(-5.62101499943431,4.2,10.7795199127535));
#17903=CARTESIAN_POINT('Ctrl Pts',(-5.45051506148982,-3.,10.8599381259737));
#17904=CARTESIAN_POINT('Ctrl Pts',(-5.45051506148982,4.2,10.8599381259737));
#17905=CARTESIAN_POINT('Ctrl Pts',(-5.28082876351929,-3.,10.9511663773826));
#17906=CARTESIAN_POINT('Ctrl Pts',(-5.28082876351929,4.2,10.9511663773826));
#17907=CARTESIAN_POINT('Ctrl Pts',(-5.11112998264616,-3.,11.0513704191329));
#17908=CARTESIAN_POINT('Ctrl Pts',(-5.11112998264616,4.2,11.0513704191329));
#17909=CARTESIAN_POINT('Ctrl Pts',(-4.94211773226973,-3.,11.1598106424589));
#17910=CARTESIAN_POINT('Ctrl Pts',(-4.94211773226973,4.2,11.1598106424589));
#17911=CARTESIAN_POINT('Ctrl Pts',(-4.77596612414951,-3.,11.2768795166235));
#17912=CARTESIAN_POINT('Ctrl Pts',(-4.77596612414951,4.2,11.2768795166235));
#17913=CARTESIAN_POINT('Ctrl Pts',(-4.61532593596946,-3.,11.4029224160731));
#17914=CARTESIAN_POINT('Ctrl Pts',(-4.61532593596946,4.2,11.4029224160731));
#17915=CARTESIAN_POINT('Ctrl Pts',(-4.46255574628757,-3.,11.5373242211527));
#17916=CARTESIAN_POINT('Ctrl Pts',(-4.46255574628757,4.2,11.5373242211527));
#17917=CARTESIAN_POINT('Ctrl Pts',(-4.31893584999241,-3.,11.6776492463597));
#17918=CARTESIAN_POINT('Ctrl Pts',(-4.31893584999241,4.2,11.6776492463597));
#17919=CARTESIAN_POINT('Ctrl Pts',(-4.18369962429796,-3.,11.8183570873721));
#17920=CARTESIAN_POINT('Ctrl Pts',(-4.18369962429796,4.2,11.8183570873721));
#17921=CARTESIAN_POINT('Ctrl Pts',(-4.05395481372655,-3.,11.9514202619522));
#17922=CARTESIAN_POINT('Ctrl Pts',(-4.05395481372655,4.2,11.9514202619522));
#17923=CARTESIAN_POINT('Ctrl Pts',(-3.92533033057354,-3.,12.0684942936867));
#17924=CARTESIAN_POINT('Ctrl Pts',(-3.92533033057354,4.2,12.0684942936867));
#17925=CARTESIAN_POINT('Ctrl Pts',(-3.79241297762166,-3.,12.1626050652586));
#17926=CARTESIAN_POINT('Ctrl Pts',(-3.79241297762166,4.2,12.1626050652586));
#17927=CARTESIAN_POINT('Ctrl Pts',(-3.64927048315908,-3.,12.2301117722809));
#17928=CARTESIAN_POINT('Ctrl Pts',(-3.64927048315908,4.2,12.2301117722809));
#17929=CARTESIAN_POINT('Ctrl Pts',(-3.48993681214334,-3.,12.2723364229645));
#17930=CARTESIAN_POINT('Ctrl Pts',(-3.48993681214334,4.2,12.2723364229645));
#17931=CARTESIAN_POINT('Ctrl Pts',(-3.30884480305534,-3.,12.2938762651139));
#17932=CARTESIAN_POINT('Ctrl Pts',(-3.30884480305534,4.2,12.2938762651139));
#17933=CARTESIAN_POINT('Ctrl Pts',(-3.10127560868576,-3.,12.3010487961981));
#17934=CARTESIAN_POINT('Ctrl Pts',(-3.10127560868576,4.2,12.3010487961981));
#17935=CARTESIAN_POINT('Ctrl Pts',(-2.86376302967345,-3.,12.300400839059));
#17936=CARTESIAN_POINT('Ctrl Pts',(-2.86376302967345,4.2,12.300400839059));
#17937=CARTESIAN_POINT('Ctrl Pts',(-2.59461297443094,-3.,12.2969132923574));
#17938=CARTESIAN_POINT('Ctrl Pts',(-2.59461297443094,4.2,12.2969132923574));
#17939=CARTESIAN_POINT('Ctrl Pts',(-2.29394197380209,-3.,12.2935845551224));
#17940=CARTESIAN_POINT('Ctrl Pts',(-2.29394197380209,4.2,12.2935845551224));
#17941=CARTESIAN_POINT('Ctrl Pts',(-1.96338745719135,-3.,12.2919684497906));
#17942=CARTESIAN_POINT('Ctrl Pts',(-1.96338745719135,4.2,12.2919684497906));
#17943=CARTESIAN_POINT('Ctrl Pts',(-1.60591558979456,-3.,12.2924280531798));
#17944=CARTESIAN_POINT('Ctrl Pts',(-1.60591558979456,4.2,12.2924280531798));
#17945=CARTESIAN_POINT('Ctrl Pts',(-1.22558901314075,-3.,12.2945066442122));
#17946=CARTESIAN_POINT('Ctrl Pts',(-1.22558901314075,4.2,12.2945066442122));
#17947=CARTESIAN_POINT('Ctrl Pts',(-0.827351903312651,-3.,12.2972483292773));
#17948=CARTESIAN_POINT('Ctrl Pts',(-0.827351903312651,4.2,12.2972483292773));
#17949=CARTESIAN_POINT('Ctrl Pts',(-0.498916532526571,-3.,12.299081889758));
#17950=CARTESIAN_POINT('Ctrl Pts',(-0.498916532526571,4.2,12.299081889758));
#17951=CARTESIAN_POINT('Ctrl Pts',(-0.249771440080693,-3.,12.2998330708668));
#17952=CARTESIAN_POINT('Ctrl Pts',(-0.249771440080693,4.2,12.2998330708668));
#17953=CARTESIAN_POINT('Ctrl Pts',(-0.0832571466935557,-3.,12.2999999999989));
#17954=CARTESIAN_POINT('Ctrl Pts',(-0.0832571466935557,4.2,12.2999999999989));
#17955=CARTESIAN_POINT('Ctrl Pts',(0.,-3.,12.3));
#17956=CARTESIAN_POINT('Ctrl Pts',(0.,4.2,12.3));
#17957=CARTESIAN_POINT('Ctrl Pts',(0.0832571466935396,-3.,12.3000000000011));
#17958=CARTESIAN_POINT('Ctrl Pts',(0.0832571466935396,4.2,12.3000000000011));
#17959=CARTESIAN_POINT('Ctrl Pts',(0.24977144008061,-3.,12.2998330708736));
#17960=CARTESIAN_POINT('Ctrl Pts',(0.24977144008061,4.2,12.2998330708736));
#17961=CARTESIAN_POINT('Ctrl Pts',(0.498916532526534,-3.,12.2990818897713));
#17962=CARTESIAN_POINT('Ctrl Pts',(0.498916532526534,4.2,12.2990818897713));
#17963=CARTESIAN_POINT('Ctrl Pts',(0.827351903312438,-3.,12.2972483292974));
#17964=CARTESIAN_POINT('Ctrl Pts',(0.827351903312438,4.2,12.2972483292974));
#17965=CARTESIAN_POINT('Ctrl Pts',(1.22558901314046,-3.,12.2945066442369));
#17966=CARTESIAN_POINT('Ctrl Pts',(1.22558901314046,4.2,12.2945066442369));
#17967=CARTESIAN_POINT('Ctrl Pts',(1.60591558979418,-3.,12.2924280532047));
#17968=CARTESIAN_POINT('Ctrl Pts',(1.60591558979418,4.2,12.2924280532047));
#17969=CARTESIAN_POINT('Ctrl Pts',(1.96338745719096,-3.,12.291968449812));
#17970=CARTESIAN_POINT('Ctrl Pts',(1.96338745719096,4.2,12.291968449812));
#17971=CARTESIAN_POINT('Ctrl Pts',(2.29394197380175,-3.,12.2935845551378));
#17972=CARTESIAN_POINT('Ctrl Pts',(2.29394197380175,4.2,12.2935845551378));
#17973=CARTESIAN_POINT('Ctrl Pts',(2.59461297443069,-3.,12.2969132923658));
#17974=CARTESIAN_POINT('Ctrl Pts',(2.59461297443069,4.2,12.2969132923658));
#17975=CARTESIAN_POINT('Ctrl Pts',(2.86376302967335,-3.,12.3004008390612));
#17976=CARTESIAN_POINT('Ctrl Pts',(2.86376302967335,4.2,12.3004008390612));
#17977=CARTESIAN_POINT('Ctrl Pts',(3.10127560868576,-3.,12.3010487961961));
#17978=CARTESIAN_POINT('Ctrl Pts',(3.10127560868576,4.2,12.3010487961961));
#17979=CARTESIAN_POINT('Ctrl Pts',(3.30884480305537,-3.,12.2938762651102));
#17980=CARTESIAN_POINT('Ctrl Pts',(3.30884480305537,4.2,12.2938762651102));
#17981=CARTESIAN_POINT('Ctrl Pts',(3.48993681214337,-3.,12.2723364229612));
#17982=CARTESIAN_POINT('Ctrl Pts',(3.48993681214337,4.2,12.2723364229612));
#17983=CARTESIAN_POINT('Ctrl Pts',(3.64927048315907,-3.,12.2301117722792));
#17984=CARTESIAN_POINT('Ctrl Pts',(3.64927048315907,4.2,12.2301117722792));
#17985=CARTESIAN_POINT('Ctrl Pts',(3.79241297762162,-3.,12.1626050652587));
#17986=CARTESIAN_POINT('Ctrl Pts',(3.79241297762162,4.2,12.1626050652587));
#17987=CARTESIAN_POINT('Ctrl Pts',(3.92533033057351,-3.,12.0684942936878));
#17988=CARTESIAN_POINT('Ctrl Pts',(3.92533033057351,4.2,12.0684942936878));
#17989=CARTESIAN_POINT('Ctrl Pts',(4.05395481372655,-3.,11.9514202619535));
#17990=CARTESIAN_POINT('Ctrl Pts',(4.05395481372655,4.2,11.9514202619535));
#17991=CARTESIAN_POINT('Ctrl Pts',(4.18369962429796,-3.,11.8183570873731));
#17992=CARTESIAN_POINT('Ctrl Pts',(4.18369962429796,4.2,11.8183570873731));
#17993=CARTESIAN_POINT('Ctrl Pts',(4.3189358499924,-3.,11.67764924636));
#17994=CARTESIAN_POINT('Ctrl Pts',(4.3189358499924,4.2,11.67764924636));
#17995=CARTESIAN_POINT('Ctrl Pts',(4.46255574628753,-3.,11.5373242211525));
#17996=CARTESIAN_POINT('Ctrl Pts',(4.46255574628753,4.2,11.5373242211525));
#17997=CARTESIAN_POINT('Ctrl Pts',(4.61532593596939,-3.,11.4029224160728));
#17998=CARTESIAN_POINT('Ctrl Pts',(4.61532593596939,4.2,11.4029224160728));
#17999=CARTESIAN_POINT('Ctrl Pts',(4.77596612414944,-3.,11.2768795166233));
#18000=CARTESIAN_POINT('Ctrl Pts',(4.77596612414944,4.2,11.2768795166233));
#18001=CARTESIAN_POINT('Ctrl Pts',(4.94211773226968,-3.,11.1598106424589));
#18002=CARTESIAN_POINT('Ctrl Pts',(4.94211773226968,4.2,11.1598106424589));
#18003=CARTESIAN_POINT('Ctrl Pts',(5.11112998264613,-3.,11.051370419133));
#18004=CARTESIAN_POINT('Ctrl Pts',(5.11112998264613,4.2,11.051370419133));
#18005=CARTESIAN_POINT('Ctrl Pts',(5.28082876351925,-3.,10.9511663773825));
#18006=CARTESIAN_POINT('Ctrl Pts',(5.28082876351925,4.2,10.9511663773825));
#18007=CARTESIAN_POINT('Ctrl Pts',(5.45051506148977,-3.,10.8599381259735));
#18008=CARTESIAN_POINT('Ctrl Pts',(5.45051506148977,4.2,10.8599381259735));
#18009=CARTESIAN_POINT('Ctrl Pts',(5.62101499943423,-3.,10.7795199127532));
#18010=CARTESIAN_POINT('Ctrl Pts',(5.62101499943423,4.2,10.7795199127532));
#18011=CARTESIAN_POINT('Ctrl Pts',(5.7936769541502,-3.,10.7114411549111));
#18012=CARTESIAN_POINT('Ctrl Pts',(5.7936769541502,4.2,10.7114411549111));
#18013=CARTESIAN_POINT('Ctrl Pts',(5.96961932707136,-3.,10.6558377434042));
#18014=CARTESIAN_POINT('Ctrl Pts',(5.96961932707136,4.2,10.6558377434042));
#18015=CARTESIAN_POINT('Ctrl Pts',(6.14893768388704,-3.,10.6103475969888));
#18016=CARTESIAN_POINT('Ctrl Pts',(6.14893768388704,4.2,10.6103475969888));
#18017=CARTESIAN_POINT('Ctrl Pts',(6.32976796473819,-3.,10.5687216653907));
#18018=CARTESIAN_POINT('Ctrl Pts',(6.32976796473819,4.2,10.5687216653907));
#18019=CARTESIAN_POINT('Ctrl Pts',(6.50892555577775,-3.,10.5222908830264));
#18020=CARTESIAN_POINT('Ctrl Pts',(6.50892555577775,4.2,10.5222908830264));
#18021=CARTESIAN_POINT('Ctrl Pts',(6.68288828293941,-3.,10.462050267878));
#18022=CARTESIAN_POINT('Ctrl Pts',(6.68288828293941,4.2,10.462050267878));
#18023=CARTESIAN_POINT('Ctrl Pts',(6.84859008776107,-3.,10.3804015453596));
#18024=CARTESIAN_POINT('Ctrl Pts',(6.84859008776107,4.2,10.3804015453596));
#18025=CARTESIAN_POINT('Ctrl Pts',(7.00445448641038,-3.,10.2733319413005));
#18026=CARTESIAN_POINT('Ctrl Pts',(7.00445448641038,4.2,10.2733319413005));
#18027=CARTESIAN_POINT('Ctrl Pts',(7.15081550722288,-3.,10.1414720974144));
#18028=CARTESIAN_POINT('Ctrl Pts',(7.15081550722288,4.2,10.1414720974144));
#18029=CARTESIAN_POINT('Ctrl Pts',(7.28883796912684,-3.,9.98835756998534));
#18030=CARTESIAN_POINT('Ctrl Pts',(7.28883796912684,4.2,9.98835756998534));
#18031=CARTESIAN_POINT('Ctrl Pts',(7.41967047354988,-3.,9.81917361987377));
#18032=CARTESIAN_POINT('Ctrl Pts',(7.41967047354988,4.2,9.81917361987377));
#18033=CARTESIAN_POINT('Ctrl Pts',(7.54360573526532,-3.,9.63939026966049));
#18034=CARTESIAN_POINT('Ctrl Pts',(7.54360573526532,4.2,9.63939026966049));
#18035=CARTESIAN_POINT('Ctrl Pts',(7.6590003866074,-3.,9.45324999450471));
#18036=CARTESIAN_POINT('Ctrl Pts',(7.6590003866074,4.2,9.45324999450471));
#18037=CARTESIAN_POINT('Ctrl Pts',(7.76209282457502,-3.,9.26297089919836));
#18038=CARTESIAN_POINT('Ctrl Pts',(7.76209282457502,4.2,9.26297089919836));
#18039=CARTESIAN_POINT('Ctrl Pts',(7.84862074946283,-3.,9.06945407017055));
#18040=CARTESIAN_POINT('Ctrl Pts',(7.84862074946283,4.2,9.06945407017055));
#18041=CARTESIAN_POINT('Ctrl Pts',(7.91508259073031,-3.,8.87266947141857));
#18042=CARTESIAN_POINT('Ctrl Pts',(7.91508259073031,4.2,8.87266947141857));
#18043=CARTESIAN_POINT('Ctrl Pts',(7.96007609558387,-3.,8.67216210283894));
#18044=CARTESIAN_POINT('Ctrl Pts',(7.96007609558387,4.2,8.67216210283894));
#18045=CARTESIAN_POINT('Ctrl Pts',(7.98575825096082,-3.,8.46752658699496));
#18046=CARTESIAN_POINT('Ctrl Pts',(7.98575825096082,4.2,8.46752658699496));
#18047=CARTESIAN_POINT('Ctrl Pts',(7.9987984391963,-3.,8.25883677791438));
#18048=CARTESIAN_POINT('Ctrl Pts',(7.9987984391963,4.2,8.25883677791438));
#18049=CARTESIAN_POINT('Ctrl Pts',(8.00781893805568,-3.,8.04662057355209));
#18050=CARTESIAN_POINT('Ctrl Pts',(8.00781893805568,4.2,8.04662057355209));
#18051=CARTESIAN_POINT('Ctrl Pts',(8.02124364536257,-3.,7.8318867323277));
#18052=CARTESIAN_POINT('Ctrl Pts',(8.02124364536257,4.2,7.8318867323277));
#18053=CARTESIAN_POINT('Ctrl Pts',(8.04494633492827,-3.,7.61613341658679));
#18054=CARTESIAN_POINT('Ctrl Pts',(8.04494633492827,4.2,7.61613341658679));
#18055=CARTESIAN_POINT('Ctrl Pts',(8.08008348678094,-3.,7.40136016279815));
#18056=CARTESIAN_POINT('Ctrl Pts',(8.08008348678094,4.2,7.40136016279815));
#18057=CARTESIAN_POINT('Ctrl Pts',(8.12057943633426,-3.,7.19009032473197));
#18058=CARTESIAN_POINT('Ctrl Pts',(8.12057943633426,4.2,7.19009032473197));
#18059=CARTESIAN_POINT('Ctrl Pts',(8.15569042861283,-3.,6.98516923427904));
#18060=CARTESIAN_POINT('Ctrl Pts',(8.15569042861283,4.2,6.98516923427904));
#18061=CARTESIAN_POINT('Ctrl Pts',(8.17293082304204,-3.,6.78954489191915));
#18062=CARTESIAN_POINT('Ctrl Pts',(8.17293082304204,4.2,6.78954489191915));
#18063=CARTESIAN_POINT('Ctrl Pts',(8.16089752265956,-3.,6.60605451948904));
#18064=CARTESIAN_POINT('Ctrl Pts',(8.16089752265956,4.2,6.60605451948904));
#18065=CARTESIAN_POINT('Ctrl Pts',(8.11207116917844,-3.,6.43720976255638));
#18066=CARTESIAN_POINT('Ctrl Pts',(8.11207116917844,4.2,6.43720976255638));
#18067=CARTESIAN_POINT('Ctrl Pts',(8.02580908828092,-3.,6.28498018271691));
#18068=CARTESIAN_POINT('Ctrl Pts',(8.02580908828092,4.2,6.28498018271691));
#18069=CARTESIAN_POINT('Ctrl Pts',(7.90644860448881,-3.,6.15052660592943));
#18070=CARTESIAN_POINT('Ctrl Pts',(7.90644860448881,4.2,6.15052660592943));
#18071=CARTESIAN_POINT('Ctrl Pts',(7.76106756457749,-3.,6.03389995867286));
#18072=CARTESIAN_POINT('Ctrl Pts',(7.76106756457749,4.2,6.03389995867286));
#18073=CARTESIAN_POINT('Ctrl Pts',(7.59751903688427,-3.,5.93381436957244));
#18074=CARTESIAN_POINT('Ctrl Pts',(7.59751903688427,4.2,5.93381436957244));
#18075=CARTESIAN_POINT('Ctrl Pts',(7.42198551710643,-3.,5.84723737025948));
#18076=CARTESIAN_POINT('Ctrl Pts',(7.42198551710643,4.2,5.84723737025948));
#18077=CARTESIAN_POINT('Ctrl Pts',(7.23853768475023,-3.,5.76979878895671));
#18078=CARTESIAN_POINT('Ctrl Pts',(7.23853768475023,4.2,5.76979878895671));
#18079=CARTESIAN_POINT('Ctrl Pts',(7.04976847947264,-3.,5.69662713609756));
#18080=CARTESIAN_POINT('Ctrl Pts',(7.04976847947264,4.2,5.69662713609756));
#18081=CARTESIAN_POINT('Ctrl Pts',(6.85709976037512,-3.,5.62308582598972));
#18082=CARTESIAN_POINT('Ctrl Pts',(6.85709976037512,4.2,5.62308582598972));
#18083=CARTESIAN_POINT('Ctrl Pts',(6.66121503090593,-3.,5.54547963906641));
#18084=CARTESIAN_POINT('Ctrl Pts',(6.66121503090593,4.2,5.54547963906641));
#18085=CARTESIAN_POINT('Ctrl Pts',(6.46246210121974,-3.,5.46195513100458));
#18086=CARTESIAN_POINT('Ctrl Pts',(6.46246210121974,4.2,5.46195513100458));
#18087=CARTESIAN_POINT('Ctrl Pts',(6.26112587698791,-3.,5.37226655127806));
#18088=CARTESIAN_POINT('Ctrl Pts',(6.26112587698791,4.2,5.37226655127806));
#18089=CARTESIAN_POINT('Ctrl Pts',(6.05762450882876,-3.,5.27709955371581));
#18090=CARTESIAN_POINT('Ctrl Pts',(6.05762450882876,4.2,5.27709955371581));
#18091=CARTESIAN_POINT('Ctrl Pts',(5.85274048349253,-3.,5.17752467829117));
#18092=CARTESIAN_POINT('Ctrl Pts',(5.85274048349253,4.2,5.17752467829117));
#18093=CARTESIAN_POINT('Ctrl Pts',(5.6478173738032,-3.,5.07442896098936));
#18094=CARTESIAN_POINT('Ctrl Pts',(5.6478173738032,4.2,5.07442896098936));
#18095=CARTESIAN_POINT('Ctrl Pts',(5.44501860313336,-3.,4.96787993373722));
#18096=CARTESIAN_POINT('Ctrl Pts',(5.44501860313336,4.2,4.96787993373722));
#18097=CARTESIAN_POINT('Ctrl Pts',(5.24741086000008,-3.,4.85676111532844));
#18098=CARTESIAN_POINT('Ctrl Pts',(5.24741086000008,4.2,4.85676111532844));
#18099=CARTESIAN_POINT('Ctrl Pts',(5.05850630701875,-3.,4.73929437247794));
#18100=CARTESIAN_POINT('Ctrl Pts',(5.05850630701875,4.2,4.73929437247794));
#18101=CARTESIAN_POINT('Ctrl Pts',(4.88190185104846,-3.,4.61340315498245));
#18102=CARTESIAN_POINT('Ctrl Pts',(4.88190185104846,4.2,4.61340315498245));
#18103=CARTESIAN_POINT('Ctrl Pts',(4.7208720035032,-3.,4.47714872481864));
#18104=CARTESIAN_POINT('Ctrl Pts',(4.7208720035032,4.2,4.47714872481864));
#18105=CARTESIAN_POINT('Ctrl Pts',(4.57800047823784,-3.,4.32911151507775));
#18106=CARTESIAN_POINT('Ctrl Pts',(4.57800047823784,4.2,4.32911151507775));
#18107=CARTESIAN_POINT('Ctrl Pts',(4.4547451964031,-3.,4.16885849319143));
#18108=CARTESIAN_POINT('Ctrl Pts',(4.4547451964031,4.2,4.16885849319143));
#18109=CARTESIAN_POINT('Ctrl Pts',(4.35148411330737,-3.,3.99681013615577));
#18110=CARTESIAN_POINT('Ctrl Pts',(4.35148411330737,4.2,3.99681013615577));
#18111=CARTESIAN_POINT('Ctrl Pts',(4.26765207024408,-3.,3.81399668859083));
#18112=CARTESIAN_POINT('Ctrl Pts',(4.26765207024408,4.2,3.81399668859083));
#18113=CARTESIAN_POINT('Ctrl Pts',(4.20184334854117,-3.,3.62185203209172));
#18114=CARTESIAN_POINT('Ctrl Pts',(4.20184334854117,4.2,3.62185203209172));
#18115=CARTESIAN_POINT('Ctrl Pts',(4.15193466045737,-3.,3.42199345348454));
#18116=CARTESIAN_POINT('Ctrl Pts',(4.15193466045737,4.2,3.42199345348454));
#18117=CARTESIAN_POINT('Ctrl Pts',(4.11518318246501,-3.,3.21600287470933));
#18118=CARTESIAN_POINT('Ctrl Pts',(4.11518318246501,4.2,3.21600287470933));
#18119=CARTESIAN_POINT('Ctrl Pts',(4.08854433447712,-3.,3.00529120729351));
#18120=CARTESIAN_POINT('Ctrl Pts',(4.08854433447712,4.2,3.00529120729351));
#18121=CARTESIAN_POINT('Ctrl Pts',(4.06899962712481,-3.,2.7909834104826));
#18122=CARTESIAN_POINT('Ctrl Pts',(4.06899962712481,4.2,2.7909834104826));
#18123=CARTESIAN_POINT('Ctrl Pts',(4.05390260344518,-3.,2.57377631141663));
#18124=CARTESIAN_POINT('Ctrl Pts',(4.05390260344518,4.2,2.57377631141663));
#18125=CARTESIAN_POINT('Ctrl Pts',(4.04126813644791,-3.,2.35385258470204));
#18126=CARTESIAN_POINT('Ctrl Pts',(4.04126813644791,4.2,2.35385258470204));
#18127=CARTESIAN_POINT('Ctrl Pts',(4.03021014446877,-3.,2.13065748555701));
#18128=CARTESIAN_POINT('Ctrl Pts',(4.03021014446877,4.2,2.13065748555701));
#18129=CARTESIAN_POINT('Ctrl Pts',(4.02066709528519,-3.,1.9033255681334));
#18130=CARTESIAN_POINT('Ctrl Pts',(4.02066709528519,4.2,1.9033255681334));
#18131=CARTESIAN_POINT('Ctrl Pts',(4.012782399266,-3.,1.67142113207676));
#18132=CARTESIAN_POINT('Ctrl Pts',(4.012782399266,4.2,1.67142113207676));
#18133=CARTESIAN_POINT('Ctrl Pts',(4.00639322616619,-3.,1.4355810193293));
#18134=CARTESIAN_POINT('Ctrl Pts',(4.00639322616619,4.2,1.4355810193293));
#18135=CARTESIAN_POINT('Ctrl Pts',(4.00047520099043,-3.,1.19819542279832));
#18136=CARTESIAN_POINT('Ctrl Pts',(4.00047520099043,4.2,1.19819542279832));
#18137=CARTESIAN_POINT('Ctrl Pts',(3.99260375067002,-3.,0.964078729991153));
#18138=CARTESIAN_POINT('Ctrl Pts',(3.99260375067002,4.2,0.964078729991153));
#18139=CARTESIAN_POINT('Ctrl Pts',(3.97841403016118,-3.,0.741129277895168));
#18140=CARTESIAN_POINT('Ctrl Pts',(3.97841403016118,4.2,0.741129277895168));
#18141=CARTESIAN_POINT('Ctrl Pts',(3.95259200169988,-3.,0.538436816836329));
#18142=CARTESIAN_POINT('Ctrl Pts',(3.95259200169988,4.2,0.538436816836329));
#18143=CARTESIAN_POINT('Ctrl Pts',(3.90986572419832,-3.,0.364350357241537));
#18144=CARTESIAN_POINT('Ctrl Pts',(3.90986572419832,4.2,0.364350357241537));
#18145=CARTESIAN_POINT('Ctrl Pts',(3.84598208672298,-3.,0.224659532804428));
#18146=CARTESIAN_POINT('Ctrl Pts',(3.84598208672298,4.2,0.224659532804428));
#18147=CARTESIAN_POINT('Ctrl Pts',(3.75872318140661,-3.,0.120497232333236));
#18148=CARTESIAN_POINT('Ctrl Pts',(3.75872318140661,4.2,0.120497232333236));
#18149=CARTESIAN_POINT('Ctrl Pts',(3.64881642260075,-3.,0.0470540298718229));
#18150=CARTESIAN_POINT('Ctrl Pts',(3.64881642260075,4.2,0.0470540298718229));
#18151=CARTESIAN_POINT('Ctrl Pts',(3.52045328348988,-3.,-0.00118366394786523));
#18152=CARTESIAN_POINT('Ctrl Pts',(3.52045328348988,4.2,-0.00118366394786523));
#18153=CARTESIAN_POINT('Ctrl Pts',(3.3816469894381,-3.,-0.0263068037111615));
#18154=CARTESIAN_POINT('Ctrl Pts',(3.3816469894381,4.2,-0.0263068037111615));
#18155=CARTESIAN_POINT('Ctrl Pts',(3.2451100102617,-3.,-0.0214179570895094));
#18156=CARTESIAN_POINT('Ctrl Pts',(3.2451100102617,4.2,-0.0214179570895094));
#18157=CARTESIAN_POINT('Ctrl Pts',(3.12452733970665,-3.,0.0241851999814078));
#18158=CARTESIAN_POINT('Ctrl Pts',(3.12452733970665,4.2,0.0241851999814078));
#18159=CARTESIAN_POINT('Ctrl Pts',(3.03063129752059,-3.,0.119017371327004));
#18160=CARTESIAN_POINT('Ctrl Pts',(3.03063129752059,4.2,0.119017371327004));
#18161=CARTESIAN_POINT('Ctrl Pts',(2.96639254265844,-3.,0.262319630540593));
#18162=CARTESIAN_POINT('Ctrl Pts',(2.96639254265844,4.2,0.262319630540593));
#18163=CARTESIAN_POINT('Ctrl Pts',(2.92780415844446,-3.,0.444963858672424));
#18164=CARTESIAN_POINT('Ctrl Pts',(2.92780415844446,4.2,0.444963858672424));
#18165=CARTESIAN_POINT('Ctrl Pts',(2.90717911786689,-3.,0.65402023086958));
#18166=CARTESIAN_POINT('Ctrl Pts',(2.90717911786689,4.2,0.65402023086958));
#18167=CARTESIAN_POINT('Ctrl Pts',(2.89547076625581,-3.,0.875890304828918));
#18168=CARTESIAN_POINT('Ctrl Pts',(2.89547076625581,4.2,0.875890304828918));
#18169=CARTESIAN_POINT('Ctrl Pts',(2.88537704766906,-3.,1.10060381648398));
#18170=CARTESIAN_POINT('Ctrl Pts',(2.88537704766906,4.2,1.10060381648398));
#18171=CARTESIAN_POINT('Ctrl Pts',(2.8728456296504,-3.,1.32371934078733));
#18172=CARTESIAN_POINT('Ctrl Pts',(2.8728456296504,4.2,1.32371934078733));
#18173=CARTESIAN_POINT('Ctrl Pts',(2.85578261679345,-3.,1.54401727992264));
#18174=CARTESIAN_POINT('Ctrl Pts',(2.85578261679345,4.2,1.54401727992264));
#18175=CARTESIAN_POINT('Ctrl Pts',(2.83335686249019,-3.,1.76209503442146));
#18176=CARTESIAN_POINT('Ctrl Pts',(2.83335686249019,4.2,1.76209503442146));
#18177=CARTESIAN_POINT('Ctrl Pts',(2.80505146480345,-3.,1.97856787413951));
#18178=CARTESIAN_POINT('Ctrl Pts',(2.80505146480345,4.2,1.97856787413951));
#18179=CARTESIAN_POINT('Ctrl Pts',(2.76985908233915,-3.,2.19251877196071));
#18180=CARTESIAN_POINT('Ctrl Pts',(2.76985908233915,4.2,2.19251877196071));
#18181=CARTESIAN_POINT('Ctrl Pts',(2.72531955636536,-3.,2.39962532458029));
#18182=CARTESIAN_POINT('Ctrl Pts',(2.72531955636536,4.2,2.39962532458029));
#18183=CARTESIAN_POINT('Ctrl Pts',(2.66797634363184,-3.,2.59347738935741));
#18184=CARTESIAN_POINT('Ctrl Pts',(2.66797634363184,4.2,2.59347738935741));
#18185=CARTESIAN_POINT('Ctrl Pts',(2.59397540849171,-3.,2.7672283971178));
#18186=CARTESIAN_POINT('Ctrl Pts',(2.59397540849171,4.2,2.7672283971178));
#18187=CARTESIAN_POINT('Ctrl Pts',(2.49960870420485,-3.,2.91510580081997));
#18188=CARTESIAN_POINT('Ctrl Pts',(2.49960870420485,4.2,2.91510580081997));
#18189=CARTESIAN_POINT('Ctrl Pts',(2.38189256086504,-3.,3.03403241435618));
#18190=CARTESIAN_POINT('Ctrl Pts',(2.38189256086504,4.2,3.03403241435618));
#18191=CARTESIAN_POINT('Ctrl Pts',(2.23909845280558,-3.,3.12505646843308));
#18192=CARTESIAN_POINT('Ctrl Pts',(2.23909845280558,4.2,3.12505646843308));
#18193=CARTESIAN_POINT('Ctrl Pts',(2.07061055216582,-3.,3.19196918412265));
#18194=CARTESIAN_POINT('Ctrl Pts',(2.07061055216582,4.2,3.19196918412265));
#18195=CARTESIAN_POINT('Ctrl Pts',(1.87681490437036,-3.,3.24001322621211));
#18196=CARTESIAN_POINT('Ctrl Pts',(1.87681490437036,4.2,3.24001322621211));
#18197=CARTESIAN_POINT('Ctrl Pts',(1.65897747541321,-3.,3.27464765209773));
#18198=CARTESIAN_POINT('Ctrl Pts',(1.65897747541321,4.2,3.27464765209773));
#18199=CARTESIAN_POINT('Ctrl Pts',(1.4191255439272,-3.,3.30006519349576));
#18200=CARTESIAN_POINT('Ctrl Pts',(1.4191255439272,4.2,3.30006519349576));
#18201=CARTESIAN_POINT('Ctrl Pts',(1.15993538533448,-3.,3.31897283641381));
#18202=CARTESIAN_POINT('Ctrl Pts',(1.15993538533448,4.2,3.31897283641381));
#18203=CARTESIAN_POINT('Ctrl Pts',(0.884625090385968,-3.,3.33300441174764));
#18204=CARTESIAN_POINT('Ctrl Pts',(0.884625090385968,4.2,3.33300441174764));
#18205=CARTESIAN_POINT('Ctrl Pts',(0.596845720618978,-3.,3.34293392264922));
#18206=CARTESIAN_POINT('Ctrl Pts',(0.596845720618978,4.2,3.34293392264922));
#18207=CARTESIAN_POINT('Ctrl Pts',(0.30057321210183,-3.,3.34897162637417));
#18208=CARTESIAN_POINT('Ctrl Pts',(0.30057321210183,4.2,3.34897162637417));
#18209=CARTESIAN_POINT('Ctrl Pts',(1.66741620510891E-14,-3.,3.35102435732185));
#18210=CARTESIAN_POINT('Ctrl Pts',(1.66741620510891E-14,4.2,3.35102435732185));
#18211=CARTESIAN_POINT('Ctrl Pts',(-0.300573212101791,-3.,3.34897162637426));
#18212=CARTESIAN_POINT('Ctrl Pts',(-0.300573212101791,4.2,3.34897162637426));
#18213=CARTESIAN_POINT('Ctrl Pts',(-0.596845720618908,-3.,3.34293392264938));
#18214=CARTESIAN_POINT('Ctrl Pts',(-0.596845720618908,4.2,3.34293392264938));
#18215=CARTESIAN_POINT('Ctrl Pts',(-0.884625090385886,-3.,3.33300441174785));
#18216=CARTESIAN_POINT('Ctrl Pts',(-0.884625090385886,4.2,3.33300441174785));
#18217=CARTESIAN_POINT('Ctrl Pts',(-1.15993538533442,-3.,3.31897283641402));
#18218=CARTESIAN_POINT('Ctrl Pts',(-1.15993538533442,4.2,3.31897283641402));
#18219=CARTESIAN_POINT('Ctrl Pts',(-1.41912554392716,-3.,3.30006519349591));
#18220=CARTESIAN_POINT('Ctrl Pts',(-1.41912554392716,4.2,3.30006519349591));
#18221=CARTESIAN_POINT('Ctrl Pts',(-1.65897747541319,-3.,3.27464765209779));
#18222=CARTESIAN_POINT('Ctrl Pts',(-1.65897747541319,4.2,3.27464765209779));
#18223=CARTESIAN_POINT('Ctrl Pts',(-1.87681490437034,-3.,3.24001322621208));
#18224=CARTESIAN_POINT('Ctrl Pts',(-1.87681490437034,4.2,3.24001322621208));
#18225=CARTESIAN_POINT('Ctrl Pts',(-2.07061055216576,-3.,3.19196918412254));
#18226=CARTESIAN_POINT('Ctrl Pts',(-2.07061055216576,4.2,3.19196918412254));
#18227=CARTESIAN_POINT('Ctrl Pts',(-2.23909845280547,-3.,3.12505646843295));
#18228=CARTESIAN_POINT('Ctrl Pts',(-2.23909845280547,4.2,3.12505646843295));
#18229=CARTESIAN_POINT('Ctrl Pts',(-2.38189256086493,-3.,3.03403241435609));
#18230=CARTESIAN_POINT('Ctrl Pts',(-2.38189256086493,4.2,3.03403241435609));
#18231=CARTESIAN_POINT('Ctrl Pts',(-2.49960870420481,-3.,2.91510580081997));
#18232=CARTESIAN_POINT('Ctrl Pts',(-2.49960870420481,4.2,2.91510580081997));
#18233=CARTESIAN_POINT('Ctrl Pts',(-2.59397540849182,-3.,2.76722839711793));
#18234=CARTESIAN_POINT('Ctrl Pts',(-2.59397540849182,4.2,2.76722839711793));
#18235=CARTESIAN_POINT('Ctrl Pts',(-2.66797634363209,-3.,2.59347738935767));
#18236=CARTESIAN_POINT('Ctrl Pts',(-2.66797634363209,4.2,2.59347738935767));
#18237=CARTESIAN_POINT('Ctrl Pts',(-2.72531955636566,-3.,2.39962532458057));
#18238=CARTESIAN_POINT('Ctrl Pts',(-2.72531955636566,4.2,2.39962532458057));
#18239=CARTESIAN_POINT('Ctrl Pts',(-2.76985908233936,-3.,2.19251877196088));
#18240=CARTESIAN_POINT('Ctrl Pts',(-2.76985908233936,4.2,2.19251877196088));
#18241=CARTESIAN_POINT('Ctrl Pts',(-2.80505146480344,-3.,1.97856787413951));
#18242=CARTESIAN_POINT('Ctrl Pts',(-2.80505146480344,4.2,1.97856787413951));
#18243=CARTESIAN_POINT('Ctrl Pts',(-2.8333568624899,-3.,1.76209503442131));
#18244=CARTESIAN_POINT('Ctrl Pts',(-2.8333568624899,4.2,1.76209503442131));
#18245=CARTESIAN_POINT('Ctrl Pts',(-2.85578261679294,-3.,1.54401727992238));
#18246=CARTESIAN_POINT('Ctrl Pts',(-2.85578261679294,4.2,1.54401727992238));
#18247=CARTESIAN_POINT('Ctrl Pts',(-2.87284562964987,-3.,1.32371934078708));
#18248=CARTESIAN_POINT('Ctrl Pts',(-2.87284562964987,4.2,1.32371934078708));
#18249=CARTESIAN_POINT('Ctrl Pts',(-2.88537704766869,-3.,1.10060381648384));
#18250=CARTESIAN_POINT('Ctrl Pts',(-2.88537704766869,4.2,1.10060381648384));
#18251=CARTESIAN_POINT('Ctrl Pts',(-2.89547076625573,-3.,0.875890304828914));
#18252=CARTESIAN_POINT('Ctrl Pts',(-2.89547076625573,4.2,0.875890304828914));
#18253=CARTESIAN_POINT('Ctrl Pts',(-2.90717911786707,-3.,0.654020230869684));
#18254=CARTESIAN_POINT('Ctrl Pts',(-2.90717911786707,4.2,0.654020230869684));
#18255=CARTESIAN_POINT('Ctrl Pts',(-2.92780415844476,-3.,0.444963858672577));
#18256=CARTESIAN_POINT('Ctrl Pts',(-2.92780415844476,4.2,0.444963858672577));
#18257=CARTESIAN_POINT('Ctrl Pts',(-2.96639254265869,-3.,0.262319630540737));
#18258=CARTESIAN_POINT('Ctrl Pts',(-2.96639254265869,4.2,0.262319630540737));
#18259=CARTESIAN_POINT('Ctrl Pts',(-3.03063129752067,-3.,0.11901737132707));
#18260=CARTESIAN_POINT('Ctrl Pts',(-3.03063129752067,4.2,0.11901737132707));
#18261=CARTESIAN_POINT('Ctrl Pts',(-3.12452733970658,-3.,0.0241851999813871));
#18262=CARTESIAN_POINT('Ctrl Pts',(-3.12452733970658,4.2,0.0241851999813871));
#18263=CARTESIAN_POINT('Ctrl Pts',(-3.24511001026157,-3.,-0.0214179570895714));
#18264=CARTESIAN_POINT('Ctrl Pts',(-3.24511001026157,4.2,-0.0214179570895714));
#18265=CARTESIAN_POINT('Ctrl Pts',(-3.38164698943802,-3.,-0.0263068037112043));
#18266=CARTESIAN_POINT('Ctrl Pts',(-3.38164698943802,4.2,-0.0263068037112043));
#18267=CARTESIAN_POINT('Ctrl Pts',(-3.52045328348989,-3.,-0.00118366394785932));
#18268=CARTESIAN_POINT('Ctrl Pts',(-3.52045328348989,4.2,-0.00118366394785932));
#18269=CARTESIAN_POINT('Ctrl Pts',(-3.64881642260079,-3.,0.0470540298718583));
#18270=CARTESIAN_POINT('Ctrl Pts',(-3.64881642260079,4.2,0.0470540298718583));
#18271=CARTESIAN_POINT('Ctrl Pts',(-3.75872318140663,-3.,0.120497232333251));
#18272=CARTESIAN_POINT('Ctrl Pts',(-3.75872318140663,4.2,0.120497232333251));
#18273=CARTESIAN_POINT('Ctrl Pts',(-3.84598208672296,-3.,0.224659532804408));
#18274=CARTESIAN_POINT('Ctrl Pts',(-3.84598208672296,4.2,0.224659532804408));
#18275=CARTESIAN_POINT('Ctrl Pts',(-3.9098657241983,-3.,0.364350357241515));
#18276=CARTESIAN_POINT('Ctrl Pts',(-3.9098657241983,4.2,0.364350357241515));
#18277=CARTESIAN_POINT('Ctrl Pts',(-3.9525920016999,-3.,0.538436816836325));
#18278=CARTESIAN_POINT('Ctrl Pts',(-3.9525920016999,4.2,0.538436816836325));
#18279=CARTESIAN_POINT('Ctrl Pts',(-3.97841403016126,-3.,0.741129277895169));
#18280=CARTESIAN_POINT('Ctrl Pts',(-3.97841403016126,4.2,0.741129277895169));
#18281=CARTESIAN_POINT('Ctrl Pts',(-3.99260375067011,-3.,0.964078729991154));
#18282=CARTESIAN_POINT('Ctrl Pts',(-3.99260375067011,4.2,0.964078729991154));
#18283=CARTESIAN_POINT('Ctrl Pts',(-4.00047520099045,-3.,1.1981954227983));
#18284=CARTESIAN_POINT('Ctrl Pts',(-4.00047520099045,4.2,1.1981954227983));
#18285=CARTESIAN_POINT('Ctrl Pts',(-4.00639322616607,-3.,1.43558101932923));
#18286=CARTESIAN_POINT('Ctrl Pts',(-4.00639322616607,4.2,1.43558101932923));
#18287=CARTESIAN_POINT('Ctrl Pts',(-4.01278239926574,-3.,1.67142113207667));
#18288=CARTESIAN_POINT('Ctrl Pts',(-4.01278239926574,4.2,1.67142113207667));
#18289=CARTESIAN_POINT('Ctrl Pts',(-4.02066709528487,-3.,1.90332556813333));
#18290=CARTESIAN_POINT('Ctrl Pts',(-4.02066709528487,4.2,1.90332556813333));
#18291=CARTESIAN_POINT('Ctrl Pts',(-4.0302101444685,-3.,2.130657485557));
#18292=CARTESIAN_POINT('Ctrl Pts',(-4.0302101444685,4.2,2.130657485557));
#18293=CARTESIAN_POINT('Ctrl Pts',(-4.04126813644779,-3.,2.35385258470204));
#18294=CARTESIAN_POINT('Ctrl Pts',(-4.04126813644779,4.2,2.35385258470204));
#18295=CARTESIAN_POINT('Ctrl Pts',(-4.05237622399436,-3.,2.5472071607522));
#18296=CARTESIAN_POINT('Ctrl Pts',(-4.05237622399436,4.2,2.5472071607522));
#18297=CARTESIAN_POINT('Ctrl Pts',(-4.0623773838412,-3.,2.69501052271264));
#18298=CARTESIAN_POINT('Ctrl Pts',(-4.0623773838412,4.2,2.69501052271264));
#18299=CARTESIAN_POINT('Ctrl Pts',(-4.07059539687633,-3.,2.79846879209956));
#18300=CARTESIAN_POINT('Ctrl Pts',(-4.07059539687633,4.2,2.79846879209956));
#18301=CARTESIAN_POINT('Ctrl Pts',(-4.07588877936474,-3.,2.85844305779059));
#18302=CARTESIAN_POINT('Ctrl Pts',(-4.07588877936474,4.2,2.85844305779059));
#18303=CARTESIAN_POINT('Ctrl Pts',(-4.07743349288644,-3.,2.87542908850901));
#18304=CARTESIAN_POINT('Ctrl Pts',(-4.07743349288644,4.2,2.87542908850901));
#18305=CARTESIAN_POINT('Ctrl Pts',(-4.26562934894771,0.281862854502613,
3.79515655425571));
#18306=CARTESIAN_POINT('Ctrl Pts',(-4.28076756904347,0.225365966174025,
3.83396390718086));
#18307=CARTESIAN_POINT('Ctrl Pts',(-4.29636831527147,0.167143869993732,
3.87046814413346));
#18308=CARTESIAN_POINT('Ctrl Pts',(-4.31223161698407,0.107940822442962,
3.90484829258838));
#18309=CARTESIAN_POINT('Ctrl Pts',(-4.20352761804101,0.513629669484374,
3.61216526483895));
#18310=CARTESIAN_POINT('Ctrl Pts',(-4.17637358974273,0.506353769530596,
3.51942422402296));
#18311=CARTESIAN_POINT('Ctrl Pts',(-4.1544631012454,0.503326431198334,3.42375049497737));
#18312=CARTESIAN_POINT('Ctrl Pts',(-4.12235794997748,0.500363612845377,
3.2498423204338));
#18313=CARTESIAN_POINT('Ctrl Pts',(-4.11054280568554,0.500016016851208,
3.17079826924657));
#18314=CARTESIAN_POINT('Ctrl Pts',(-4.10062628985476,0.500000490299028,
3.09201395473891));
#18315=CARTESIAN_POINT('Ctrl Pts',(4.03928538163603,0.5,2.62055334362004));
#18316=CARTESIAN_POINT('Ctrl Pts',(4.04632311223308,0.5,2.71168199850908));
#18317=CARTESIAN_POINT('Ctrl Pts',(4.05429381417606,0.5,2.80274587021811));
#18318=CARTESIAN_POINT('Ctrl Pts',(4.06419081564702,0.5,2.89360843325953));
#18319=CARTESIAN_POINT('Ctrl Pts',(4.04946587537915,0.5,2.61976711921679));
#18320=CARTESIAN_POINT('Ctrl Pts',(4.05599586658109,0.499999012141377,2.71086143217845));
#18321=CARTESIAN_POINT('Ctrl Pts',(4.06337743637285,0.500000842758452,2.8018781295488));
#18322=CARTESIAN_POINT('Ctrl Pts',(4.07248440131376,0.5,2.89270507298886));
#18323=CARTESIAN_POINT('Ctrl Pts',(4.05964274711213,0.498021577508466,2.618981174536));
#18324=CARTESIAN_POINT('Ctrl Pts',(4.06566601882076,0.498217963156433,2.71004109669973));
#18325=CARTESIAN_POINT('Ctrl Pts',(4.07245903442752,0.49843691230792,2.80101058727309));
#18326=CARTESIAN_POINT('Ctrl Pts',(4.0807766690114,0.49868446715054,2.89180185627502));
#18327=CARTESIAN_POINT('Ctrl Pts',(4.06908600086855,0.494206646511993,2.61825188608136));
#18328=CARTESIAN_POINT('Ctrl Pts',(4.07471056556753,0.494770866965848,2.70927438603916));
#18329=CARTESIAN_POINT('Ctrl Pts',(4.08102662411876,0.495395378179633,2.80019313822991));
#18330=CARTESIAN_POINT('Ctrl Pts',(4.08866768906678,0.496116848585951,2.89094234456325));
#18331=CARTESIAN_POINT('',(4.06895185517798,0.494291809244787,2.61828946467431));
#18332=CARTESIAN_POINT('',(4.03928538163603,0.5,2.62055334362004));
#18333=CARTESIAN_POINT('Origin',(4.03928538163603,0.42,2.62055334362004));
#18334=CARTESIAN_POINT('',(4.06419081564702,0.5,2.89360843325953));
#18335=CARTESIAN_POINT('Ctrl Pts',(4.03928538163603,0.5,2.62055334362004));
#18336=CARTESIAN_POINT('Ctrl Pts',(4.04632311223308,0.5,2.71168199850908));
#18337=CARTESIAN_POINT('Ctrl Pts',(4.05429381417606,0.5,2.80274587021811));
#18338=CARTESIAN_POINT('Ctrl Pts',(4.06419081564702,0.5,2.89360843325953));
#18339=CARTESIAN_POINT('',(4.08866768906134,0.496116848587722,2.89094234456384));
#18340=CARTESIAN_POINT('Origin',(4.06419081564702,0.42,2.89360843325953));
#18341=CARTESIAN_POINT('',(4.06920856586713,0.494219105064871,2.62023245236732));
#18342=CARTESIAN_POINT('Ctrl Pts',(4.08866768906678,0.496116848585951,2.89094234456325));
#18343=CARTESIAN_POINT('Ctrl Pts',(4.08108204558666,0.495400611082276,2.80085135200771));
#18344=CARTESIAN_POINT('Ctrl Pts',(4.07480225738019,0.494779931360968,2.71059326414412));
#18345=CARTESIAN_POINT('Ctrl Pts',(4.06920849696627,0.494218933096588,2.62023245770026));
#18346=CARTESIAN_POINT('Ctrl Pts',(4.06894150822957,0.49426616699978,2.61829026217753));
#18347=CARTESIAN_POINT('Ctrl Pts',(4.06903049704884,0.494250393508785,2.61893766197901));
#18348=CARTESIAN_POINT('Ctrl Pts',(4.06911951629768,0.494234706228949,2.61958505872445));
#18349=CARTESIAN_POINT('Ctrl Pts',(4.06920856586577,0.494219105065422,2.62023245236742));
#18350=CARTESIAN_POINT('Ctrl Pts',(4.06419081564702,0.5,2.89360843325953));
#18351=CARTESIAN_POINT('Ctrl Pts',(4.07131106760875,0.5,2.95897816616719));
#18352=CARTESIAN_POINT('Ctrl Pts',(4.07943237959568,0.5,3.02424484221767));
#18353=CARTESIAN_POINT('Ctrl Pts',(4.08915845468123,0.5,3.0892779371144));
#18354=CARTESIAN_POINT('Ctrl Pts',(4.07248440131376,0.5,2.89270507298886));
#18355=CARTESIAN_POINT('Ctrl Pts',(4.07903627312829,0.499999393689843,2.95804917989885));
#18356=CARTESIAN_POINT('Ctrl Pts',(4.08648871622279,0.500000399314335,3.02329507294375));
#18357=CARTESIAN_POINT('Ctrl Pts',(4.09533030979853,0.5,3.08835490052229));
#18358=CARTESIAN_POINT('Ctrl Pts',(4.0807766690114,0.49868446715054,2.89180185627502));
#18359=CARTESIAN_POINT('Ctrl Pts',(4.08676066872451,0.498862566836487,2.95712029773586));
#18360=CARTESIAN_POINT('Ctrl Pts',(4.09354449716726,0.499059402802659,3.02234538076767));
#18361=CARTESIAN_POINT('Ctrl Pts',(4.10150185721175,0.499266489702861,3.0874319099491));
#18362=CARTESIAN_POINT('Ctrl Pts',(4.08866768906678,0.496116848585951,2.89094234456325));
#18363=CARTESIAN_POINT('Ctrl Pts',(4.09416494071875,0.496635899845162,2.9562305246566));
#18364=CARTESIAN_POINT('Ctrl Pts',(4.1003612228726,0.49720813915017,3.02142856695316));
#18365=CARTESIAN_POINT('Ctrl Pts',(4.10750548227104,0.497819390704154,3.08653403313415));
#18366=CARTESIAN_POINT('',(4.08915845468123,0.5,3.0892779371144));
#18367=CARTESIAN_POINT('',(4.10750548294116,0.497819393547925,3.08653403303397));
#18368=CARTESIAN_POINT('Origin',(4.08915845468123,0.42,3.0892779371144));
#18369=CARTESIAN_POINT('Ctrl Pts',(4.10750548227104,0.497819390704154,3.08653403313415));
#18370=CARTESIAN_POINT('Ctrl Pts',(4.1003612228726,0.49720813915017,3.02142856695316));
#18371=CARTESIAN_POINT('Ctrl Pts',(4.09416494071875,0.496635899845162,2.9562305246566));
#18372=CARTESIAN_POINT('Ctrl Pts',(4.08866768906678,0.496116848585951,2.89094234456325));
#18373=CARTESIAN_POINT('Ctrl Pts',(4.06419081564702,0.5,2.89360843325953));
#18374=CARTESIAN_POINT('Ctrl Pts',(4.07131106760875,0.5,2.95897816616719));
#18375=CARTESIAN_POINT('Ctrl Pts',(4.07943237959568,0.5,3.02424484221767));
#18376=CARTESIAN_POINT('Ctrl Pts',(4.08915845468123,0.5,3.0892779371144));
#18377=CARTESIAN_POINT('Ctrl Pts',(4.07450283659624,0.492655764110889,2.63858224625082));
#18378=CARTESIAN_POINT('Ctrl Pts',(4.05896272385424,0.496331141448606,2.56408596426312));
#18379=CARTESIAN_POINT('Ctrl Pts',(4.04957454955023,0.500000000000001,2.48480145080403));
#18380=CARTESIAN_POINT('Ctrl Pts',(4.04448131648779,0.500000000000001,2.40449423379407));
#18381=CARTESIAN_POINT('Ctrl Pts',(4.06410669092888,0.497480565443957,2.63967404822527));
#18382=CARTESIAN_POINT('Ctrl Pts',(4.05053789212333,0.498773941797688,2.56386105153688));
#18383=CARTESIAN_POINT('Ctrl Pts',(4.04494307880602,0.500000000000001,2.48428386223388));
#18384=CARTESIAN_POINT('Ctrl Pts',(4.04448131648779,0.500000000000001,2.40449423379407));
#18385=CARTESIAN_POINT('Ctrl Pts',(4.05265695048639,0.500002014863448,2.64087431669902));
#18386=CARTESIAN_POINT('Ctrl Pts',(4.04188900161745,0.499993283788508,2.56356311273528));
#18387=CARTESIAN_POINT('Ctrl Pts',(4.04031160806179,0.500000000000001,2.48376627366372));
#18388=CARTESIAN_POINT('Ctrl Pts',(4.04448131648779,0.500000000000001,2.40449423379407));
#18389=CARTESIAN_POINT('Ctrl Pts',(4.0412012036484,0.5,2.64207519476898));
#18390=CARTESIAN_POINT('Ctrl Pts',(4.03324251291048,0.5,2.56326450267563));
#18391=CARTESIAN_POINT('Ctrl Pts',(4.03568013731757,0.500000000000001,2.48324868509357));
#18392=CARTESIAN_POINT('Ctrl Pts',(4.04448131648779,0.500000000000001,2.40449423379407));
#18393=CARTESIAN_POINT('',(4.04442943268642,0.499941163643867,2.40450168102723));
#18394=CARTESIAN_POINT('Ctrl Pts',(4.06886801794898,0.49433551594449,2.61829782579792));
#18395=CARTESIAN_POINT('Ctrl Pts',(4.06465789083201,0.495298098708667,2.59562064419044));
#18396=CARTESIAN_POINT('Ctrl Pts',(4.0608935194358,0.496315176554883,2.57122223594089));
#18397=CARTESIAN_POINT('Ctrl Pts',(4.05758292507581,0.497209522471247,2.54587396190639));
#18398=CARTESIAN_POINT('Ctrl Pts',(4.05456867152398,0.498023812916352,2.52279468467315));
#18399=CARTESIAN_POINT('Ctrl Pts',(4.05193046449298,0.498735979011545,2.49892750607437));
#18400=CARTESIAN_POINT('Ctrl Pts',(4.0497085040971,0.499233961791349,2.47484691613384));
#18401=CARTESIAN_POINT('Ctrl Pts',(4.04754737437031,0.499718311283297,2.45142558114697));
#18402=CARTESIAN_POINT('Ctrl Pts',(4.04577933129341,0.499999944019269,2.42780226396996));
#18403=CARTESIAN_POINT('Ctrl Pts',(4.044481720465,0.499999999991593,2.40450148814583));
#18404=CARTESIAN_POINT('Ctrl Pts',(4.04447960468408,0.500000000000001,2.40450955203947));
#18405=CARTESIAN_POINT('Ctrl Pts',(4.0364798534531,0.500000000000001,2.47609955036283));
#18406=CARTESIAN_POINT('Ctrl Pts',(4.03373870432118,0.5,2.5487317193285));
#18407=CARTESIAN_POINT('Ctrl Pts',(4.03928538163603,0.5,2.62055334362004));
#18408=CARTESIAN_POINT('Ctrl Pts',(4.1,0.5,3.15505167992283));
#18409=CARTESIAN_POINT('Ctrl Pts',(4.12354928830202,0.5,3.3096462519264));
#18410=CARTESIAN_POINT('Ctrl Pts',(4.15597088871579,0.501106120178651,3.46379338521867));
#18411=CARTESIAN_POINT('Ctrl Pts',(4.20302510049204,0.513494829718804,3.61060092780471));
#18412=CARTESIAN_POINT('Ctrl Pts',(4.20327611767679,0.513562280164884,3.61138321913356));
#18413=CARTESIAN_POINT('Ctrl Pts',(4.20352761804101,0.513629669484372,3.61216526483892));
#18414=CARTESIAN_POINT('Ctrl Pts',(4.10514574956508,0.5,3.15411106159347));
#18415=CARTESIAN_POINT('Ctrl Pts',(4.12748779335588,0.500302630511343,3.3086923919502));
#18416=CARTESIAN_POINT('Ctrl Pts',(4.15822497958996,0.501690302643301,3.46288253392766));
#18417=CARTESIAN_POINT('Ctrl Pts',(4.20304883308115,0.513501203389107,3.61059108834772));
#18418=CARTESIAN_POINT('Ctrl Pts',(4.20328800103192,0.513565464300295,3.61137830395557));
#18419=CARTESIAN_POINT('Ctrl Pts',(4.20352761804101,0.513629669484372,3.61216526483892));
#18420=CARTESIAN_POINT('Ctrl Pts',(4.11029137237376,0.499485295444531,3.15317046643458));
#18421=CARTESIAN_POINT('Ctrl Pts',(4.13145665971031,0.500324828934127,3.30773853156512));
#18422=CARTESIAN_POINT('Ctrl Pts',(4.1604840495311,0.502266600047225,3.46197168157039));
#18423=CARTESIAN_POINT('Ctrl Pts',(4.20307255308428,0.513507583754598,3.61058124889467));
#18424=CARTESIAN_POINT('Ctrl Pts',(4.20329988438705,0.513568648435705,3.61137338877759));
#18425=CARTESIAN_POINT('Ctrl Pts',(4.20352761804101,0.513629669484372,3.61216526483892));
#18426=CARTESIAN_POINT('Ctrl Pts',(4.11533843497839,0.498465732400005,3.15224788760805));
#18427=CARTESIAN_POINT('Ctrl Pts',(4.13542434682827,0.500061728589708,3.30679480627255));
#18428=CARTESIAN_POINT('Ctrl Pts',(4.16275021805235,0.502834940834963,3.46106041128606));
#18429=CARTESIAN_POINT('Ctrl Pts',(4.20309625252131,0.513513971085243,3.61057141101541));
#18430=CARTESIAN_POINT('Ctrl Pts',(4.20331176774218,0.513571832571116,3.6113684735996));
#18431=CARTESIAN_POINT('Ctrl Pts',(4.20352761804101,0.513629669484372,3.61216526483892));
#18432=CARTESIAN_POINT('',(4.1,0.5,3.15505167992283));
#18433=CARTESIAN_POINT('Ctrl Pts',(4.1,0.5,3.15505167992283));
#18434=CARTESIAN_POINT('Ctrl Pts',(4.12354928830202,0.5,3.3096462519264));
#18435=CARTESIAN_POINT('Ctrl Pts',(4.15597088871579,0.501106120178651,3.46379338521867));
#18436=CARTESIAN_POINT('Ctrl Pts',(4.20302510049204,0.513494829718804,3.61060092780471));
#18437=CARTESIAN_POINT('Ctrl Pts',(4.20327611767679,0.513562280164884,3.61138321913356));
#18438=CARTESIAN_POINT('Ctrl Pts',(4.20352761804101,0.513629669484372,3.61216526483892));
#18439=CARTESIAN_POINT('',(4.20223747325117,0.513287047238827,3.60738446017534));
#18440=CARTESIAN_POINT('Ctrl Pts',(4.20352761804101,0.513629669484372,3.61216526483892));
#18441=CARTESIAN_POINT('Ctrl Pts',(4.20331176774218,0.513571832571116,3.6113684735996));
#18442=CARTESIAN_POINT('Ctrl Pts',(4.20309625252131,0.513513971085243,3.61057141101541));
#18443=CARTESIAN_POINT('Ctrl Pts',(4.20266625878817,0.513400157766436,3.60897797578032));
#18444=CARTESIAN_POINT('Ctrl Pts',(4.20245168277568,0.513343490433672,3.60818129720179));
#18445=CARTESIAN_POINT('Ctrl Pts',(4.20223747325117,0.513287047238827,3.60738446017534));
#18446=CARTESIAN_POINT('',(4.11533843497839,0.498465732400005,3.15224788760805));
#18447=CARTESIAN_POINT('Ctrl Pts',(4.20223747325117,0.513287047238827,3.60738446017534));
#18448=CARTESIAN_POINT('Ctrl Pts',(4.16245770855631,0.502805267707013,3.45940789617989));
#18449=CARTESIAN_POINT('Ctrl Pts',(4.13531676578111,0.500053180362341,3.30596704602595));
#18450=CARTESIAN_POINT('Ctrl Pts',(4.11533843497839,0.498465732400005,3.15224788760805));
#18451=CARTESIAN_POINT('Origin',(4.1,0.42,3.15505167992283));
#18452=CARTESIAN_POINT('Ctrl Pts',(4.08915845468123,0.5,3.0892779371144));
#18453=CARTESIAN_POINT('Ctrl Pts',(4.09244523897257,0.5,3.11125491681526));
#18454=CARTESIAN_POINT('Ctrl Pts',(4.09600424357276,0.5,3.13319248235467));
#18455=CARTESIAN_POINT('Ctrl Pts',(4.1,0.5,3.15505167992283));
#18456=CARTESIAN_POINT('Ctrl Pts',(4.09533030979853,0.5,3.08835490052229));
#18457=CARTESIAN_POINT('Ctrl Pts',(4.09831694095011,0.499999865724806,3.11032259202407));
#18458=CARTESIAN_POINT('Ctrl Pts',(4.10154259105465,0.500000103565783,3.13225323052938));
#18459=CARTESIAN_POINT('Ctrl Pts',(4.10514574956508,0.5,3.15411106159347));
#18460=CARTESIAN_POINT('Ctrl Pts',(4.10150185721175,0.499266489702861,3.0874319099491));
#18461=CARTESIAN_POINT('Ctrl Pts',(4.10418841876551,0.499336125654538,3.10939030384142));
#18462=CARTESIAN_POINT('Ctrl Pts',(4.10708075806979,0.4994092082085,3.13131400963607));
#18463=CARTESIAN_POINT('Ctrl Pts',(4.11029137237376,0.499485295444531,3.15317046643458));
#18464=CARTESIAN_POINT('Ctrl Pts',(4.10750548227104,0.497819390704154,3.08653403313415));
#18465=CARTESIAN_POINT('Ctrl Pts',(4.10991596810902,0.49802493283953,3.10848101609958));
#18466=CARTESIAN_POINT('Ctrl Pts',(4.11249834874657,0.498240063441667,3.13039542807567));
#18467=CARTESIAN_POINT('Ctrl Pts',(4.1153384349784,0.498465732400005,3.15224788760805));
#18468=CARTESIAN_POINT('Ctrl Pts',(4.11533084388102,0.498427288961305,3.15224922644314));
#18469=CARTESIAN_POINT('Ctrl Pts',(4.11249458022437,0.498223938268274,3.13039599596135));
#18470=CARTESIAN_POINT('Ctrl Pts',(4.10991588274464,0.498024571772185,3.10848102746594));
#18471=CARTESIAN_POINT('Ctrl Pts',(4.10750548495196,0.497819402079132,3.08653403273337));
#18472=CARTESIAN_POINT('Ctrl Pts',(4.08915845468123,0.5,3.0892779371144));
#18473=CARTESIAN_POINT('Ctrl Pts',(4.09244523897257,0.5,3.11125491681526));
#18474=CARTESIAN_POINT('Ctrl Pts',(4.09600424357276,0.5,3.13319248235467));
#18475=CARTESIAN_POINT('Ctrl Pts',(4.1,0.5,3.15505167992283));
#18476=CARTESIAN_POINT('Ctrl Pts',(4.08866768906678,0.496116848585951,2.89094234456324));
#18477=CARTESIAN_POINT('Ctrl Pts',(4.08065486646877,0.49551208126272,2.80011197287451));
#18478=CARTESIAN_POINT('Ctrl Pts',(4.07407036444164,0.495008985691453,2.70919313424665));
#18479=CARTESIAN_POINT('Ctrl Pts',(4.06822070400199,0.494561147702366,2.61828756807606));
#18480=CARTESIAN_POINT('Ctrl Pts',(4.10320659093045,0.491413943800592,2.89015338698478));
#18481=CARTESIAN_POINT('Ctrl Pts',(4.09590560906221,0.490023602254911,2.79936307019029));
#18482=CARTESIAN_POINT('Ctrl Pts',(4.08980775472146,0.488878406811895,2.7084928654444));
#18483=CARTESIAN_POINT('Ctrl Pts',(4.08435563880312,0.487840362968629,2.61762358805541));
#18484=CARTESIAN_POINT('Ctrl Pts',(4.11909837273532,0.491006921387143,2.88921565674865));
#18485=CARTESIAN_POINT('Ctrl Pts',(4.11282012019298,0.489318592483934,2.79845239738339));
#18486=CARTESIAN_POINT('Ctrl Pts',(4.10749604313151,0.487903857194521,2.7076259216545));
#18487=CARTESIAN_POINT('Ctrl Pts',(4.10271622937717,0.486617339304039,2.61678827445837));
#18488=CARTESIAN_POINT('Ctrl Pts',(4.13385008609474,0.494959631068776,2.88827625586696));
#18489=CARTESIAN_POINT('Ctrl Pts',(4.12845897149287,0.493515086264903,2.79753965428624));
#18490=CARTESIAN_POINT('Ctrl Pts',(4.12379844489011,0.492266301925388,2.70675672533888));
#18491=CARTESIAN_POINT('Ctrl Pts',(4.11959214370927,0.491139226920861,2.61595042854269));
#18492=CARTESIAN_POINT('',(4.1102894955425,0.490554628217515,2.74850282871571));
#18493=CARTESIAN_POINT('Ctrl Pts',(4.10983817729973,0.490298889823543,2.74868144584745));
#18494=CARTESIAN_POINT('Ctrl Pts',(4.09912059002179,0.489547803684328,2.73380263969482));
#18495=CARTESIAN_POINT('Ctrl Pts',(4.09060288993725,0.490523597563226,2.70804325577999));
#18496=CARTESIAN_POINT('Ctrl Pts',(4.07916964200075,0.492005281603662,2.66917053317873));
#18497=CARTESIAN_POINT('Ctrl Pts',(4.07363486591143,0.493180967854886,2.64394223670214));
#18498=CARTESIAN_POINT('Ctrl Pts',(4.06920856586713,0.494219105064871,2.62023245236732));
#18499=CARTESIAN_POINT('Origin',(4.11314456248654,0.572233697171902,2.88827625586697));
#18500=CARTESIAN_POINT('Ctrl Pts',(4.12725971987735,0.493193747719603,2.77093882623153));
#18501=CARTESIAN_POINT('Ctrl Pts',(4.12455800459528,0.492469895869088,2.76708747448196));
#18502=CARTESIAN_POINT('Ctrl Pts',(4.1218042657884,0.491865483418447,2.76326519725518));
#18503=CARTESIAN_POINT('Ctrl Pts',(4.11625238064331,0.490914087391762,2.75567430292574));
#18504=CARTESIAN_POINT('Ctrl Pts',(4.11346892427127,0.490565796408723,2.75192428752783));
#18505=CARTESIAN_POINT('Ctrl Pts',(4.11066809033619,0.490343257580657,2.74816669957651));
#18506=CARTESIAN_POINT('Ctrl Pts',(4.10750548227104,0.497819390704154,3.08653403313415));
#18507=CARTESIAN_POINT('Ctrl Pts',(4.09988751844767,0.497321971238036,3.02148952956988));
#18508=CARTESIAN_POINT('Ctrl Pts',(4.09333086416513,0.496883068938475,2.95626908269239));
#18509=CARTESIAN_POINT('Ctrl Pts',(4.08753393606525,0.496492976538145,2.89100371845852));
#18510=CARTESIAN_POINT('Ctrl Pts',(4.12030577414111,0.494771961793561,3.08569517253432));
#18511=CARTESIAN_POINT('Ctrl Pts',(4.11358761799295,0.493524694122167,3.02063134445983));
#18512=CARTESIAN_POINT('Ctrl Pts',(4.1076623367844,0.492431642898789,2.9554374626284));
#18513=CARTESIAN_POINT('Ctrl Pts',(4.10237819873081,0.491444738231125,2.89020211564854));
#18514=CARTESIAN_POINT('Ctrl Pts',(4.13385584109311,0.494961173115941,3.08474311994105));
#18515=CARTESIAN_POINT('Ctrl Pts',(4.12828398728823,0.493463687530671,3.01963734956761));
#18516=CARTESIAN_POINT('Ctrl Pts',(4.12324167296667,0.492121940958461,2.95445550879435));
#18517=CARTESIAN_POINT('Ctrl Pts',(4.11871398375975,0.490903924671562,2.88924013494544));
#18518=CARTESIAN_POINT('Ctrl Pts',(4.14655803346906,0.498364715305182,3.0837901291539));
#18519=CARTESIAN_POINT('Ctrl Pts',(4.14199767141828,0.497142769976483,3.01864202972875));
#18520=CARTESIAN_POINT('Ctrl Pts',(4.13772368979234,0.495997560051348,2.95347198278946));
#18521=CARTESIAN_POINT('Ctrl Pts',(4.13385008609474,0.494959631068777,2.88827625586697));
#18522=CARTESIAN_POINT('Origin',(4.12585250986086,0.575638781408308,3.0837901291539));
#18523=CARTESIAN_POINT('Ctrl Pts',(4.20352761804101,0.513629669484372,3.61216526483892));
#18524=CARTESIAN_POINT('Ctrl Pts',(4.2034515520887,0.51360928767388,3.61188709994706));
#18525=CARTESIAN_POINT('Ctrl Pts',(4.20337579441033,0.513588620909437,3.61160915407523));
#18526=CARTESIAN_POINT('Ctrl Pts',(4.15654326855526,0.501204320694855,3.43986804670352));
#18527=CARTESIAN_POINT('Ctrl Pts',(4.12742700794855,0.499257234215814,3.26327059408423));
#18528=CARTESIAN_POINT('Ctrl Pts',(4.10655417222842,0.498052118158934,3.0865962596308));
#18529=CARTESIAN_POINT('Ctrl Pts',(4.20352761804101,0.513629669484372,3.61216526483892));
#18530=CARTESIAN_POINT('Ctrl Pts',(4.20346328242755,0.5136124308087,3.61188634858972));
#18531=CARTESIAN_POINT('Ctrl Pts',(4.20339351891518,0.513598371022242,3.61160471600277));
#18532=CARTESIAN_POINT('Ctrl Pts',(4.16301739273852,0.502680404850424,3.4388303755424));
#18533=CARTESIAN_POINT('Ctrl Pts',(4.13810208850384,0.497947580543976,3.26236737839722));
#18534=CARTESIAN_POINT('Ctrl Pts',(4.11963294253909,0.494765631312812,3.08574238943294));
#18535=CARTESIAN_POINT('Ctrl Pts',(4.20352761804101,0.513629669484372,3.61216526483892));
#18536=CARTESIAN_POINT('Ctrl Pts',(4.20347237327524,0.513614866693999,3.61188267429505));
#18537=CARTESIAN_POINT('Ctrl Pts',(4.20341613842376,0.513599798610958,3.61160296503507));
#18538=CARTESIAN_POINT('Ctrl Pts',(4.16924973697742,0.504444938935139,3.43771198364712));
#18539=CARTESIAN_POINT('Ctrl Pts',(4.14873646433035,0.498948424095233,3.26128633907584));
#18540=CARTESIAN_POINT('Ctrl Pts',(4.13354070272714,0.494876732045277,3.08476676341538));
#18541=CARTESIAN_POINT('Ctrl Pts',(4.20352761804101,0.513629669484372,3.61216526483892));
#18542=CARTESIAN_POINT('Ctrl Pts',(4.20348225943688,0.513617515683026,3.61188189200445));
#18543=CARTESIAN_POINT('Ctrl Pts',(4.20343686017451,0.513605350987338,3.61159855052174));
#18544=CARTESIAN_POINT('Ctrl Pts',(4.17554861335302,0.506132717773207,3.43668170480236));
#18545=CARTESIAN_POINT('Ctrl Pts',(4.15891388414094,0.501675455514513,3.26030247161513));
#18546=CARTESIAN_POINT('Ctrl Pts',(4.14655803346906,0.498364715305183,3.0837901291539));
#18547=CARTESIAN_POINT('Ctrl Pts',(4.06730463307991,0.5,2.7548988716696));
#18548=CARTESIAN_POINT('Ctrl Pts',(4.04477623135907,0.5,2.46323477342689));
#18549=CARTESIAN_POINT('Ctrl Pts',(4.03124587888692,0.500000000000004,2.17098509479316));
#18550=CARTESIAN_POINT('Ctrl Pts',(4.02013482858588,0.5,1.87705481005079));
#18551=CARTESIAN_POINT('Ctrl Pts',(4.02006773773253,0.5,1.87522368040185));
#18552=CARTESIAN_POINT('Ctrl Pts',(4.02,0.5,1.87339241925346));
#18553=CARTESIAN_POINT('Ctrl Pts',(4.0701214409961,0.488945949397786,2.75298513275217));
#18554=CARTESIAN_POINT('Ctrl Pts',(4.0521727324952,0.495960044053856,2.46215351379707));
#18555=CARTESIAN_POINT('Ctrl Pts',(4.03379752250834,0.500113514316493,2.17064344747657));
#18556=CARTESIAN_POINT('Ctrl Pts',(4.02016777946955,0.49999925948703,1.8770506998427));
#18557=CARTESIAN_POINT('Ctrl Pts',(4.02008397514388,0.5,1.87522162637816));
#18558=CARTESIAN_POINT('Ctrl Pts',(4.02,0.5,1.87339241925346));
#18559=CARTESIAN_POINT('Ctrl Pts',(4.07538773587724,0.478557974340581,2.7508822733927));
#18560=CARTESIAN_POINT('Ctrl Pts',(4.05924753225934,0.493164525555191,2.46115599049795));
#18561=CARTESIAN_POINT('Ctrl Pts',(4.03637623393824,0.500137583027881,2.17029238050623));
#18562=CARTESIAN_POINT('Ctrl Pts',(4.02020061161559,0.499998948815406,1.87704663109656));
#18563=CARTESIAN_POINT('Ctrl Pts',(4.02010021255523,0.5,1.87521957235447));
#18564=CARTESIAN_POINT('Ctrl Pts',(4.02,0.5,1.87339241925346));
#18565=CARTESIAN_POINT('Ctrl Pts',(4.08262506058196,0.469786517311005,2.74878220268511));
#18566=CARTESIAN_POINT('Ctrl Pts',(4.0658320892877,0.491020613169402,2.46015855202445));
#18567=CARTESIAN_POINT('Ctrl Pts',(4.03900592459406,0.500139057369812,2.16994131329339));
#18568=CARTESIAN_POINT('Ctrl Pts',(4.02023321948065,0.49999877382774,1.8770425623582));
#18569=CARTESIAN_POINT('Ctrl Pts',(4.02011644996657,0.5,1.87521751833078));
#18570=CARTESIAN_POINT('Ctrl Pts',(4.02,0.5,1.87339241925346));
#18571=CARTESIAN_POINT('',(4.07425885705739,0.479232380498994,2.68379303474969));
#18572=CARTESIAN_POINT('Ctrl Pts',(4.04448172046659,0.499999999988976,2.40450148817435));
#18573=CARTESIAN_POINT('Ctrl Pts',(4.04463591392868,0.499999991267764,2.40727029004885));
#18574=CARTESIAN_POINT('Ctrl Pts',(4.04479651104661,0.499994808468355,2.4100383627539));
#18575=CARTESIAN_POINT('Ctrl Pts',(4.04496328520179,0.499984248258457,2.41280641893295));
#18576=CARTESIAN_POINT('Ctrl Pts',(4.04516949057082,0.499971191247455,2.41622893991844));
#18577=CARTESIAN_POINT('Ctrl Pts',(4.04538506477277,0.499949917237401,2.41965021876981));
#18578=CARTESIAN_POINT('Ctrl Pts',(4.04560958710345,0.499920089612813,2.42307148910707));
#18579=CARTESIAN_POINT('Ctrl Pts',(4.046168184163,0.49984588040904,2.43158338876807));
#18580=CARTESIAN_POINT('Ctrl Pts',(4.04678126083676,0.499718763421518,2.44008296252431));
#18581=CARTESIAN_POINT('Ctrl Pts',(4.04744268468172,0.499534811332572,2.44858609368312));
#18582=CARTESIAN_POINT('Ctrl Pts',(4.04916608154842,0.4990555083015,2.47074173519485));
#18583=CARTESIAN_POINT('Ctrl Pts',(4.0512029869943,0.49818690046067,2.49278507911436));
#18584=CARTESIAN_POINT('Ctrl Pts',(4.05345548579231,0.496916182347658,2.51477945136454));
#18585=CARTESIAN_POINT('Ctrl Pts',(4.05591683934511,0.495527641521432,2.53881317174981));
#18586=CARTESIAN_POINT('Ctrl Pts',(4.05863587671313,0.493660110871332,2.56278860465434));
#18587=CARTESIAN_POINT('Ctrl Pts',(4.06154550645518,0.49131004765369,2.58679034176726));
#18588=CARTESIAN_POINT('Ctrl Pts',(4.06260468059428,0.490454568982503,2.59552754254441));
#18589=CARTESIAN_POINT('Ctrl Pts',(4.06368963170895,0.489535178864469,2.60426823220296));
#18590=CARTESIAN_POINT('Ctrl Pts',(4.06479877481585,0.488551656167653,2.61301647477758));
#18591=CARTESIAN_POINT('Ctrl Pts',(4.06741316103876,0.486233372645465,2.63363715457938));
#18592=CARTESIAN_POINT('Ctrl Pts',(4.07015511481845,0.483565049488091,2.65424997138026));
#18593=CARTESIAN_POINT('Ctrl Pts',(4.07300374745784,0.480567084366157,2.67479487671516));
#18594=CARTESIAN_POINT('Ctrl Pts',(4.0734198337187,0.480129185817727,2.67779577360951));
#18595=CARTESIAN_POINT('Ctrl Pts',(4.07383822268607,0.479684259277039,2.68079522108865));
#18596=CARTESIAN_POINT('Ctrl Pts',(4.07425885705739,0.479232380498994,2.68379303474969));
#18597=CARTESIAN_POINT('',(4.0809602708998,0.471805843027818,2.72818635208988));
#18598=CARTESIAN_POINT('Ctrl Pts',(4.07431256837795,0.479317097635081,2.68379826229727));
#18599=CARTESIAN_POINT('Ctrl Pts',(4.07535643858548,0.478197393643414,2.69122711204079));
#18600=CARTESIAN_POINT('Ctrl Pts',(4.0764134383116,0.477033123389242,2.69864815707777));
#18601=CARTESIAN_POINT('Ctrl Pts',(4.07855234656971,0.474619335589603,2.71346580990626));
#18602=CARTESIAN_POINT('Ctrl Pts',(4.07963448015113,0.473369601956344,2.7208641126329));
#18603=CARTESIAN_POINT('Ctrl Pts',(4.08072980562297,0.472078321008102,2.72825206195681));
#18604=CARTESIAN_POINT('',(4.02,0.5,1.87339241925342));
#18605=CARTESIAN_POINT('Ctrl Pts',(4.0809602708998,0.471805843027818,2.72818635208988));
#18606=CARTESIAN_POINT('Ctrl Pts',(4.07764839286774,0.475702951350386,2.67263460081295));
#18607=CARTESIAN_POINT('Ctrl Pts',(4.07398527921688,0.479249586578106,2.61702556232049));
#18608=CARTESIAN_POINT('Ctrl Pts',(4.07009274281801,0.482375613159057,2.56136441565828));
#18609=CARTESIAN_POINT('Ctrl Pts',(4.06612731105444,0.485560180707732,2.50466090505392));
#18610=CARTESIAN_POINT('Ctrl Pts',(4.06192505627188,0.488307767931295,2.44790331635054));
#18611=CARTESIAN_POINT('Ctrl Pts',(4.05763254837964,0.490595972282094,2.39109712504011));
#18612=CARTESIAN_POINT('Ctrl Pts',(4.05327949071071,0.492916453862411,2.33348963008985));
#18613=CARTESIAN_POINT('Ctrl Pts',(4.04883495697235,0.49476468329804,2.27583215169267));
#18614=CARTESIAN_POINT('Ctrl Pts',(4.0444496090073,0.496172282487727,2.21813040033497));
#18615=CARTESIAN_POINT('Ctrl Pts',(4.03986024699307,0.497645365651001,2.15774426269066));
#18616=CARTESIAN_POINT('Ctrl Pts',(4.03533701131399,0.498636468850484,2.0973096369561));
#18617=CARTESIAN_POINT('Ctrl Pts',(4.03102904348286,0.499236104143585,2.03683306825523));
#18618=CARTESIAN_POINT('Ctrl Pts',(4.02728039024729,0.49975788723709,1.98420832874381));
#18619=CARTESIAN_POINT('Ctrl Pts',(4.02369449212959,0.499984720705903,1.93155183038186));
#18620=CARTESIAN_POINT('Ctrl Pts',(4.02034716371852,0.499999246729907,1.87886788564175));
#18621=CARTESIAN_POINT('Ctrl Pts',(4.02023120593227,0.499999749938848,1.87704281416613));
#18622=CARTESIAN_POINT('Ctrl Pts',(4.02011544505978,0.5,1.87521764545094));
#18623=CARTESIAN_POINT('Ctrl Pts',(4.02,0.5,1.87339241925346));
#18624=CARTESIAN_POINT('Ctrl Pts',(4.02,0.5,1.87339241925346));
#18625=CARTESIAN_POINT('Ctrl Pts',(4.02002404870585,0.5,1.87404256591536));
#18626=CARTESIAN_POINT('Ctrl Pts',(4.020048124588,0.499999999225747,1.87469286273721));
#18627=CARTESIAN_POINT('Ctrl Pts',(4.02007222763371,0.49999999809316,1.87534330899108));
#18628=CARTESIAN_POINT('Ctrl Pts',(4.02009633067943,0.499999996960572,1.87599375524495));
#18629=CARTESIAN_POINT('Ctrl Pts',(4.0201204602048,0.499999996385127,1.87664435102068));
#18630=CARTESIAN_POINT('Ctrl Pts',(4.02014462258731,0.4999999976786,1.87729509477937));
#18631=CARTESIAN_POINT('Ctrl Pts',(4.0201643119008,0.499999998732619,1.8778253693857));
#18632=CARTESIAN_POINT('Ctrl Pts',(4.02018411754459,0.499999999632519,1.87835571847931));
#18633=CARTESIAN_POINT('Ctrl Pts',(4.02020412741357,0.499999999958576,1.87888616583914));
#18634=CARTESIAN_POINT('Ctrl Pts',(4.0202332290698,0.50000000043278,1.87965762999687));
#18635=CARTESIAN_POINT('Ctrl Pts',(4.02026240571076,0.5,1.88042926065977));
#18636=CARTESIAN_POINT('Ctrl Pts',(4.02029161790995,0.5,1.88120111622291));
#18637=CARTESIAN_POINT('Ctrl Pts',(4.02039021406171,0.5,1.88380626031799));
#18638=CARTESIAN_POINT('Ctrl Pts',(4.02048909882791,0.5,1.88641377586908));
#18639=CARTESIAN_POINT('Ctrl Pts',(4.02058827628576,0.5,1.88902361917288));
#18640=CARTESIAN_POINT('Ctrl Pts',(4.02078663120146,0.5,1.89424330578047));
#18641=CARTESIAN_POINT('Ctrl Pts',(4.02098611903685,0.500000001963655,1.89947230693178));
#18642=CARTESIAN_POINT('Ctrl Pts',(4.02118710576848,0.499999999141363,1.90471020328437));
#18643=CARTESIAN_POINT('Ctrl Pts',(4.02348494037357,0.499999966874759,1.96459385530179));
#18644=CARTESIAN_POINT('Ctrl Pts',(4.02595913585852,0.499998572838881,2.02564279695681));
#18645=CARTESIAN_POINT('Ctrl Pts',(4.02865623488046,0.499980627301766,2.08729249963769));
#18646=CARTESIAN_POINT('Ctrl Pts',(4.03110154710007,0.499964357064434,2.143186914368));
#18647=CARTESIAN_POINT('Ctrl Pts',(4.03372928221755,0.499932544589326,2.19957498349665));
#18648=CARTESIAN_POINT('Ctrl Pts',(4.03653956308091,0.499898182578179,2.25604062027684));
#18649=CARTESIAN_POINT('Ctrl Pts',(4.03900413643723,0.499868047619696,2.30556012054119));
#18650=CARTESIAN_POINT('Ctrl Pts',(4.04160722520186,0.499835636299494,2.35513929660828));
#18651=CARTESIAN_POINT('Ctrl Pts',(4.04434137221638,0.499842074417939,2.40450200575315));
#18652=CARTESIAN_POINT('Ctrl Pts',(4.22955939312853,0.10102905344224,11.7707450664009));
#18653=CARTESIAN_POINT('Ctrl Pts',(4.21654931683645,0.207401903813072,11.7841012806179));
#18654=CARTESIAN_POINT('Ctrl Pts',(4.20605403928643,0.31441823415144,11.7948904430433));
#18655=CARTESIAN_POINT('Ctrl Pts',(4.19893756066089,0.421920994121332,11.8021991336745));
#18656=CARTESIAN_POINT('Ctrl Pts',(4.24536267111276,0.104989885152963,11.7545212387652));
#18657=CARTESIAN_POINT('Ctrl Pts',(4.23114949583097,0.210504261951862,11.7691939848541));
#18658=CARTESIAN_POINT('Ctrl Pts',(4.21935602279,0.316778326210449,11.7811764288609));
#18659=CARTESIAN_POINT('Ctrl Pts',(4.21085539742978,0.423544704078567,11.7899594459956));
#18660=CARTESIAN_POINT('Ctrl Pts',(4.28598710678366,0.111856705035166,11.7392780563968));
#18661=CARTESIAN_POINT('Ctrl Pts',(4.2674307302526,0.215927568411162,11.7537105073236));
#18662=CARTESIAN_POINT('Ctrl Pts',(4.25155716799185,0.320887527746463,11.7661024302623));
#18663=CARTESIAN_POINT('Ctrl Pts',(4.23883095697931,0.42637816873375,11.77559001791));
#18664=CARTESIAN_POINT('Ctrl Pts',(4.32514653100426,0.114600833742749,11.7555174901866));
#18665=CARTESIAN_POINT('Ctrl Pts',(4.30459583266175,0.218704714738053,11.7646869062335));
#18666=CARTESIAN_POINT('Ctrl Pts',(4.28594490659705,0.323351812836807,11.7725098097745));
#18667=CARTESIAN_POINT('Ctrl Pts',(4.26959555894274,0.428231125093901,11.7783349626985));
#18668=CARTESIAN_POINT('Ctrl Pts',(4.33821035750186,0.1147842101985,11.7667789364918));
#18669=CARTESIAN_POINT('Ctrl Pts',(4.31798914414459,0.219217033838757,11.7734397365619));
#18670=CARTESIAN_POINT('Ctrl Pts',(4.29900887782759,0.323961874179476,11.7788360517208));
#18671=CARTESIAN_POINT('Ctrl Pts',(4.28176747596058,0.428754931584936,11.7824947042679));
#18672=CARTESIAN_POINT('',(4.28177589321514,0.428644841197042,11.7824875832413));
#18673=CARTESIAN_POINT('',(4.19894501008283,0.421808480676737,11.8021914830441));
#18674=CARTESIAN_POINT('Origin',(4.25626225479035,0.421808480673776,11.858001280205));
#18675=CARTESIAN_POINT('',(4.2295457775513,0.101140384725978,11.770759044231));
#18676=CARTESIAN_POINT('Ctrl Pts',(4.19894501008295,0.421808480673776,11.802191483044));
#18677=CARTESIAN_POINT('Ctrl Pts',(4.20605887902608,0.314381068971518,11.7948854653236));
#18678=CARTESIAN_POINT('Ctrl Pts',(4.21654653248185,0.2074394630476,11.7841041492711));
#18679=CARTESIAN_POINT('Ctrl Pts',(4.2295457775513,0.101140384725978,11.770759044231));
#18680=CARTESIAN_POINT('',(4.33817886049863,0.114893365388572,11.7667770031876));
#18681=CARTESIAN_POINT('Origin',(4.28685203791006,0.101140384725978,11.8265801202122));
#18682=CARTESIAN_POINT('Ctrl Pts',(4.33817886049861,0.114893365388635,11.7667770031876));
#18683=CARTESIAN_POINT('Ctrl Pts',(4.3293833989095,0.16031902928837,11.7696747648638));
#18684=CARTESIAN_POINT('Ctrl Pts',(4.32083110204483,0.205805953395781,11.7723064625421));
#18685=CARTESIAN_POINT('Ctrl Pts',(4.31254982212002,0.251328908890292,11.7746750829505));
#18686=CARTESIAN_POINT('Ctrl Pts',(4.30465032591334,0.294753164260322,11.7769345051777));
#18687=CARTESIAN_POINT('Ctrl Pts',(4.29699862304371,0.338210524013558,11.7789549955099));
#18688=CARTESIAN_POINT('Ctrl Pts',(4.2896312933914,0.381682414128188,11.7806948857785));
#18689=CARTESIAN_POINT('Ctrl Pts',(4.28697846310439,0.397335785454289,11.781321385992));
#18690=CARTESIAN_POINT('Ctrl Pts',(4.28436254073142,0.412991050589563,11.7819110385617));
#18691=CARTESIAN_POINT('Ctrl Pts',(4.28178519416781,0.428647331668438,11.7824601840726));
#18692=CARTESIAN_POINT('Ctrl Pts',(4.2486735668154,0.525726490000048,11.7797315270537));
#18693=CARTESIAN_POINT('Ctrl Pts',(4.26374619995914,0.497289984563685,11.7830226438474));
#18694=CARTESIAN_POINT('Ctrl Pts',(4.27616566022512,0.462742784615148,11.783679000487));
#18695=CARTESIAN_POINT('Ctrl Pts',(4.28177589348483,0.428644839557943,11.782487583184));
#18696=CARTESIAN_POINT('Ctrl Pts',(4.2368038791629,0.514253184188583,11.773132618748));
#18697=CARTESIAN_POINT('Ctrl Pts',(4.25038555537826,0.48960012188578,11.777985280354));
#18698=CARTESIAN_POINT('Ctrl Pts',(4.26245207313798,0.458525980311001,11.7793725972104));
#18699=CARTESIAN_POINT('Ctrl Pts',(4.26757735435752,0.428033621458704,11.7776350210923));
#18700=CARTESIAN_POINT('Ctrl Pts',(4.20817000679401,0.490033235054154,11.7711728984776));
#18701=CARTESIAN_POINT('Ctrl Pts',(4.22105394566052,0.473487226884366,11.7768547886379));
#18702=CARTESIAN_POINT('Ctrl Pts',(4.23282911654911,0.449515232679256,11.7785372227129));
#18703=CARTESIAN_POINT('Ctrl Pts',(4.2364394051555,0.426069510514664,11.7761487419229));
#18704=CARTESIAN_POINT('Ctrl Pts',(4.18191946942526,0.473520527526364,11.7923527205827));
#18705=CARTESIAN_POINT('Ctrl Pts',(4.19617224734773,0.460605230875895,11.7941633853966));
#18706=CARTESIAN_POINT('Ctrl Pts',(4.20728837804396,0.442036565491117,11.7934702039683));
#18707=CARTESIAN_POINT('Ctrl Pts',(4.20937438480907,0.423229901258667,11.7914804062487));
#18708=CARTESIAN_POINT('Ctrl Pts',(4.17218826315047,0.468962654353794,11.80651609725));
#18709=CARTESIAN_POINT('Ctrl Pts',(4.18688126868098,0.455889756420883,11.806032917619));
#18710=CARTESIAN_POINT('Ctrl Pts',(4.19736873106825,0.439262007746224,11.8038103380598));
#18711=CARTESIAN_POINT('Ctrl Pts',(4.19894501008283,0.421808480676737,11.8021914830441));
#18712=CARTESIAN_POINT('Ctrl Pts',(4.28177589321514,0.428644841197042,11.7824875832413));
#18713=CARTESIAN_POINT('Ctrl Pts',(4.27616577833755,0.462742065438141,11.7836789752985));
#18714=CARTESIAN_POINT('Ctrl Pts',(4.26374672441132,0.497288525471169,11.7830226715236));
#18715=CARTESIAN_POINT('Ctrl Pts',(4.24867452199362,0.525724687915784,11.7797317356146));
#18716=CARTESIAN_POINT('',(4.17218826315256,0.468962654354822,11.8065160972469));
#18717=CARTESIAN_POINT('Origin',(4.21654544948669,0.517117786907486,11.8524891679444));
#18718=CARTESIAN_POINT('Ctrl Pts',(4.17218826315047,0.468962654353794,11.80651609725));
#18719=CARTESIAN_POINT('Ctrl Pts',(4.18688126868098,0.455889756420883,11.806032917619));
#18720=CARTESIAN_POINT('Ctrl Pts',(4.19736873106825,0.439262007746224,11.8038103380598));
#18721=CARTESIAN_POINT('Ctrl Pts',(4.19894501008283,0.421808480676737,11.8021914830441));
#18722=CARTESIAN_POINT('Ctrl Pts',(4.23244357912718,0.0834503638580652,
11.7677845155721));
#18723=CARTESIAN_POINT('Ctrl Pts',(4.23124359603722,0.0892621551574759,
11.7690161098144));
#18724=CARTESIAN_POINT('Ctrl Pts',(4.23027567575553,0.0951717685553224,
11.7700097262397));
#18725=CARTESIAN_POINT('Ctrl Pts',(4.22954577757009,0.101140384729842,11.7707590442118));
#18726=CARTESIAN_POINT('Ctrl Pts',(4.24783021369305,0.0899565784776398,
11.7519925509196));
#18727=CARTESIAN_POINT('Ctrl Pts',(4.24680279265781,0.0949288632967188,
11.7530451914931));
#18728=CARTESIAN_POINT('Ctrl Pts',(4.24597265680021,0.0999940784592962,
11.7538961092212));
#18729=CARTESIAN_POINT('Ctrl Pts',(4.24534779634232,0.105100317994799,11.7545365944285));
#18730=CARTESIAN_POINT('Ctrl Pts',(4.28772157465326,0.101235139924101,11.7374963477574));
#18731=CARTESIAN_POINT('Ctrl Pts',(4.28699316039155,0.104761359558322,11.7382410744884));
#18732=CARTESIAN_POINT('Ctrl Pts',(4.28640608685963,0.108344058397789,11.7388415688776));
#18733=CARTESIAN_POINT('Ctrl Pts',(4.28596309958905,0.111964864227218,11.7392947835658));
#18734=CARTESIAN_POINT('Ctrl Pts',(4.32658203586776,0.105745113375536,11.7540207776828));
#18735=CARTESIAN_POINT('Ctrl Pts',(4.32597549644476,0.108688259084721,11.7546424103689));
#18736=CARTESIAN_POINT('Ctrl Pts',(4.32548517203557,0.111686864219622,11.7551450805111));
#18737=CARTESIAN_POINT('Ctrl Pts',(4.32511617292258,0.114709169987786,11.7555234177697));
#18738=CARTESIAN_POINT('Ctrl Pts',(4.33962418453247,0.106048354957064,11.7652934103049));
#18739=CARTESIAN_POINT('Ctrl Pts',(4.3390257792157,0.108954250606769,11.7659075794119));
#18740=CARTESIAN_POINT('Ctrl Pts',(4.33854297284435,0.111909057305692,11.7664032032109));
#18741=CARTESIAN_POINT('Ctrl Pts',(4.33817886051713,0.114893365392952,11.7667770031683));
#18742=CARTESIAN_POINT('',(4.23244376179554,0.0834501820051857,11.7677846774689));
#18743=CARTESIAN_POINT('',(4.33962418453247,0.106048354957064,11.7652934103049));
#18744=CARTESIAN_POINT('Origin',(4.28974268595947,0.0834503638580657,11.8236129344662));
#18745=CARTESIAN_POINT('Origin',(4.39309251486109,0.128651272185532,11.7104388275966));
#18746=CARTESIAN_POINT('Origin',(4.33906241113996,0.128640496010329,11.6584014009706));
#18747=CARTESIAN_POINT('Ctrl Pts',(4.1864400889711,0.599559286979599,11.7367177974007));
#18748=CARTESIAN_POINT('Ctrl Pts',(4.1886804737254,0.599217388237333,11.7419000771489));
#18749=CARTESIAN_POINT('Ctrl Pts',(4.19485662924956,0.59640540998248,11.7517403335914));
#18750=CARTESIAN_POINT('Ctrl Pts',(4.20959478601258,0.583418316193309,11.7648503721434));
#18751=CARTESIAN_POINT('Ctrl Pts',(4.22860122563327,0.56002441203863,11.7744735096015));
#18752=CARTESIAN_POINT('Ctrl Pts',(4.24226657406414,0.537814124752668,11.7783325570636));
#18753=CARTESIAN_POINT('Ctrl Pts',(4.24867356681529,0.525726490000265,11.7797315270537));
#18754=CARTESIAN_POINT('Ctrl Pts',(4.18952705913928,0.586463809002539,11.735700158011));
#18755=CARTESIAN_POINT('Ctrl Pts',(4.19137342751675,0.585902923557031,11.7399942324166));
#18756=CARTESIAN_POINT('Ctrl Pts',(4.19607564927109,0.582996738128302,11.7478909268382));
#18757=CARTESIAN_POINT('Ctrl Pts',(4.20718567353011,0.571444962213375,11.759339123899));
#18758=CARTESIAN_POINT('Ctrl Pts',(4.22315764354396,0.550663720789415,11.7694614446329));
#18759=CARTESIAN_POINT('Ctrl Pts',(4.23584186027139,0.530339176921929,11.7741901849771));
#18760=CARTESIAN_POINT('Ctrl Pts',(4.24189088815672,0.51917031525084,11.7759607223076));
#18761=CARTESIAN_POINT('Ctrl Pts',(4.18941786442921,0.5586701286686,11.7362685864366));
#18762=CARTESIAN_POINT('Ctrl Pts',(4.19047278915203,0.557673290482625,11.7393205950847));
#18763=CARTESIAN_POINT('Ctrl Pts',(4.19257132672879,0.554666512895981,11.7443495285969));
#18764=CARTESIAN_POINT('Ctrl Pts',(4.19793491703686,0.546370059453453,11.7532207324389));
#18765=CARTESIAN_POINT('Ctrl Pts',(4.20960649937055,0.531257609322764,11.763935815195));
#18766=CARTESIAN_POINT('Ctrl Pts',(4.22112932284417,0.514903265836773,11.7697717579804));
#18767=CARTESIAN_POINT('Ctrl Pts',(4.22676242995304,0.505649359848945,11.7720002083824));
#18768=CARTESIAN_POINT('Ctrl Pts',(4.16745842900663,0.516177609788138,11.7460636132259));
#18769=CARTESIAN_POINT('Ctrl Pts',(4.16745960968501,0.514934209415718,11.7493116799598));
#18770=CARTESIAN_POINT('Ctrl Pts',(4.16742526266361,0.512400102456327,11.754170815901));
#18771=CARTESIAN_POINT('Ctrl Pts',(4.1702424679982,0.508565778427457,11.7620313775964));
#18772=CARTESIAN_POINT('Ctrl Pts',(4.18112328052461,0.500936758529474,11.7716132782273));
#18773=CARTESIAN_POINT('Ctrl Pts',(4.19285904104883,0.490293107380878,11.776638091041));
#18774=CARTESIAN_POINT('Ctrl Pts',(4.19855158379117,0.483870890196332,11.7784814265239));
#18775=CARTESIAN_POINT('Ctrl Pts',(4.13708840011498,0.501283154238658,11.7587835155587));
#18776=CARTESIAN_POINT('Ctrl Pts',(4.13701026579034,0.500653265378882,11.7642021491914));
#18777=CARTESIAN_POINT('Ctrl Pts',(4.13829951247469,0.49908582037805,11.7733140929352));
#18778=CARTESIAN_POINT('Ctrl Pts',(4.14609086019466,0.495348174409366,11.7840463234316));
#18779=CARTESIAN_POINT('Ctrl Pts',(4.16138741638408,0.487734747778109,11.791448977135));
#18780=CARTESIAN_POINT('Ctrl Pts',(4.17444554632098,0.478374076350456,11.7937488231701));
#18781=CARTESIAN_POINT('Ctrl Pts',(4.18052929710018,0.472869402787525,11.7943760601066));
#18782=CARTESIAN_POINT('Ctrl Pts',(4.11838193196953,0.500422592509204,11.7664617086384));
#18783=CARTESIAN_POINT('Ctrl Pts',(4.11865168183635,0.500435001928776,11.7735428707743));
#18784=CARTESIAN_POINT('Ctrl Pts',(4.12165523740038,0.499626427226189,11.7860588810822));
#18785=CARTESIAN_POINT('Ctrl Pts',(4.13375709461643,0.494528711775158,11.7996999793846));
#18786=CARTESIAN_POINT('Ctrl Pts',(4.15222669835934,0.484505223058561,11.8062291222987));
#18787=CARTESIAN_POINT('Ctrl Pts',(4.16594264043612,0.474519610560075,11.8067214846143));
#18788=CARTESIAN_POINT('Ctrl Pts',(4.17218826315036,0.468962654353894,11.80651609725));
#18789=CARTESIAN_POINT('',(4.11838200569138,0.500422526122696,11.7664617661004));
#18790=CARTESIAN_POINT('Ctrl Pts',(4.20352712124656,0.513629536369044,11.7694536414083));
#18791=CARTESIAN_POINT('Ctrl Pts',(4.18960278591621,0.509898541151459,11.769080316127));
#18792=CARTESIAN_POINT('Ctrl Pts',(4.17615741309794,0.507139097066293,11.7705957934386));
#18793=CARTESIAN_POINT('Ctrl Pts',(4.15632514529375,0.503898993650465,11.7723830647377));
#18794=CARTESIAN_POINT('Ctrl Pts',(4.14962589610481,0.503026780112622,11.7727554305325));
#18795=CARTESIAN_POINT('Ctrl Pts',(4.1351819577934,0.501481089633748,11.7717516560017));
#18796=CARTESIAN_POINT('Ctrl Pts',(4.12736858237728,0.500845146597188,11.7702972624861));
#18797=CARTESIAN_POINT('Ctrl Pts',(4.11865840483925,0.500435383006644,11.7665811325368));
#18798=CARTESIAN_POINT('Ctrl Pts',(4.11852016115429,0.500428951553896,11.7665216619244));
#18799=CARTESIAN_POINT('Ctrl Pts',(4.11838201228193,0.500422596203858,11.7664617434719));
#18800=CARTESIAN_POINT('Ctrl Pts',(4.11838193425775,0.500422592614458,11.7664617687052));
#18801=CARTESIAN_POINT('Ctrl Pts',(4.11865169032903,0.500434999642494,11.7735429061638));
#18802=CARTESIAN_POINT('Ctrl Pts',(4.12165524766592,0.499626422901991,11.7860588926534));
#18803=CARTESIAN_POINT('Ctrl Pts',(4.13375709461643,0.494528711775158,11.7996999793846));
#18804=CARTESIAN_POINT('Ctrl Pts',(4.15222669835934,0.484505223058561,11.8062291222987));
#18805=CARTESIAN_POINT('Ctrl Pts',(4.16594264043612,0.474519610560075,11.8067214846143));
#18806=CARTESIAN_POINT('Ctrl Pts',(4.17218826315036,0.468962654353894,11.80651609725));
#18807=CARTESIAN_POINT('Ctrl Pts',(4.33962418453247,0.106048354957063,11.7652934103049));
#18808=CARTESIAN_POINT('Ctrl Pts',(4.34246949077866,0.0922313603362983,
11.7623731501614));
#18809=CARTESIAN_POINT('Ctrl Pts',(4.34745706311513,0.0672688955414189,
11.7459971874554));
#18810=CARTESIAN_POINT('Ctrl Pts',(4.3556551375003,0.0558301882629109,11.7196032056567));
#18811=CARTESIAN_POINT('Ctrl Pts',(4.36216987636126,0.0534615492574821,
11.7069738861294));
#18812=CARTESIAN_POINT('Ctrl Pts',(4.32223465297952,0.10564403284836,11.7502632334754));
#18813=CARTESIAN_POINT('Ctrl Pts',(4.32478575489734,0.095417896876601,11.748512775078));
#18814=CARTESIAN_POINT('Ctrl Pts',(4.3306965583525,0.0742071101490252,11.737276832848));
#18815=CARTESIAN_POINT('Ctrl Pts',(4.34109202085652,0.0611390274796559,
11.7121170913212));
#18816=CARTESIAN_POINT('Ctrl Pts',(4.34880635645981,0.0583202788559448,
11.6991691569315));
#18817=CARTESIAN_POINT('Ctrl Pts',(4.28058245277421,0.0997299260061634,
11.7376622728835));
#18818=CARTESIAN_POINT('Ctrl Pts',(4.28392629294866,0.092691693017298,11.7364042543565));
#18819=CARTESIAN_POINT('Ctrl Pts',(4.29468264038552,0.0750207280329448,
11.7276251801877));
#18820=CARTESIAN_POINT('Ctrl Pts',(4.31151716837604,0.0612211827675296,
11.7004931914203));
#18821=CARTESIAN_POINT('Ctrl Pts',(4.3224279424754,0.0584221672677555,11.6855429425366));
#18822=CARTESIAN_POINT('Ctrl Pts',(4.24398355505158,0.0883300248227467,
11.7559405420827));
#18823=CARTESIAN_POINT('Ctrl Pts',(4.24866969340974,0.0774044433934375,
11.7521028590549));
#18824=CARTESIAN_POINT('Ctrl Pts',(4.26266537403032,0.0561815068305335,
11.7323050480364));
#18825=CARTESIAN_POINT('Ctrl Pts',(4.28486228403869,0.0454021943366394,
11.6953979077451));
#18826=CARTESIAN_POINT('Ctrl Pts',(4.2989472341934,0.0439270963371727,11.6761491591203));
#18827=CARTESIAN_POINT('Ctrl Pts',(4.23244357912718,0.0834503638580655,
11.7677845155721));
#18828=CARTESIAN_POINT('Ctrl Pts',(4.23751751309539,0.0698384627757711,
11.7625769189705));
#18829=CARTESIAN_POINT('Ctrl Pts',(4.25171234512073,0.0457415007973147,
11.7367473849806));
#18830=CARTESIAN_POINT('Ctrl Pts',(4.27527634265085,0.0364965974668743,
11.6946834568217));
#18831=CARTESIAN_POINT('Ctrl Pts',(4.29045125549198,0.035695688094989,11.6733103800476));
#18832=CARTESIAN_POINT('',(4.29045125544124,0.0356956880470215,11.6733103800327));
#18833=CARTESIAN_POINT('',(4.36216987635991,0.0534615492579749,11.7069738861286));
#18834=CARTESIAN_POINT('Origin',(4.33483406961706,-0.0217232475410972,11.7069738861151));
#18835=CARTESIAN_POINT('Ctrl Pts',(4.36216987636126,0.0534615492574821,
11.7069738861294));
#18836=CARTESIAN_POINT('Ctrl Pts',(4.3556551375003,0.0558301882629109,11.7196032056567));
#18837=CARTESIAN_POINT('Ctrl Pts',(4.34745706311513,0.0672688955414189,
11.7459971874554));
#18838=CARTESIAN_POINT('Ctrl Pts',(4.34246949077866,0.0922313603362983,
11.7623731501614));
#18839=CARTESIAN_POINT('Ctrl Pts',(4.33962418453247,0.106048354957063,11.7652934103049));
#18840=CARTESIAN_POINT('Ctrl Pts',(4.23245081468777,0.0834309576742871,
11.7677770855905));
#18841=CARTESIAN_POINT('Ctrl Pts',(4.23752425974456,0.0698270114887331,
11.7625646425201));
#18842=CARTESIAN_POINT('Ctrl Pts',(4.2517179445374,0.0457393039686254,11.7367373895008));
#18843=CARTESIAN_POINT('Ctrl Pts',(4.27527634265085,0.0364965974668743,
11.6946834568217));
#18844=CARTESIAN_POINT('Ctrl Pts',(4.29045125549198,0.035695688094989,11.6733103800476));
#18845=CARTESIAN_POINT('Ctrl Pts',(4.34421258421314,0.0378725448121803,
11.5962093343554));
#18846=CARTESIAN_POINT('Ctrl Pts',(4.32681581897869,0.0356051827682455,
11.6219251290513));
#18847=CARTESIAN_POINT('Ctrl Pts',(4.30862493048636,0.0347365085016417,
11.64771370248));
#18848=CARTESIAN_POINT('Ctrl Pts',(4.29045125548377,0.0356956880906077,
11.673310380051));
#18849=CARTESIAN_POINT('Ctrl Pts',(4.35122162761644,0.0423700546448687,
11.5993028404662));
#18850=CARTESIAN_POINT('Ctrl Pts',(4.33537392032581,0.0418771635834138,
11.6257460902884));
#18851=CARTESIAN_POINT('Ctrl Pts',(4.31864236216508,0.0431620305839684,
11.6518872279534));
#18852=CARTESIAN_POINT('Ctrl Pts',(4.30177922708538,0.0466708990771757,
11.6770954188119));
#18853=CARTESIAN_POINT('Ctrl Pts',(4.36466668386284,0.0479840668591653,
11.605316017609));
#18854=CARTESIAN_POINT('Ctrl Pts',(4.35226885751852,0.0494632699189516,
11.6335433648312));
#18855=CARTESIAN_POINT('Ctrl Pts',(4.33918335764944,0.0531330803712445,
11.6611567729366));
#18856=CARTESIAN_POINT('Ctrl Pts',(4.32650404086796,0.0594318912603617,
11.6874561924858));
#18857=CARTESIAN_POINT('Ctrl Pts',(4.37888556984392,0.0491234947965908,
11.6118011873195));
#18858=CARTESIAN_POINT('Ctrl Pts',(4.37020796655163,0.0501668611945751,
11.6422225306338));
#18859=CARTESIAN_POINT('Ctrl Pts',(4.36099713174971,0.0527032630974422,
11.6720529183227));
#18860=CARTESIAN_POINT('Ctrl Pts',(4.35214723642143,0.0571055964480933,
11.7011203392195));
#18861=CARTESIAN_POINT('Ctrl Pts',(4.38493129402142,0.048777234595766,11.6145804154759));
#18862=CARTESIAN_POINT('Ctrl Pts',(4.37774644585057,0.0491887364932216,
11.6459417104654));
#18863=CARTESIAN_POINT('Ctrl Pts',(4.36997201320337,0.0506248360545129,
11.6767238081028));
#18864=CARTESIAN_POINT('Ctrl Pts',(4.36216987634685,0.0534615492511837,
11.7069738861159));
#18865=CARTESIAN_POINT('',(4.38493129402142,0.0487772345957665,11.6145804154759));
#18866=CARTESIAN_POINT('',(4.32736007730607,0.0514806398808873,11.6713697523917));
#18867=CARTESIAN_POINT('Ctrl Pts',(4.38493129402142,0.048777234595766,11.6145804154759));
#18868=CARTESIAN_POINT('Ctrl Pts',(4.37601770603885,0.0492877475921092,
11.6232421393828));
#18869=CARTESIAN_POINT('Ctrl Pts',(4.3668693999289,0.049677922134395,11.632197583949));
#18870=CARTESIAN_POINT('Ctrl Pts',(4.35762739235915,0.0500769766269212,
11.6413098490428));
#18871=CARTESIAN_POINT('Ctrl Pts',(4.35431874628973,0.0502198384530139,
11.6445720472024));
#18872=CARTESIAN_POINT('Ctrl Pts',(4.35101123017846,0.0503624490374187,
11.6478412754132));
#18873=CARTESIAN_POINT('Ctrl Pts',(4.34770259990182,0.0505083669896217,
11.6511194166589));
#18874=CARTESIAN_POINT('Ctrl Pts',(4.3409327813208,0.0508069310422763,11.6578268513558));
#18875=CARTESIAN_POINT('Ctrl Pts',(4.33415830379631,0.051119715599887,11.6645715917699));
#18876=CARTESIAN_POINT('Ctrl Pts',(4.32736007730607,0.0514806398808858,
11.6713697523917));
#18877=CARTESIAN_POINT('Ctrl Pts',(4.38493129402142,0.048777234595766,11.6145804154759));
#18878=CARTESIAN_POINT('Ctrl Pts',(4.37774644585057,0.0491887364932216,
11.6459417104654));
#18879=CARTESIAN_POINT('Ctrl Pts',(4.36997201320337,0.0506248360545129,
11.6767238081028));
#18880=CARTESIAN_POINT('Ctrl Pts',(4.36216987634685,0.0534615492511837,
11.7069738861159));
#18881=CARTESIAN_POINT('',(4.33139507209999,0.0364734805255282,11.6149738861246));
#18882=CARTESIAN_POINT('Ctrl Pts',(4.29045125548377,0.0356956880906077,
11.673310380051));
#18883=CARTESIAN_POINT('Ctrl Pts',(4.30420562082409,0.0349697531054306,
11.6539380706662));
#18884=CARTESIAN_POINT('Ctrl Pts',(4.31796984588305,0.0352907949390317,
11.63445584521));
#18885=CARTESIAN_POINT('Ctrl Pts',(4.33139221270344,0.0364727682572349,
11.614978441252));
#18886=CARTESIAN_POINT('Ctrl Pts',(4.32736007730609,0.051480639880892,11.6713697523917));
#18887=CARTESIAN_POINT('Ctrl Pts',(4.32798253826001,0.0491575839751223,
11.6619619576146));
#18888=CARTESIAN_POINT('Ctrl Pts',(4.32862960298899,0.0467427055308035,
11.6524786614797));
#18889=CARTESIAN_POINT('Ctrl Pts',(4.3299579720458,0.0417851647195623,11.6337717205853));
#18890=CARTESIAN_POINT('Ctrl Pts',(4.33065634771171,0.0391787912516445,
11.6243066674654));
#18891=CARTESIAN_POINT('Ctrl Pts',(4.33138167302864,0.0364718403168447,
11.614993735436));
#18892=CARTESIAN_POINT('Ctrl Pts',(4.44483865181741,0.143472770337244,11.7628168777948));
#18893=CARTESIAN_POINT('Ctrl Pts',(4.31439385308573,0.630299386786979,11.7628168777948));
#18894=CARTESIAN_POINT('Ctrl Pts',(4.42917451869962,0.1392755785182,11.7794523105961));
#18895=CARTESIAN_POINT('Ctrl Pts',(4.29872971996794,0.626102194967936,11.7794523105961));
#18896=CARTESIAN_POINT('Ctrl Pts',(4.38897935642072,0.128505317245929,11.7951014042888));
#18897=CARTESIAN_POINT('Ctrl Pts',(4.25853455768904,0.615331933695665,11.7951014042888));
#18898=CARTESIAN_POINT('Ctrl Pts',(4.35076008096908,0.118264493253361,11.7783502649473));
#18899=CARTESIAN_POINT('Ctrl Pts',(4.2203152822374,0.605091109703097,11.7783502649473));
#18900=CARTESIAN_POINT('Ctrl Pts',(4.33817886049864,0.114893365388508,11.7667770031876));
#18901=CARTESIAN_POINT('Ctrl Pts',(4.20773406176696,0.601719981838243,11.7667770031876));
#18902=CARTESIAN_POINT('',(4.44483865181741,0.143472770337245,11.7628168777948));
#18903=CARTESIAN_POINT('Origin',(4.38950568308719,0.128646346051165,11.706973886163));
#18904=CARTESIAN_POINT('',(4.44483865181741,0.143472770337244,11.7628168777948));
#18905=CARTESIAN_POINT('Origin',(4.38950568310546,0.128646346056062,11.7069738861436));
#18906=CARTESIAN_POINT('Origin',(4.38950568308719,0.128646346051166,11.7069738861252));
#18907=CARTESIAN_POINT('Origin',(4.38950568310546,0.128646346056062,11.7069738861436));
#18908=CARTESIAN_POINT('Origin',(4.38950568308719,0.128646346051166,5.29092677993983));
#18909=CARTESIAN_POINT('Origin',(4.38948772286522,0.129021219720988,11.6136857339278));
#18910=CARTESIAN_POINT('Ctrl Pts',(4.08617023400024,-0.552060840994624,
11.9163435012344));
#18911=CARTESIAN_POINT('Ctrl Pts',(4.08617023400024,1.61522066995007,11.9163435012344));
#18912=CARTESIAN_POINT('Ctrl Pts',(4.10576511646638,-0.552060840994624,
11.8970344456328));
#18913=CARTESIAN_POINT('Ctrl Pts',(4.10576511646638,1.61522066995007,11.8970344456328));
#18914=CARTESIAN_POINT('Ctrl Pts',(4.15149421914094,-0.552060840994624,
11.8511956487512));
#18915=CARTESIAN_POINT('Ctrl Pts',(4.15149421914094,1.61522066995007,11.8511956487512));
#18916=CARTESIAN_POINT('Ctrl Pts',(4.22408937937455,-0.552060840994624,
11.7763607682953));
#18917=CARTESIAN_POINT('Ctrl Pts',(4.22408937937455,1.61522066995007,11.7763607682953));
#18918=CARTESIAN_POINT('Ctrl Pts',(4.3260071847331,-0.552060840994624,11.6707401393954));
#18919=CARTESIAN_POINT('Ctrl Pts',(4.3260071847331,1.61522066995007,11.6707401393954));
#18920=CARTESIAN_POINT('Ctrl Pts',(4.46255574628753,-0.552060840994624,
11.5373242211525));
#18921=CARTESIAN_POINT('Ctrl Pts',(4.46255574628753,1.61522066995007,11.5373242211525));
#18922=CARTESIAN_POINT('Ctrl Pts',(4.61532593596939,-0.552060840994624,
11.4029224160728));
#18923=CARTESIAN_POINT('Ctrl Pts',(4.61532593596939,1.61522066995007,11.4029224160728));
#18924=CARTESIAN_POINT('Ctrl Pts',(4.77596612414944,-0.552060840994624,
11.2768795166233));
#18925=CARTESIAN_POINT('Ctrl Pts',(4.77596612414944,1.61522066995007,11.2768795166233));
#18926=CARTESIAN_POINT('Ctrl Pts',(4.94211773226968,-0.552060840994624,
11.1598106424589));
#18927=CARTESIAN_POINT('Ctrl Pts',(4.94211773226968,1.61522066995007,11.1598106424589));
#18928=CARTESIAN_POINT('Ctrl Pts',(5.11112998264613,-0.552060840994624,
11.051370419133));
#18929=CARTESIAN_POINT('Ctrl Pts',(5.11112998264613,1.61522066995007,11.051370419133));
#18930=CARTESIAN_POINT('Ctrl Pts',(5.28082876351925,-0.552060840994624,
10.9511663773825));
#18931=CARTESIAN_POINT('Ctrl Pts',(5.28082876351925,1.61522066995007,10.9511663773825));
#18932=CARTESIAN_POINT('Ctrl Pts',(5.45051506148977,-0.552060840994624,
10.8599381259735));
#18933=CARTESIAN_POINT('Ctrl Pts',(5.45051506148977,1.61522066995007,10.8599381259735));
#18934=CARTESIAN_POINT('Ctrl Pts',(5.62101499943423,-0.552060840994624,
10.7795199127532));
#18935=CARTESIAN_POINT('Ctrl Pts',(5.62101499943423,1.61522066995007,10.7795199127532));
#18936=CARTESIAN_POINT('Ctrl Pts',(5.7936769541502,-0.552060840994624,10.7114411549111));
#18937=CARTESIAN_POINT('Ctrl Pts',(5.7936769541502,1.61522066995007,10.7114411549111));
#18938=CARTESIAN_POINT('Ctrl Pts',(5.96961932707136,-0.552060840994624,
10.6558377434042));
#18939=CARTESIAN_POINT('Ctrl Pts',(5.96961932707136,1.61522066995007,10.6558377434042));
#18940=CARTESIAN_POINT('Ctrl Pts',(6.14893768388704,-0.552060840994624,
10.6103475969888));
#18941=CARTESIAN_POINT('Ctrl Pts',(6.14893768388704,1.61522066995007,10.6103475969888));
#18942=CARTESIAN_POINT('Ctrl Pts',(6.32976796473819,-0.552060840994624,
10.5687216653907));
#18943=CARTESIAN_POINT('Ctrl Pts',(6.32976796473819,1.61522066995007,10.5687216653907));
#18944=CARTESIAN_POINT('Ctrl Pts',(6.50892555577775,-0.552060840994624,
10.5222908830264));
#18945=CARTESIAN_POINT('Ctrl Pts',(6.50892555577775,1.61522066995007,10.5222908830264));
#18946=CARTESIAN_POINT('Ctrl Pts',(6.68288828293941,-0.552060840994624,
10.462050267878));
#18947=CARTESIAN_POINT('Ctrl Pts',(6.68288828293941,1.61522066995007,10.462050267878));
#18948=CARTESIAN_POINT('Ctrl Pts',(6.84859008776107,-0.552060840994624,
10.3804015453596));
#18949=CARTESIAN_POINT('Ctrl Pts',(6.84859008776107,1.61522066995007,10.3804015453596));
#18950=CARTESIAN_POINT('Ctrl Pts',(7.00445448641038,-0.552060840994624,
10.2733319413005));
#18951=CARTESIAN_POINT('Ctrl Pts',(7.00445448641038,1.61522066995007,10.2733319413005));
#18952=CARTESIAN_POINT('Ctrl Pts',(7.15081550722288,-0.552060840994624,
10.1414720974144));
#18953=CARTESIAN_POINT('Ctrl Pts',(7.15081550722288,1.61522066995007,10.1414720974144));
#18954=CARTESIAN_POINT('Ctrl Pts',(7.28883796912684,-0.552060840994624,
9.98835756998534));
#18955=CARTESIAN_POINT('Ctrl Pts',(7.28883796912684,1.61522066995007,9.98835756998534));
#18956=CARTESIAN_POINT('Ctrl Pts',(7.41967047354988,-0.552060840994624,
9.81917361987377));
#18957=CARTESIAN_POINT('Ctrl Pts',(7.41967047354988,1.61522066995007,9.81917361987377));
#18958=CARTESIAN_POINT('Ctrl Pts',(7.54360573526532,-0.552060840994624,
9.63939026966049));
#18959=CARTESIAN_POINT('Ctrl Pts',(7.54360573526532,1.61522066995007,9.63939026966049));
#18960=CARTESIAN_POINT('Ctrl Pts',(7.6590003866074,-0.552060840994624,9.45324999450471));
#18961=CARTESIAN_POINT('Ctrl Pts',(7.6590003866074,1.61522066995007,9.45324999450471));
#18962=CARTESIAN_POINT('Ctrl Pts',(7.76209282457502,-0.552060840994624,
9.26297089919836));
#18963=CARTESIAN_POINT('Ctrl Pts',(7.76209282457502,1.61522066995007,9.26297089919836));
#18964=CARTESIAN_POINT('Ctrl Pts',(7.84862074946283,-0.552060840994624,
9.06945407017055));
#18965=CARTESIAN_POINT('Ctrl Pts',(7.84862074946283,1.61522066995007,9.06945407017055));
#18966=CARTESIAN_POINT('Ctrl Pts',(7.91508259073031,-0.552060840994624,
8.87266947141857));
#18967=CARTESIAN_POINT('Ctrl Pts',(7.91508259073031,1.61522066995007,8.87266947141857));
#18968=CARTESIAN_POINT('Ctrl Pts',(7.96007609558387,-0.552060840994624,
8.67216210283894));
#18969=CARTESIAN_POINT('Ctrl Pts',(7.96007609558387,1.61522066995007,8.67216210283894));
#18970=CARTESIAN_POINT('Ctrl Pts',(7.98575825096082,-0.552060840994624,
8.46752658699496));
#18971=CARTESIAN_POINT('Ctrl Pts',(7.98575825096082,1.61522066995007,8.46752658699496));
#18972=CARTESIAN_POINT('Ctrl Pts',(7.9987984391963,-0.552060840994624,8.25883677791438));
#18973=CARTESIAN_POINT('Ctrl Pts',(7.9987984391963,1.61522066995007,8.25883677791438));
#18974=CARTESIAN_POINT('Ctrl Pts',(8.00781893805568,-0.552060840994624,
8.04662057355209));
#18975=CARTESIAN_POINT('Ctrl Pts',(8.00781893805568,1.61522066995007,8.04662057355209));
#18976=CARTESIAN_POINT('Ctrl Pts',(8.02124364536257,-0.552060840994624,
7.8318867323277));
#18977=CARTESIAN_POINT('Ctrl Pts',(8.02124364536257,1.61522066995007,7.8318867323277));
#18978=CARTESIAN_POINT('Ctrl Pts',(8.04494633492827,-0.552060840994624,
7.61613341658679));
#18979=CARTESIAN_POINT('Ctrl Pts',(8.04494633492827,1.61522066995007,7.61613341658679));
#18980=CARTESIAN_POINT('Ctrl Pts',(8.08008348678094,-0.552060840994624,
7.40136016279815));
#18981=CARTESIAN_POINT('Ctrl Pts',(8.08008348678094,1.61522066995007,7.40136016279815));
#18982=CARTESIAN_POINT('Ctrl Pts',(8.12057943633426,-0.552060840994624,
7.19009032473197));
#18983=CARTESIAN_POINT('Ctrl Pts',(8.12057943633426,1.61522066995007,7.19009032473197));
#18984=CARTESIAN_POINT('Ctrl Pts',(8.15569042861283,-0.552060840994624,
6.98516923427904));
#18985=CARTESIAN_POINT('Ctrl Pts',(8.15569042861283,1.61522066995007,6.98516923427904));
#18986=CARTESIAN_POINT('Ctrl Pts',(8.17293082304204,-0.552060840994624,
6.78954489191915));
#18987=CARTESIAN_POINT('Ctrl Pts',(8.17293082304204,1.61522066995007,6.78954489191915));
#18988=CARTESIAN_POINT('Ctrl Pts',(8.16089752265956,-0.552060840994624,
6.60605451948904));
#18989=CARTESIAN_POINT('Ctrl Pts',(8.16089752265956,1.61522066995007,6.60605451948904));
#18990=CARTESIAN_POINT('Ctrl Pts',(8.11207116917844,-0.552060840994624,
6.43720976255638));
#18991=CARTESIAN_POINT('Ctrl Pts',(8.11207116917844,1.61522066995007,6.43720976255638));
#18992=CARTESIAN_POINT('Ctrl Pts',(8.02580908828092,-0.552060840994624,
6.28498018271691));
#18993=CARTESIAN_POINT('Ctrl Pts',(8.02580908828092,1.61522066995007,6.28498018271691));
#18994=CARTESIAN_POINT('Ctrl Pts',(7.90644860448881,-0.552060840994624,
6.15052660592943));
#18995=CARTESIAN_POINT('Ctrl Pts',(7.90644860448881,1.61522066995007,6.15052660592943));
#18996=CARTESIAN_POINT('Ctrl Pts',(7.76106756457749,-0.552060840994624,
6.03389995867286));
#18997=CARTESIAN_POINT('Ctrl Pts',(7.76106756457749,1.61522066995007,6.03389995867286));
#18998=CARTESIAN_POINT('Ctrl Pts',(7.59751903688427,-0.552060840994624,
5.93381436957244));
#18999=CARTESIAN_POINT('Ctrl Pts',(7.59751903688427,1.61522066995007,5.93381436957244));
#19000=CARTESIAN_POINT('Ctrl Pts',(7.42198551710643,-0.552060840994624,
5.84723737025948));
#19001=CARTESIAN_POINT('Ctrl Pts',(7.42198551710643,1.61522066995007,5.84723737025948));
#19002=CARTESIAN_POINT('Ctrl Pts',(7.23853768475023,-0.552060840994624,
5.76979878895671));
#19003=CARTESIAN_POINT('Ctrl Pts',(7.23853768475023,1.61522066995007,5.76979878895671));
#19004=CARTESIAN_POINT('Ctrl Pts',(7.04976847947264,-0.552060840994624,
5.69662713609756));
#19005=CARTESIAN_POINT('Ctrl Pts',(7.04976847947264,1.61522066995007,5.69662713609756));
#19006=CARTESIAN_POINT('Ctrl Pts',(6.85709976037512,-0.552060840994624,
5.62308582598972));
#19007=CARTESIAN_POINT('Ctrl Pts',(6.85709976037512,1.61522066995007,5.62308582598972));
#19008=CARTESIAN_POINT('Ctrl Pts',(6.66121503090593,-0.552060840994624,
5.54547963906641));
#19009=CARTESIAN_POINT('Ctrl Pts',(6.66121503090593,1.61522066995007,5.54547963906641));
#19010=CARTESIAN_POINT('Ctrl Pts',(6.46246210121974,-0.552060840994624,
5.46195513100458));
#19011=CARTESIAN_POINT('Ctrl Pts',(6.46246210121974,1.61522066995007,5.46195513100458));
#19012=CARTESIAN_POINT('Ctrl Pts',(6.26112587698791,-0.552060840994624,
5.37226655127806));
#19013=CARTESIAN_POINT('Ctrl Pts',(6.26112587698791,1.61522066995007,5.37226655127806));
#19014=CARTESIAN_POINT('Ctrl Pts',(6.05762450882876,-0.552060840994624,
5.27709955371581));
#19015=CARTESIAN_POINT('Ctrl Pts',(6.05762450882876,1.61522066995007,5.27709955371581));
#19016=CARTESIAN_POINT('Ctrl Pts',(5.85274048349253,-0.552060840994624,
5.17752467829117));
#19017=CARTESIAN_POINT('Ctrl Pts',(5.85274048349253,1.61522066995007,5.17752467829117));
#19018=CARTESIAN_POINT('Ctrl Pts',(5.6478173738032,-0.552060840994624,5.07442896098936));
#19019=CARTESIAN_POINT('Ctrl Pts',(5.6478173738032,1.61522066995007,5.07442896098936));
#19020=CARTESIAN_POINT('Ctrl Pts',(5.44501860313336,-0.552060840994624,
4.96787993373722));
#19021=CARTESIAN_POINT('Ctrl Pts',(5.44501860313336,1.61522066995007,4.96787993373722));
#19022=CARTESIAN_POINT('Ctrl Pts',(5.24741086000008,-0.552060840994624,
4.85676111532844));
#19023=CARTESIAN_POINT('Ctrl Pts',(5.24741086000008,1.61522066995007,4.85676111532844));
#19024=CARTESIAN_POINT('Ctrl Pts',(5.05850630701875,-0.552060840994624,
4.73929437247794));
#19025=CARTESIAN_POINT('Ctrl Pts',(5.05850630701875,1.61522066995007,4.73929437247794));
#19026=CARTESIAN_POINT('Ctrl Pts',(4.88190185104846,-0.552060840994624,
4.61340315498245));
#19027=CARTESIAN_POINT('Ctrl Pts',(4.88190185104846,1.61522066995007,4.61340315498245));
#19028=CARTESIAN_POINT('Ctrl Pts',(4.7208720035032,-0.552060840994624,4.47714872481864));
#19029=CARTESIAN_POINT('Ctrl Pts',(4.7208720035032,1.61522066995007,4.47714872481864));
#19030=CARTESIAN_POINT('Ctrl Pts',(4.57800047823784,-0.552060840994624,
4.32911151507775));
#19031=CARTESIAN_POINT('Ctrl Pts',(4.57800047823784,1.61522066995007,4.32911151507775));
#19032=CARTESIAN_POINT('Ctrl Pts',(4.4547451964031,-0.552060840994624,4.16885849319143));
#19033=CARTESIAN_POINT('Ctrl Pts',(4.4547451964031,1.61522066995007,4.16885849319143));
#19034=CARTESIAN_POINT('Ctrl Pts',(4.35148411330737,-0.552060840994624,
3.99681013615577));
#19035=CARTESIAN_POINT('Ctrl Pts',(4.35148411330737,1.61522066995007,3.99681013615577));
#19036=CARTESIAN_POINT('Ctrl Pts',(4.26765207024408,-0.552060840994624,
3.81399668859083));
#19037=CARTESIAN_POINT('Ctrl Pts',(4.26765207024408,1.61522066995007,3.81399668859083));
#19038=CARTESIAN_POINT('Ctrl Pts',(4.20184334854117,-0.552060840994624,
3.62185203209172));
#19039=CARTESIAN_POINT('Ctrl Pts',(4.20184334854117,1.61522066995007,3.62185203209172));
#19040=CARTESIAN_POINT('Ctrl Pts',(4.15193466045737,-0.552060840994624,
3.42199345348454));
#19041=CARTESIAN_POINT('Ctrl Pts',(4.15193466045737,1.61522066995007,3.42199345348454));
#19042=CARTESIAN_POINT('Ctrl Pts',(4.11518318246501,-0.552060840994624,
3.21600287470933));
#19043=CARTESIAN_POINT('Ctrl Pts',(4.11518318246501,1.61522066995007,3.21600287470933));
#19044=CARTESIAN_POINT('Ctrl Pts',(4.08854433447712,-0.552060840994624,
3.00529120729351));
#19045=CARTESIAN_POINT('Ctrl Pts',(4.08854433447712,1.61522066995007,3.00529120729351));
#19046=CARTESIAN_POINT('Ctrl Pts',(4.06899962712481,-0.552060840994624,
2.7909834104826));
#19047=CARTESIAN_POINT('Ctrl Pts',(4.06899962712481,1.61522066995007,2.7909834104826));
#19048=CARTESIAN_POINT('Ctrl Pts',(4.05390260344518,-0.552060840994624,
2.57377631141663));
#19049=CARTESIAN_POINT('Ctrl Pts',(4.05390260344518,1.61522066995007,2.57377631141663));
#19050=CARTESIAN_POINT('Ctrl Pts',(4.04126813644791,-0.552060840994624,
2.35385258470204));
#19051=CARTESIAN_POINT('Ctrl Pts',(4.04126813644791,1.61522066995007,2.35385258470204));
#19052=CARTESIAN_POINT('Ctrl Pts',(4.03021014446877,-0.552060840994624,
2.13065748555701));
#19053=CARTESIAN_POINT('Ctrl Pts',(4.03021014446877,1.61522066995007,2.13065748555701));
#19054=CARTESIAN_POINT('Ctrl Pts',(4.02066709528519,-0.552060840994624,
1.9033255681334));
#19055=CARTESIAN_POINT('Ctrl Pts',(4.02066709528519,1.61522066995007,1.9033255681334));
#19056=CARTESIAN_POINT('Ctrl Pts',(4.012782399266,-0.552060840994624,1.67142113207676));
#19057=CARTESIAN_POINT('Ctrl Pts',(4.012782399266,1.61522066995007,1.67142113207676));
#19058=CARTESIAN_POINT('Ctrl Pts',(4.00639322616619,-0.552060840994624,
1.4355810193293));
#19059=CARTESIAN_POINT('Ctrl Pts',(4.00639322616619,1.61522066995007,1.4355810193293));
#19060=CARTESIAN_POINT('Ctrl Pts',(4.00047520099043,-0.552060840994624,
1.19819542279832));
#19061=CARTESIAN_POINT('Ctrl Pts',(4.00047520099043,1.61522066995007,1.19819542279832));
#19062=CARTESIAN_POINT('Ctrl Pts',(3.99260375067002,-0.552060840994624,
0.964078729991153));
#19063=CARTESIAN_POINT('Ctrl Pts',(3.99260375067002,1.61522066995007,0.964078729991153));
#19064=CARTESIAN_POINT('Ctrl Pts',(3.97841403016118,-0.552060840994624,
0.741129277895168));
#19065=CARTESIAN_POINT('Ctrl Pts',(3.97841403016118,1.61522066995007,0.741129277895168));
#19066=CARTESIAN_POINT('Ctrl Pts',(3.95259200169988,-0.552060840994624,
0.538436816836329));
#19067=CARTESIAN_POINT('Ctrl Pts',(3.95259200169988,1.61522066995007,0.538436816836329));
#19068=CARTESIAN_POINT('Ctrl Pts',(3.90986572419832,-0.552060840994624,
0.364350357241537));
#19069=CARTESIAN_POINT('Ctrl Pts',(3.90986572419832,1.61522066995007,0.364350357241537));
#19070=CARTESIAN_POINT('Ctrl Pts',(3.84598208672298,-0.552060840994624,
0.224659532804428));
#19071=CARTESIAN_POINT('Ctrl Pts',(3.84598208672298,1.61522066995007,0.224659532804428));
#19072=CARTESIAN_POINT('Ctrl Pts',(3.75872318140661,-0.552060840994624,
0.120497232333236));
#19073=CARTESIAN_POINT('Ctrl Pts',(3.75872318140661,1.61522066995007,0.120497232333236));
#19074=CARTESIAN_POINT('Ctrl Pts',(3.64881642260075,-0.552060840994624,
0.0470540298718229));
#19075=CARTESIAN_POINT('Ctrl Pts',(3.64881642260075,1.61522066995007,0.0470540298718229));
#19076=CARTESIAN_POINT('Ctrl Pts',(3.52045328348988,-0.552060840994624,
-0.00118366394786523));
#19077=CARTESIAN_POINT('Ctrl Pts',(3.52045328348988,1.61522066995007,-0.00118366394786523));
#19078=CARTESIAN_POINT('Ctrl Pts',(3.3816469894381,-0.552060840994624,-0.0263068037111615));
#19079=CARTESIAN_POINT('Ctrl Pts',(3.3816469894381,1.61522066995007,-0.0263068037111615));
#19080=CARTESIAN_POINT('Ctrl Pts',(3.2451100102617,-0.552060840994624,-0.0214179570895094));
#19081=CARTESIAN_POINT('Ctrl Pts',(3.2451100102617,1.61522066995007,-0.0214179570895094));
#19082=CARTESIAN_POINT('Ctrl Pts',(3.12452733970665,-0.552060840994624,
0.0241851999814078));
#19083=CARTESIAN_POINT('Ctrl Pts',(3.12452733970665,1.61522066995007,0.0241851999814078));
#19084=CARTESIAN_POINT('Ctrl Pts',(3.03063129752059,-0.552060840994624,
0.119017371327004));
#19085=CARTESIAN_POINT('Ctrl Pts',(3.03063129752059,1.61522066995007,0.119017371327004));
#19086=CARTESIAN_POINT('Ctrl Pts',(2.96639254265844,-0.552060840994624,
0.262319630540593));
#19087=CARTESIAN_POINT('Ctrl Pts',(2.96639254265844,1.61522066995007,0.262319630540593));
#19088=CARTESIAN_POINT('Ctrl Pts',(2.92780415844446,-0.552060840994624,
0.444963858672424));
#19089=CARTESIAN_POINT('Ctrl Pts',(2.92780415844446,1.61522066995007,0.444963858672424));
#19090=CARTESIAN_POINT('Ctrl Pts',(2.90717911786689,-0.552060840994624,
0.65402023086958));
#19091=CARTESIAN_POINT('Ctrl Pts',(2.90717911786689,1.61522066995007,0.65402023086958));
#19092=CARTESIAN_POINT('Ctrl Pts',(2.89547076625581,-0.552060840994624,
0.875890304828918));
#19093=CARTESIAN_POINT('Ctrl Pts',(2.89547076625581,1.61522066995007,0.875890304828918));
#19094=CARTESIAN_POINT('Ctrl Pts',(2.88537704766906,-0.552060840994624,
1.10060381648398));
#19095=CARTESIAN_POINT('Ctrl Pts',(2.88537704766906,1.61522066995007,1.10060381648398));
#19096=CARTESIAN_POINT('Ctrl Pts',(2.8728456296504,-0.552060840994624,1.32371934078733));
#19097=CARTESIAN_POINT('Ctrl Pts',(2.8728456296504,1.61522066995007,1.32371934078733));
#19098=CARTESIAN_POINT('Ctrl Pts',(2.85578261679345,-0.552060840994624,
1.54401727992264));
#19099=CARTESIAN_POINT('Ctrl Pts',(2.85578261679345,1.61522066995007,1.54401727992264));
#19100=CARTESIAN_POINT('Ctrl Pts',(2.83335686249019,-0.552060840994624,
1.76209503442146));
#19101=CARTESIAN_POINT('Ctrl Pts',(2.83335686249019,1.61522066995007,1.76209503442146));
#19102=CARTESIAN_POINT('Ctrl Pts',(2.80505146480345,-0.552060840994624,
1.97856787413951));
#19103=CARTESIAN_POINT('Ctrl Pts',(2.80505146480345,1.61522066995007,1.97856787413951));
#19104=CARTESIAN_POINT('Ctrl Pts',(2.76985908233915,-0.552060840994624,
2.19251877196071));
#19105=CARTESIAN_POINT('Ctrl Pts',(2.76985908233915,1.61522066995007,2.19251877196071));
#19106=CARTESIAN_POINT('Ctrl Pts',(2.72531955636536,-0.552060840994624,
2.39962532458029));
#19107=CARTESIAN_POINT('Ctrl Pts',(2.72531955636536,1.61522066995007,2.39962532458029));
#19108=CARTESIAN_POINT('Ctrl Pts',(2.66797634363184,-0.552060840994624,
2.59347738935741));
#19109=CARTESIAN_POINT('Ctrl Pts',(2.66797634363184,1.61522066995007,2.59347738935741));
#19110=CARTESIAN_POINT('Ctrl Pts',(2.59397540849171,-0.552060840994624,
2.7672283971178));
#19111=CARTESIAN_POINT('Ctrl Pts',(2.59397540849171,1.61522066995007,2.7672283971178));
#19112=CARTESIAN_POINT('Ctrl Pts',(2.49960870420485,-0.552060840994624,
2.91510580081997));
#19113=CARTESIAN_POINT('Ctrl Pts',(2.49960870420485,1.61522066995007,2.91510580081997));
#19114=CARTESIAN_POINT('Ctrl Pts',(2.38189256086504,-0.552060840994624,
3.03403241435618));
#19115=CARTESIAN_POINT('Ctrl Pts',(2.38189256086504,1.61522066995007,3.03403241435618));
#19116=CARTESIAN_POINT('Ctrl Pts',(2.23909845280558,-0.552060840994624,
3.12505646843308));
#19117=CARTESIAN_POINT('Ctrl Pts',(2.23909845280558,1.61522066995007,3.12505646843308));
#19118=CARTESIAN_POINT('Ctrl Pts',(2.07061055216582,-0.552060840994624,
3.19196918412265));
#19119=CARTESIAN_POINT('Ctrl Pts',(2.07061055216582,1.61522066995007,3.19196918412265));
#19120=CARTESIAN_POINT('Ctrl Pts',(1.87681490437036,-0.552060840994624,
3.24001322621211));
#19121=CARTESIAN_POINT('Ctrl Pts',(1.87681490437036,1.61522066995007,3.24001322621211));
#19122=CARTESIAN_POINT('Ctrl Pts',(1.65897747541321,-0.552060840994624,
3.27464765209773));
#19123=CARTESIAN_POINT('Ctrl Pts',(1.65897747541321,1.61522066995007,3.27464765209773));
#19124=CARTESIAN_POINT('Ctrl Pts',(1.4191255439272,-0.552060840994624,3.30006519349576));
#19125=CARTESIAN_POINT('Ctrl Pts',(1.4191255439272,1.61522066995007,3.30006519349576));
#19126=CARTESIAN_POINT('Ctrl Pts',(1.15993538533448,-0.552060840994624,
3.31897283641381));
#19127=CARTESIAN_POINT('Ctrl Pts',(1.15993538533448,1.61522066995007,3.31897283641381));
#19128=CARTESIAN_POINT('Ctrl Pts',(0.884625090385968,-0.552060840994624,
3.33300441174764));
#19129=CARTESIAN_POINT('Ctrl Pts',(0.884625090385968,1.61522066995007,3.33300441174764));
#19130=CARTESIAN_POINT('Ctrl Pts',(0.596845720618978,-0.552060840994624,
3.34293392264922));
#19131=CARTESIAN_POINT('Ctrl Pts',(0.596845720618978,1.61522066995007,3.34293392264922));
#19132=CARTESIAN_POINT('Ctrl Pts',(0.30057321210183,-0.552060840994624,
3.34897162637417));
#19133=CARTESIAN_POINT('Ctrl Pts',(0.30057321210183,1.61522066995007,3.34897162637417));
#19134=CARTESIAN_POINT('Ctrl Pts',(1.66741620510891E-14,-0.552060840994624,
3.35102435732185));
#19135=CARTESIAN_POINT('Ctrl Pts',(1.66741620510891E-14,1.61522066995007,
3.35102435732185));
#19136=CARTESIAN_POINT('Ctrl Pts',(-0.300573212101791,-0.552060840994624,
3.34897162637426));
#19137=CARTESIAN_POINT('Ctrl Pts',(-0.300573212101791,1.61522066995007,
3.34897162637426));
#19138=CARTESIAN_POINT('Ctrl Pts',(-0.596845720618908,-0.552060840994624,
3.34293392264938));
#19139=CARTESIAN_POINT('Ctrl Pts',(-0.596845720618908,1.61522066995007,
3.34293392264938));
#19140=CARTESIAN_POINT('Ctrl Pts',(-0.884625090385886,-0.552060840994624,
3.33300441174785));
#19141=CARTESIAN_POINT('Ctrl Pts',(-0.884625090385886,1.61522066995007,
3.33300441174785));
#19142=CARTESIAN_POINT('Ctrl Pts',(-1.15993538533442,-0.552060840994624,
3.31897283641402));
#19143=CARTESIAN_POINT('Ctrl Pts',(-1.15993538533442,1.61522066995007,3.31897283641402));
#19144=CARTESIAN_POINT('Ctrl Pts',(-1.41912554392716,-0.552060840994624,
3.30006519349591));
#19145=CARTESIAN_POINT('Ctrl Pts',(-1.41912554392716,1.61522066995007,3.30006519349591));
#19146=CARTESIAN_POINT('Ctrl Pts',(-1.65897747541319,-0.552060840994624,
3.27464765209779));
#19147=CARTESIAN_POINT('Ctrl Pts',(-1.65897747541319,1.61522066995007,3.27464765209779));
#19148=CARTESIAN_POINT('Ctrl Pts',(-1.87681490437034,-0.552060840994624,
3.24001322621208));
#19149=CARTESIAN_POINT('Ctrl Pts',(-1.87681490437034,1.61522066995007,3.24001322621208));
#19150=CARTESIAN_POINT('Ctrl Pts',(-2.07061055216576,-0.552060840994624,
3.19196918412254));
#19151=CARTESIAN_POINT('Ctrl Pts',(-2.07061055216576,1.61522066995007,3.19196918412254));
#19152=CARTESIAN_POINT('Ctrl Pts',(-2.23909845280547,-0.552060840994624,
3.12505646843295));
#19153=CARTESIAN_POINT('Ctrl Pts',(-2.23909845280547,1.61522066995007,3.12505646843295));
#19154=CARTESIAN_POINT('Ctrl Pts',(-2.38189256086493,-0.552060840994624,
3.03403241435609));
#19155=CARTESIAN_POINT('Ctrl Pts',(-2.38189256086493,1.61522066995007,3.03403241435609));
#19156=CARTESIAN_POINT('Ctrl Pts',(-2.49960870420481,-0.552060840994624,
2.91510580081997));
#19157=CARTESIAN_POINT('Ctrl Pts',(-2.49960870420481,1.61522066995007,2.91510580081997));
#19158=CARTESIAN_POINT('Ctrl Pts',(-2.59397540849182,-0.552060840994624,
2.76722839711793));
#19159=CARTESIAN_POINT('Ctrl Pts',(-2.59397540849182,1.61522066995007,2.76722839711793));
#19160=CARTESIAN_POINT('Ctrl Pts',(-2.66797634363209,-0.552060840994624,
2.59347738935767));
#19161=CARTESIAN_POINT('Ctrl Pts',(-2.66797634363209,1.61522066995007,2.59347738935767));
#19162=CARTESIAN_POINT('Ctrl Pts',(-2.72531955636566,-0.552060840994624,
2.39962532458057));
#19163=CARTESIAN_POINT('Ctrl Pts',(-2.72531955636566,1.61522066995007,2.39962532458057));
#19164=CARTESIAN_POINT('Ctrl Pts',(-2.76985908233936,-0.552060840994624,
2.19251877196088));
#19165=CARTESIAN_POINT('Ctrl Pts',(-2.76985908233936,1.61522066995007,2.19251877196088));
#19166=CARTESIAN_POINT('Ctrl Pts',(-2.80505146480344,-0.552060840994624,
1.97856787413951));
#19167=CARTESIAN_POINT('Ctrl Pts',(-2.80505146480344,1.61522066995007,1.97856787413951));
#19168=CARTESIAN_POINT('Ctrl Pts',(-2.8333568624899,-0.552060840994624,
1.76209503442131));
#19169=CARTESIAN_POINT('Ctrl Pts',(-2.8333568624899,1.61522066995007,1.76209503442131));
#19170=CARTESIAN_POINT('Ctrl Pts',(-2.85578261679294,-0.552060840994624,
1.54401727992238));
#19171=CARTESIAN_POINT('Ctrl Pts',(-2.85578261679294,1.61522066995007,1.54401727992238));
#19172=CARTESIAN_POINT('Ctrl Pts',(-2.87284562964987,-0.552060840994624,
1.32371934078708));
#19173=CARTESIAN_POINT('Ctrl Pts',(-2.87284562964987,1.61522066995007,1.32371934078708));
#19174=CARTESIAN_POINT('Ctrl Pts',(-2.88537704766869,-0.552060840994624,
1.10060381648384));
#19175=CARTESIAN_POINT('Ctrl Pts',(-2.88537704766869,1.61522066995007,1.10060381648384));
#19176=CARTESIAN_POINT('Ctrl Pts',(-2.89547076625573,-0.552060840994624,
0.875890304828914));
#19177=CARTESIAN_POINT('Ctrl Pts',(-2.89547076625573,1.61522066995007,0.875890304828914));
#19178=CARTESIAN_POINT('Ctrl Pts',(-2.90717911786707,-0.552060840994624,
0.654020230869684));
#19179=CARTESIAN_POINT('Ctrl Pts',(-2.90717911786707,1.61522066995007,0.654020230869684));
#19180=CARTESIAN_POINT('Ctrl Pts',(-2.92780415844476,-0.552060840994624,
0.444963858672577));
#19181=CARTESIAN_POINT('Ctrl Pts',(-2.92780415844476,1.61522066995007,0.444963858672577));
#19182=CARTESIAN_POINT('Ctrl Pts',(-2.96639254265869,-0.552060840994624,
0.262319630540737));
#19183=CARTESIAN_POINT('Ctrl Pts',(-2.96639254265869,1.61522066995007,0.262319630540737));
#19184=CARTESIAN_POINT('Ctrl Pts',(-3.03063129752067,-0.552060840994624,
0.11901737132707));
#19185=CARTESIAN_POINT('Ctrl Pts',(-3.03063129752067,1.61522066995007,0.11901737132707));
#19186=CARTESIAN_POINT('Ctrl Pts',(-3.12452733970658,-0.552060840994624,
0.0241851999813871));
#19187=CARTESIAN_POINT('Ctrl Pts',(-3.12452733970658,1.61522066995007,0.0241851999813871));
#19188=CARTESIAN_POINT('Ctrl Pts',(-3.24511001026157,-0.552060840994624,
-0.0214179570895714));
#19189=CARTESIAN_POINT('Ctrl Pts',(-3.24511001026157,1.61522066995007,-0.0214179570895714));
#19190=CARTESIAN_POINT('Ctrl Pts',(-3.38164698943802,-0.552060840994624,
-0.0263068037112043));
#19191=CARTESIAN_POINT('Ctrl Pts',(-3.38164698943802,1.61522066995007,-0.0263068037112043));
#19192=CARTESIAN_POINT('Ctrl Pts',(-3.52045328348989,-0.552060840994624,
-0.00118366394785932));
#19193=CARTESIAN_POINT('Ctrl Pts',(-3.52045328348989,1.61522066995007,-0.00118366394785932));
#19194=CARTESIAN_POINT('Ctrl Pts',(-3.64881642260079,-0.552060840994624,
0.0470540298718583));
#19195=CARTESIAN_POINT('Ctrl Pts',(-3.64881642260079,1.61522066995007,0.0470540298718583));
#19196=CARTESIAN_POINT('Ctrl Pts',(-3.75872318140663,-0.552060840994624,
0.120497232333251));
#19197=CARTESIAN_POINT('Ctrl Pts',(-3.75872318140663,1.61522066995007,0.120497232333251));
#19198=CARTESIAN_POINT('Ctrl Pts',(-3.84598208672296,-0.552060840994624,
0.224659532804408));
#19199=CARTESIAN_POINT('Ctrl Pts',(-3.84598208672296,1.61522066995007,0.224659532804408));
#19200=CARTESIAN_POINT('Ctrl Pts',(-3.9098657241983,-0.552060840994624,
0.364350357241515));
#19201=CARTESIAN_POINT('Ctrl Pts',(-3.9098657241983,1.61522066995007,0.364350357241515));
#19202=CARTESIAN_POINT('Ctrl Pts',(-3.9525920016999,-0.552060840994624,
0.538436816836325));
#19203=CARTESIAN_POINT('Ctrl Pts',(-3.9525920016999,1.61522066995007,0.538436816836325));
#19204=CARTESIAN_POINT('Ctrl Pts',(-3.97841403016126,-0.552060840994624,
0.741129277895169));
#19205=CARTESIAN_POINT('Ctrl Pts',(-3.97841403016126,1.61522066995007,0.741129277895169));
#19206=CARTESIAN_POINT('Ctrl Pts',(-3.99260375067011,-0.552060840994624,
0.964078729991154));
#19207=CARTESIAN_POINT('Ctrl Pts',(-3.99260375067011,1.61522066995007,0.964078729991154));
#19208=CARTESIAN_POINT('Ctrl Pts',(-4.00047520099045,-0.552060840994624,
1.1981954227983));
#19209=CARTESIAN_POINT('Ctrl Pts',(-4.00047520099045,1.61522066995007,1.1981954227983));
#19210=CARTESIAN_POINT('Ctrl Pts',(-4.00639322616607,-0.552060840994624,
1.43558101932923));
#19211=CARTESIAN_POINT('Ctrl Pts',(-4.00639322616607,1.61522066995007,1.43558101932923));
#19212=CARTESIAN_POINT('Ctrl Pts',(-4.01278239926574,-0.552060840994624,
1.67142113207667));
#19213=CARTESIAN_POINT('Ctrl Pts',(-4.01278239926574,1.61522066995007,1.67142113207667));
#19214=CARTESIAN_POINT('Ctrl Pts',(-4.02066709528487,-0.552060840994624,
1.90332556813333));
#19215=CARTESIAN_POINT('Ctrl Pts',(-4.02066709528487,1.61522066995007,1.90332556813333));
#19216=CARTESIAN_POINT('Ctrl Pts',(-4.0302101444685,-0.552060840994624,
2.130657485557));
#19217=CARTESIAN_POINT('Ctrl Pts',(-4.0302101444685,1.61522066995007,2.130657485557));
#19218=CARTESIAN_POINT('Ctrl Pts',(-4.04126813644779,-0.552060840994624,
2.35385258470204));
#19219=CARTESIAN_POINT('Ctrl Pts',(-4.04126813644779,1.61522066995007,2.35385258470204));
#19220=CARTESIAN_POINT('Ctrl Pts',(-4.05390260344525,-0.552060840994624,
2.57377631141659));
#19221=CARTESIAN_POINT('Ctrl Pts',(-4.05390260344525,1.61522066995007,2.57377631141659));
#19222=CARTESIAN_POINT('Ctrl Pts',(-4.06899962712502,-0.552060840994624,
2.7909834104825));
#19223=CARTESIAN_POINT('Ctrl Pts',(-4.06899962712502,1.61522066995007,2.7909834104825));
#19224=CARTESIAN_POINT('Ctrl Pts',(-4.08854433447739,-0.552060840994624,
3.00529120729338));
#19225=CARTESIAN_POINT('Ctrl Pts',(-4.08854433447739,1.61522066995007,3.00529120729338));
#19226=CARTESIAN_POINT('Ctrl Pts',(-4.11518318246524,-0.552060840994624,
3.21600287470921));
#19227=CARTESIAN_POINT('Ctrl Pts',(-4.11518318246524,1.61522066995007,3.21600287470921));
#19228=CARTESIAN_POINT('Ctrl Pts',(-4.15193466045748,-0.552060840994624,
3.42199345348447));
#19229=CARTESIAN_POINT('Ctrl Pts',(-4.15193466045748,1.61522066995007,3.42199345348447));
#19230=CARTESIAN_POINT('Ctrl Pts',(-4.20184334854115,-0.552060840994624,
3.62185203209171));
#19231=CARTESIAN_POINT('Ctrl Pts',(-4.20184334854115,1.61522066995007,3.62185203209171));
#19232=CARTESIAN_POINT('Ctrl Pts',(-4.26765207024395,-0.552060840994624,
3.81399668859083));
#19233=CARTESIAN_POINT('Ctrl Pts',(-4.26765207024395,1.61522066995007,3.81399668859083));
#19234=CARTESIAN_POINT('Ctrl Pts',(-4.35148411330718,-0.552060840994624,
3.99681013615577));
#19235=CARTESIAN_POINT('Ctrl Pts',(-4.35148411330718,1.61522066995007,3.99681013615577));
#19236=CARTESIAN_POINT('Ctrl Pts',(-4.45474519640294,-0.552060840994624,
4.16885849319142));
#19237=CARTESIAN_POINT('Ctrl Pts',(-4.45474519640294,1.61522066995007,4.16885849319142));
#19238=CARTESIAN_POINT('Ctrl Pts',(-4.57800047823775,-0.552060840994624,
4.32911151507774));
#19239=CARTESIAN_POINT('Ctrl Pts',(-4.57800047823775,1.61522066995007,4.32911151507774));
#19240=CARTESIAN_POINT('Ctrl Pts',(-4.7208720035032,-0.552060840994624,
4.47714872481861));
#19241=CARTESIAN_POINT('Ctrl Pts',(-4.7208720035032,1.61522066995007,4.47714872481861));
#19242=CARTESIAN_POINT('Ctrl Pts',(-4.88190185104852,-0.552060840994624,
4.61340315498244));
#19243=CARTESIAN_POINT('Ctrl Pts',(-4.88190185104852,1.61522066995007,4.61340315498244));
#19244=CARTESIAN_POINT('Ctrl Pts',(-5.05850630701885,-0.552060840994624,
4.73929437247796));
#19245=CARTESIAN_POINT('Ctrl Pts',(-5.05850630701885,1.61522066995007,4.73929437247796));
#19246=CARTESIAN_POINT('Ctrl Pts',(-5.24741086000019,-0.552060840994624,
4.8567611153285));
#19247=CARTESIAN_POINT('Ctrl Pts',(-5.24741086000019,1.61522066995007,4.8567611153285));
#19248=CARTESIAN_POINT('Ctrl Pts',(-5.44501860313342,-0.552060840994624,
4.96787993373728));
#19249=CARTESIAN_POINT('Ctrl Pts',(-5.44501860313342,1.61522066995007,4.96787993373728));
#19250=CARTESIAN_POINT('Ctrl Pts',(-5.64781737380319,-0.552060840994624,
5.07442896098937));
#19251=CARTESIAN_POINT('Ctrl Pts',(-5.64781737380319,1.61522066995007,5.07442896098937));
#19252=CARTESIAN_POINT('Ctrl Pts',(-5.85274048349242,-0.552060840994624,
5.17752467829109));
#19253=CARTESIAN_POINT('Ctrl Pts',(-5.85274048349242,1.61522066995007,5.17752467829109));
#19254=CARTESIAN_POINT('Ctrl Pts',(-6.05762450882858,-0.552060840994624,
5.27709955371564));
#19255=CARTESIAN_POINT('Ctrl Pts',(-6.05762450882858,1.61522066995007,5.27709955371564));
#19256=CARTESIAN_POINT('Ctrl Pts',(-6.26112587698772,-0.552060840994624,
5.37226655127787));
#19257=CARTESIAN_POINT('Ctrl Pts',(-6.26112587698772,1.61522066995007,5.37226655127787));
#19258=CARTESIAN_POINT('Ctrl Pts',(-6.46246210121964,-0.552060840994624,
5.46195513100446));
#19259=CARTESIAN_POINT('Ctrl Pts',(-6.46246210121964,1.61522066995007,5.46195513100446));
#19260=CARTESIAN_POINT('Ctrl Pts',(-6.66121503090592,-0.552060840994624,
5.54547963906637));
#19261=CARTESIAN_POINT('Ctrl Pts',(-6.66121503090592,1.61522066995007,5.54547963906637));
#19262=CARTESIAN_POINT('Ctrl Pts',(-6.8570997603751,-0.552060840994624,
5.62308582598972));
#19263=CARTESIAN_POINT('Ctrl Pts',(-6.8570997603751,1.61522066995007,5.62308582598972));
#19264=CARTESIAN_POINT('Ctrl Pts',(-7.04976847947249,-0.552060840994624,
5.69662713609756));
#19265=CARTESIAN_POINT('Ctrl Pts',(-7.04976847947249,1.61522066995007,5.69662713609756));
#19266=CARTESIAN_POINT('Ctrl Pts',(-7.23853768475,-0.552060840994624,5.76979878895672));
#19267=CARTESIAN_POINT('Ctrl Pts',(-7.23853768475,1.61522066995007,5.76979878895672));
#19268=CARTESIAN_POINT('Ctrl Pts',(-7.42198551710617,-0.552060840994624,
5.84723737025949));
#19269=CARTESIAN_POINT('Ctrl Pts',(-7.42198551710617,1.61522066995007,5.84723737025949));
#19270=CARTESIAN_POINT('Ctrl Pts',(-7.59751903688412,-0.552060840994624,
5.93381436957244));
#19271=CARTESIAN_POINT('Ctrl Pts',(-7.59751903688412,1.61522066995007,5.93381436957244));
#19272=CARTESIAN_POINT('Ctrl Pts',(-7.76106756457753,-0.552060840994624,
6.03389995867283));
#19273=CARTESIAN_POINT('Ctrl Pts',(-7.76106756457753,1.61522066995007,6.03389995867283));
#19274=CARTESIAN_POINT('Ctrl Pts',(-7.90644860448901,-0.552060840994624,
6.15052660592937));
#19275=CARTESIAN_POINT('Ctrl Pts',(-7.90644860448901,1.61522066995007,6.15052660592937));
#19276=CARTESIAN_POINT('Ctrl Pts',(-8.02580908828117,-0.552060840994624,
6.28498018271686));
#19277=CARTESIAN_POINT('Ctrl Pts',(-8.02580908828117,1.61522066995007,6.28498018271686));
#19278=CARTESIAN_POINT('Ctrl Pts',(-8.11207116917861,-0.552060840994624,
6.43720976255636));
#19279=CARTESIAN_POINT('Ctrl Pts',(-8.11207116917861,1.61522066995007,6.43720976255636));
#19280=CARTESIAN_POINT('Ctrl Pts',(-8.16089752265956,-0.552060840994624,
6.60605451948903));
#19281=CARTESIAN_POINT('Ctrl Pts',(-8.16089752265956,1.61522066995007,6.60605451948903));
#19282=CARTESIAN_POINT('Ctrl Pts',(-8.17293082304181,-0.552060840994624,
6.78954489191904));
#19283=CARTESIAN_POINT('Ctrl Pts',(-8.17293082304181,1.61522066995007,6.78954489191904));
#19284=CARTESIAN_POINT('Ctrl Pts',(-8.15569042861244,-0.552060840994624,
6.9851692342788));
#19285=CARTESIAN_POINT('Ctrl Pts',(-8.15569042861244,1.61522066995007,6.9851692342788));
#19286=CARTESIAN_POINT('Ctrl Pts',(-8.12057943633387,-0.552060840994624,
7.19009032473164));
#19287=CARTESIAN_POINT('Ctrl Pts',(-8.12057943633387,1.61522066995007,7.19009032473164));
#19288=CARTESIAN_POINT('Ctrl Pts',(-8.08008348678073,-0.552060840994624,
7.40136016279791));
#19289=CARTESIAN_POINT('Ctrl Pts',(-8.08008348678073,1.61522066995007,7.40136016279791));
#19290=CARTESIAN_POINT('Ctrl Pts',(-8.04494633492831,-0.552060840994624,
7.61613341658677));
#19291=CARTESIAN_POINT('Ctrl Pts',(-8.04494633492831,1.61522066995007,7.61613341658677));
#19292=CARTESIAN_POINT('Ctrl Pts',(-8.02124364536279,-0.552060840994624,
7.83188673232793));
#19293=CARTESIAN_POINT('Ctrl Pts',(-8.02124364536279,1.61522066995007,7.83188673232793));
#19294=CARTESIAN_POINT('Ctrl Pts',(-8.007818938056,-0.552060840994624,8.04662057355248));
#19295=CARTESIAN_POINT('Ctrl Pts',(-8.007818938056,1.61522066995007,8.04662057355248));
#19296=CARTESIAN_POINT('Ctrl Pts',(-7.99879843919661,-0.552060840994624,
8.25883677791483));
#19297=CARTESIAN_POINT('Ctrl Pts',(-7.99879843919661,1.61522066995007,8.25883677791483));
#19298=CARTESIAN_POINT('Ctrl Pts',(-7.98575825096101,-0.552060840994624,
8.46752658699528));
#19299=CARTESIAN_POINT('Ctrl Pts',(-7.98575825096101,1.61522066995007,8.46752658699528));
#19300=CARTESIAN_POINT('Ctrl Pts',(-7.96007609558389,-0.552060840994624,
8.67216210283896));
#19301=CARTESIAN_POINT('Ctrl Pts',(-7.96007609558389,1.61522066995007,8.67216210283896));
#19302=CARTESIAN_POINT('Ctrl Pts',(-7.91508259073019,-0.552060840994624,
8.87266947141823));
#19303=CARTESIAN_POINT('Ctrl Pts',(-7.91508259073019,1.61522066995007,8.87266947141823));
#19304=CARTESIAN_POINT('Ctrl Pts',(-7.84862074946261,-0.552060840994624,
9.06945407016992));
#19305=CARTESIAN_POINT('Ctrl Pts',(-7.84862074946261,1.61522066995007,9.06945407016992));
#19306=CARTESIAN_POINT('Ctrl Pts',(-7.76209282457479,-0.552060840994624,
9.26297089919765));
#19307=CARTESIAN_POINT('Ctrl Pts',(-7.76209282457479,1.61522066995007,9.26297089919765));
#19308=CARTESIAN_POINT('Ctrl Pts',(-7.65900038660722,-0.552060840994624,
9.4532499945042));
#19309=CARTESIAN_POINT('Ctrl Pts',(-7.65900038660722,1.61522066995007,9.4532499945042));
#19310=CARTESIAN_POINT('Ctrl Pts',(-7.5436057352653,-0.552060840994624,
9.63939026966035));
#19311=CARTESIAN_POINT('Ctrl Pts',(-7.5436057352653,1.61522066995007,9.63939026966035));
#19312=CARTESIAN_POINT('Ctrl Pts',(-7.41967047355001,-0.552060840994624,
9.81917361987397));
#19313=CARTESIAN_POINT('Ctrl Pts',(-7.41967047355001,1.61522066995007,9.81917361987397));
#19314=CARTESIAN_POINT('Ctrl Pts',(-7.28883796912703,-0.552060840994624,
9.98835756998572));
#19315=CARTESIAN_POINT('Ctrl Pts',(-7.28883796912703,1.61522066995007,9.98835756998572));
#19316=CARTESIAN_POINT('Ctrl Pts',(-7.15081550722306,-0.552060840994624,
10.1414720974148));
#19317=CARTESIAN_POINT('Ctrl Pts',(-7.15081550722306,1.61522066995007,10.1414720974148));
#19318=CARTESIAN_POINT('Ctrl Pts',(-7.0044544864105,-0.552060840994624,
10.2733319413008));
#19319=CARTESIAN_POINT('Ctrl Pts',(-7.0044544864105,1.61522066995007,10.2733319413008));
#19320=CARTESIAN_POINT('Ctrl Pts',(-6.84859008776113,-0.552060840994624,
10.3804015453596));
#19321=CARTESIAN_POINT('Ctrl Pts',(-6.84859008776113,1.61522066995007,10.3804015453596));
#19322=CARTESIAN_POINT('Ctrl Pts',(-6.68288828293938,-0.552060840994624,
10.4620502678778));
#19323=CARTESIAN_POINT('Ctrl Pts',(-6.68288828293938,1.61522066995007,10.4620502678778));
#19324=CARTESIAN_POINT('Ctrl Pts',(-6.50892555577766,-0.552060840994624,
10.522290883026));
#19325=CARTESIAN_POINT('Ctrl Pts',(-6.50892555577766,1.61522066995007,10.522290883026));
#19326=CARTESIAN_POINT('Ctrl Pts',(-6.32976796473811,-0.552060840994624,
10.5687216653902));
#19327=CARTESIAN_POINT('Ctrl Pts',(-6.32976796473811,1.61522066995007,10.5687216653902));
#19328=CARTESIAN_POINT('Ctrl Pts',(-6.14893768388701,-0.552060840994624,
10.6103475969885));
#19329=CARTESIAN_POINT('Ctrl Pts',(-6.14893768388701,1.61522066995007,10.6103475969885));
#19330=CARTESIAN_POINT('Ctrl Pts',(-5.96961932707142,-0.552060840994624,
10.6558377434043));
#19331=CARTESIAN_POINT('Ctrl Pts',(-5.96961932707142,1.61522066995007,10.6558377434043));
#19332=CARTESIAN_POINT('Ctrl Pts',(-5.79367695415031,-0.552060840994624,
10.7114411549114));
#19333=CARTESIAN_POINT('Ctrl Pts',(-5.79367695415031,1.61522066995007,10.7114411549114));
#19334=CARTESIAN_POINT('Ctrl Pts',(-5.62101499943431,-0.552060840994624,
10.7795199127535));
#19335=CARTESIAN_POINT('Ctrl Pts',(-5.62101499943431,1.61522066995007,10.7795199127535));
#19336=CARTESIAN_POINT('Ctrl Pts',(-5.45051506148982,-0.552060840994624,
10.8599381259737));
#19337=CARTESIAN_POINT('Ctrl Pts',(-5.45051506148982,1.61522066995007,10.8599381259737));
#19338=CARTESIAN_POINT('Ctrl Pts',(-5.28082876351929,-0.552060840994624,
10.9511663773826));
#19339=CARTESIAN_POINT('Ctrl Pts',(-5.28082876351929,1.61522066995007,10.9511663773826));
#19340=CARTESIAN_POINT('Ctrl Pts',(-5.11112998264616,-0.552060840994624,
11.0513704191329));
#19341=CARTESIAN_POINT('Ctrl Pts',(-5.11112998264616,1.61522066995007,11.0513704191329));
#19342=CARTESIAN_POINT('Ctrl Pts',(-4.94211773226973,-0.552060840994624,
11.1598106424589));
#19343=CARTESIAN_POINT('Ctrl Pts',(-4.94211773226973,1.61522066995007,11.1598106424589));
#19344=CARTESIAN_POINT('Ctrl Pts',(-4.77596612414951,-0.552060840994624,
11.2768795166235));
#19345=CARTESIAN_POINT('Ctrl Pts',(-4.77596612414951,1.61522066995007,11.2768795166235));
#19346=CARTESIAN_POINT('Ctrl Pts',(-4.61532593596946,-0.552060840994624,
11.4029224160731));
#19347=CARTESIAN_POINT('Ctrl Pts',(-4.61532593596946,1.61522066995007,11.4029224160731));
#19348=CARTESIAN_POINT('Ctrl Pts',(-4.46255574628757,-0.552060840994624,
11.5373242211527));
#19349=CARTESIAN_POINT('Ctrl Pts',(-4.46255574628757,1.61522066995007,11.5373242211527));
#19350=CARTESIAN_POINT('Ctrl Pts',(-4.31893584999241,-0.552060840994624,
11.6776492463597));
#19351=CARTESIAN_POINT('Ctrl Pts',(-4.31893584999241,1.61522066995007,11.6776492463597));
#19352=CARTESIAN_POINT('Ctrl Pts',(-4.18369962429796,-0.552060840994624,
11.8183570873721));
#19353=CARTESIAN_POINT('Ctrl Pts',(-4.18369962429796,1.61522066995007,11.8183570873721));
#19354=CARTESIAN_POINT('Ctrl Pts',(-4.05395481372655,-0.552060840994624,
11.9514202619522));
#19355=CARTESIAN_POINT('Ctrl Pts',(-4.05395481372655,1.61522066995007,11.9514202619522));
#19356=CARTESIAN_POINT('Ctrl Pts',(-3.92533033057354,-0.552060840994624,
12.0684942936867));
#19357=CARTESIAN_POINT('Ctrl Pts',(-3.92533033057354,1.61522066995007,12.0684942936867));
#19358=CARTESIAN_POINT('Ctrl Pts',(-3.79241297762166,-0.552060840994624,
12.1626050652586));
#19359=CARTESIAN_POINT('Ctrl Pts',(-3.79241297762166,1.61522066995007,12.1626050652586));
#19360=CARTESIAN_POINT('Ctrl Pts',(-3.64927048315908,-0.552060840994624,
12.2301117722809));
#19361=CARTESIAN_POINT('Ctrl Pts',(-3.64927048315908,1.61522066995007,12.2301117722809));
#19362=CARTESIAN_POINT('Ctrl Pts',(-3.48993681214334,-0.552060840994624,
12.2723364229645));
#19363=CARTESIAN_POINT('Ctrl Pts',(-3.48993681214334,1.61522066995007,12.2723364229645));
#19364=CARTESIAN_POINT('Ctrl Pts',(-3.30884480305534,-0.552060840994624,
12.2938762651139));
#19365=CARTESIAN_POINT('Ctrl Pts',(-3.30884480305534,1.61522066995007,12.2938762651139));
#19366=CARTESIAN_POINT('Ctrl Pts',(-3.10127560868576,-0.552060840994624,
12.3010487961981));
#19367=CARTESIAN_POINT('Ctrl Pts',(-3.10127560868576,1.61522066995007,12.3010487961981));
#19368=CARTESIAN_POINT('Ctrl Pts',(-2.86376302967345,-0.552060840994624,
12.300400839059));
#19369=CARTESIAN_POINT('Ctrl Pts',(-2.86376302967345,1.61522066995007,12.300400839059));
#19370=CARTESIAN_POINT('Ctrl Pts',(-2.59461297443094,-0.552060840994624,
12.2969132923574));
#19371=CARTESIAN_POINT('Ctrl Pts',(-2.59461297443094,1.61522066995007,12.2969132923574));
#19372=CARTESIAN_POINT('Ctrl Pts',(-2.29394197380209,-0.552060840994624,
12.2935845551224));
#19373=CARTESIAN_POINT('Ctrl Pts',(-2.29394197380209,1.61522066995007,12.2935845551224));
#19374=CARTESIAN_POINT('Ctrl Pts',(-1.96338745719135,-0.552060840994624,
12.2919684497906));
#19375=CARTESIAN_POINT('Ctrl Pts',(-1.96338745719135,1.61522066995007,12.2919684497906));
#19376=CARTESIAN_POINT('Ctrl Pts',(-1.60591558979456,-0.552060840994624,
12.2924280531798));
#19377=CARTESIAN_POINT('Ctrl Pts',(-1.60591558979456,1.61522066995007,12.2924280531798));
#19378=CARTESIAN_POINT('Ctrl Pts',(-1.22558901314075,-0.552060840994624,
12.2945066442122));
#19379=CARTESIAN_POINT('Ctrl Pts',(-1.22558901314075,1.61522066995007,12.2945066442122));
#19380=CARTESIAN_POINT('Ctrl Pts',(-0.827351903312651,-0.552060840994624,
12.2972483292773));
#19381=CARTESIAN_POINT('Ctrl Pts',(-0.827351903312651,1.61522066995007,
12.2972483292773));
#19382=CARTESIAN_POINT('Ctrl Pts',(-0.498916532526571,-0.552060840994624,
12.299081889758));
#19383=CARTESIAN_POINT('Ctrl Pts',(-0.498916532526571,1.61522066995007,
12.299081889758));
#19384=CARTESIAN_POINT('Ctrl Pts',(-0.249771440080693,-0.552060840994624,
12.2998330708668));
#19385=CARTESIAN_POINT('Ctrl Pts',(-0.249771440080693,1.61522066995007,
12.2998330708668));
#19386=CARTESIAN_POINT('Ctrl Pts',(-0.0832571466935557,-0.552060840994624,
12.2999999999989));
#19387=CARTESIAN_POINT('Ctrl Pts',(-0.0832571466935557,1.61522066995007,
12.2999999999989));
#19388=CARTESIAN_POINT('Ctrl Pts',(0.,-0.552060840994624,12.3));
#19389=CARTESIAN_POINT('Ctrl Pts',(0.,1.61522066995007,12.3));
#19390=CARTESIAN_POINT('Ctrl Pts',(0.0832571466935396,-0.552060840994624,
12.3000000000011));
#19391=CARTESIAN_POINT('Ctrl Pts',(0.0832571466935396,1.61522066995007,
12.3000000000011));
#19392=CARTESIAN_POINT('Ctrl Pts',(0.24977144008061,-0.552060840994624,
12.2998330708736));
#19393=CARTESIAN_POINT('Ctrl Pts',(0.24977144008061,1.61522066995007,12.2998330708736));
#19394=CARTESIAN_POINT('Ctrl Pts',(0.498916532526534,-0.552060840994624,
12.2990818897713));
#19395=CARTESIAN_POINT('Ctrl Pts',(0.498916532526534,1.61522066995007,12.2990818897713));
#19396=CARTESIAN_POINT('Ctrl Pts',(0.827351903312438,-0.552060840994624,
12.2972483292974));
#19397=CARTESIAN_POINT('Ctrl Pts',(0.827351903312438,1.61522066995007,12.2972483292974));
#19398=CARTESIAN_POINT('Ctrl Pts',(1.22558901314046,-0.552060840994624,
12.2945066442369));
#19399=CARTESIAN_POINT('Ctrl Pts',(1.22558901314046,1.61522066995007,12.2945066442369));
#19400=CARTESIAN_POINT('Ctrl Pts',(1.60591558979418,-0.552060840994624,
12.2924280532047));
#19401=CARTESIAN_POINT('Ctrl Pts',(1.60591558979418,1.61522066995007,12.2924280532047));
#19402=CARTESIAN_POINT('Ctrl Pts',(1.96338745719096,-0.552060840994624,
12.291968449812));
#19403=CARTESIAN_POINT('Ctrl Pts',(1.96338745719096,1.61522066995007,12.291968449812));
#19404=CARTESIAN_POINT('Ctrl Pts',(2.29394197380175,-0.552060840994624,
12.2935845551378));
#19405=CARTESIAN_POINT('Ctrl Pts',(2.29394197380175,1.61522066995007,12.2935845551378));
#19406=CARTESIAN_POINT('Ctrl Pts',(2.59461297443069,-0.552060840994624,
12.2969132923658));
#19407=CARTESIAN_POINT('Ctrl Pts',(2.59461297443069,1.61522066995007,12.2969132923658));
#19408=CARTESIAN_POINT('Ctrl Pts',(2.86376302967335,-0.552060840994624,
12.3004008390612));
#19409=CARTESIAN_POINT('Ctrl Pts',(2.86376302967335,1.61522066995007,12.3004008390612));
#19410=CARTESIAN_POINT('Ctrl Pts',(3.10127560868576,-0.552060840994624,
12.3010487961961));
#19411=CARTESIAN_POINT('Ctrl Pts',(3.10127560868576,1.61522066995007,12.3010487961961));
#19412=CARTESIAN_POINT('Ctrl Pts',(3.30884480305537,-0.552060840994624,
12.2938762651102));
#19413=CARTESIAN_POINT('Ctrl Pts',(3.30884480305537,1.61522066995007,12.2938762651102));
#19414=CARTESIAN_POINT('Ctrl Pts',(3.48993681214337,-0.552060840994624,
12.2723364229612));
#19415=CARTESIAN_POINT('Ctrl Pts',(3.48993681214337,1.61522066995007,12.2723364229612));
#19416=CARTESIAN_POINT('Ctrl Pts',(3.64927048315907,-0.552060840994624,
12.2301117722792));
#19417=CARTESIAN_POINT('Ctrl Pts',(3.64927048315907,1.61522066995007,12.2301117722792));
#19418=CARTESIAN_POINT('Ctrl Pts',(3.79241297762162,-0.552060840994624,
12.1626050652587));
#19419=CARTESIAN_POINT('Ctrl Pts',(3.79241297762162,1.61522066995007,12.1626050652587));
#19420=CARTESIAN_POINT('Ctrl Pts',(3.90529123941674,-0.552060840994624,
12.0826827671148));
#19421=CARTESIAN_POINT('Ctrl Pts',(3.90529123941674,1.61522066995007,12.0826827671148));
#19422=CARTESIAN_POINT('Ctrl Pts',(3.98932418204563,-0.552060840994624,
12.0094836266392));
#19423=CARTESIAN_POINT('Ctrl Pts',(3.98932418204563,1.61522066995007,12.0094836266392));
#19424=CARTESIAN_POINT('Ctrl Pts',(4.04740991713241,-0.552060840994624,
11.9543581845679));
#19425=CARTESIAN_POINT('Ctrl Pts',(4.04740991713241,1.61522066995007,11.9543581845679));
#19426=CARTESIAN_POINT('Ctrl Pts',(4.07977092452996,-0.552060840994624,
11.9226494651812));
#19427=CARTESIAN_POINT('Ctrl Pts',(4.07977092452996,1.61522066995007,11.9226494651812));
#19428=CARTESIAN_POINT('Ctrl Pts',(4.08617023400024,-0.552060840994624,
11.9163435012344));
#19429=CARTESIAN_POINT('Ctrl Pts',(4.08617023400024,1.61522066995007,11.9163435012344));
#19430=CARTESIAN_POINT('Ctrl Pts',(4.32736007730607,0.051480639880881,11.6713697523917));
#19431=CARTESIAN_POINT('Ctrl Pts',(4.32922017460619,0.0445386622515201,
11.6695096731142));
#19432=CARTESIAN_POINT('Ctrl Pts',(4.33107905956623,0.0376012091336625,
11.6676530278345));
#19433=CARTESIAN_POINT('Ctrl Pts',(4.33293714059226,0.0306667563398385,
11.6657994729934));
#19434=CARTESIAN_POINT('Ctrl Pts',(4.3617605754817,-0.0769037671161592,
11.9026515720695));
#19435=CARTESIAN_POINT('Ctrl Pts',(4.11947753888128,0.827308835288644,11.9026515720695));
#19436=CARTESIAN_POINT('Ctrl Pts',(4.37804997056012,-0.0725390368597044,
11.8858809149492));
#19437=CARTESIAN_POINT('Ctrl Pts',(4.1357669339597,0.831673565545099,11.8858809149492));
#19438=CARTESIAN_POINT('Ctrl Pts',(4.41963045011986,-0.0613975809407722,
11.842517268502));
#19439=CARTESIAN_POINT('Ctrl Pts',(4.17734741351944,0.842815021464031,11.842517268502));
#19440=CARTESIAN_POINT('Ctrl Pts',(4.48720217786378,-0.0432917910606122,
11.7703786717735));
#19441=CARTESIAN_POINT('Ctrl Pts',(4.24491914126336,0.860920811344191,11.7703786717735));
#19442=CARTESIAN_POINT('Ctrl Pts',(4.58301627616637,-0.0176184807969185,
11.667756621275));
#19443=CARTESIAN_POINT('Ctrl Pts',(4.34073323956595,0.886594121607884,11.667756621275));
#19444=CARTESIAN_POINT('Ctrl Pts',(4.71196253429032,0.0169325649344106,
11.5373242211525));
#19445=CARTESIAN_POINT('Ctrl Pts',(4.4696794976899,0.921145167339214,11.5373242211525));
#19446=CARTESIAN_POINT('Ctrl Pts',(4.85952720599112,0.056472399548002,11.4029224160728));
#19447=CARTESIAN_POINT('Ctrl Pts',(4.6172441693907,0.960685001952805,11.4029224160728));
#19448=CARTESIAN_POINT('Ctrl Pts',(5.01469371249416,0.0980491396578512,
11.2768795166233));
#19449=CARTESIAN_POINT('Ctrl Pts',(4.77241067589374,1.00226174206265,11.2768795166233));
#19450=CARTESIAN_POINT('Ctrl Pts',(5.17518384185696,0.141052340213779,11.1598106424589));
#19451=CARTESIAN_POINT('Ctrl Pts',(4.93290080525654,1.04526494261858,11.1598106424589));
#19452=CARTESIAN_POINT('Ctrl Pts',(5.33843713945481,0.18479592946684,11.051370419133));
#19453=CARTESIAN_POINT('Ctrl Pts',(5.09615410285439,1.08900853187164,11.051370419133));
#19454=CARTESIAN_POINT('Ctrl Pts',(5.50235357458993,0.228717205887484,10.9511663773825));
#19455=CARTESIAN_POINT('Ctrl Pts',(5.26007053798951,1.13292980829229,10.9511663773825));
#19456=CARTESIAN_POINT('Ctrl Pts',(5.66625795216703,0.272635251495195,10.8599381259735));
#19457=CARTESIAN_POINT('Ctrl Pts',(5.42397491556661,1.1768478539,10.8599381259735));
#19458=CARTESIAN_POINT('Ctrl Pts',(5.83094824560827,0.31676388262402,10.7795199127532));
#19459=CARTESIAN_POINT('Ctrl Pts',(5.58866520900785,1.22097648502882,10.7795199127532));
#19460=CARTESIAN_POINT('Ctrl Pts',(5.99772688688598,0.361452084869143,10.7114411549111));
#19461=CARTESIAN_POINT('Ctrl Pts',(5.75544385028556,1.26566468727395,10.7114411549111));
#19462=CARTESIAN_POINT('Ctrl Pts',(6.16767416882911,0.406989321821667,10.6558377434042));
#19463=CARTESIAN_POINT('Ctrl Pts',(5.92539113222869,1.31120192422647,10.6558377434042));
#19464=CARTESIAN_POINT('Ctrl Pts',(6.3408824008051,0.453400327702056,10.6103475969888));
#19465=CARTESIAN_POINT('Ctrl Pts',(6.09859936420468,1.35761293010686,10.6103475969888));
#19466=CARTESIAN_POINT('Ctrl Pts',(6.51555103925432,0.50020264831757,10.5687216653907));
#19467=CARTESIAN_POINT('Ctrl Pts',(6.2732680026539,1.40441525072237,10.5687216653907));
#19468=CARTESIAN_POINT('Ctrl Pts',(6.68860398341517,0.546572044953298,10.5222908830264));
#19469=CARTESIAN_POINT('Ctrl Pts',(6.44632094681475,1.4507846473581,10.5222908830264));
#19470=CARTESIAN_POINT('Ctrl Pts',(6.8566390743923,0.591596911880709,10.462050267878));
#19471=CARTESIAN_POINT('Ctrl Pts',(6.61435603779188,1.49580951428551,10.462050267878));
#19472=CARTESIAN_POINT('Ctrl Pts',(7.01669472713225,0.634483694776415,10.3804015453596));
#19473=CARTESIAN_POINT('Ctrl Pts',(6.77441169053183,1.53869629718122,10.3804015453596));
#19474=CARTESIAN_POINT('Ctrl Pts',(7.16724817518663,0.674824369600307,10.2733319413005));
#19475=CARTESIAN_POINT('Ctrl Pts',(6.92496513858621,1.57903697200511,10.2733319413005));
#19476=CARTESIAN_POINT('Ctrl Pts',(7.30862206515146,0.71270538924723,10.1414720974144));
#19477=CARTESIAN_POINT('Ctrl Pts',(7.06633902855104,1.61691799165203,10.1414720974144));
#19478=CARTESIAN_POINT('Ctrl Pts',(7.44194152571249,0.748428231039911,9.98835756998534));
#19479=CARTESIAN_POINT('Ctrl Pts',(7.19965848911207,1.65264083344471,9.98835756998534));
#19480=CARTESIAN_POINT('Ctrl Pts',(7.56831602065279,0.782290174903054,9.81917361987377));
#19481=CARTESIAN_POINT('Ctrl Pts',(7.32603298405237,1.68650277730786,9.81917361987377));
#19482=CARTESIAN_POINT('Ctrl Pts',(7.68802829073163,0.814366980994775,9.63939026966049));
#19483=CARTESIAN_POINT('Ctrl Pts',(7.44574525413121,1.71857958339958,9.63939026966049));
#19484=CARTESIAN_POINT('Ctrl Pts',(7.79949096467857,0.844233314465072,9.45324999450471));
#19485=CARTESIAN_POINT('Ctrl Pts',(7.55720792807815,1.74844591686987,9.45324999450471));
#19486=CARTESIAN_POINT('Ctrl Pts',(7.89907061300659,0.87091560081714,9.26297089919836));
#19487=CARTESIAN_POINT('Ctrl Pts',(7.65678757640617,1.77512820322194,9.26297089919836));
#19488=CARTESIAN_POINT('Ctrl Pts',(7.98265017035093,0.893310675711308,9.06945407017055));
#19489=CARTESIAN_POINT('Ctrl Pts',(7.74036713375051,1.79752327811611,9.06945407017055));
#19490=CARTESIAN_POINT('Ctrl Pts',(8.04684737929391,0.910512266003911,8.87266947141857));
#19491=CARTESIAN_POINT('Ctrl Pts',(7.80456434269349,1.81472486840871,8.87266947141857));
#19492=CARTESIAN_POINT('Ctrl Pts',(8.09030776764722,0.922157441965925,8.67216210283894));
#19493=CARTESIAN_POINT('Ctrl Pts',(7.8480247310468,1.82637004437073,8.67216210283894));
#19494=CARTESIAN_POINT('Ctrl Pts',(8.11511482480059,0.928804472896761,8.46752658699496));
#19495=CARTESIAN_POINT('Ctrl Pts',(7.87283178820017,1.83301707530156,8.46752658699496));
#19496=CARTESIAN_POINT('Ctrl Pts',(8.12771067939691,0.932179521963826,8.25883677791438));
#19497=CARTESIAN_POINT('Ctrl Pts',(7.88542764279649,1.83639212436863,8.25883677791438));
#19498=CARTESIAN_POINT('Ctrl Pts',(8.1364238122112,0.93451419886496,8.04662057355209));
#19499=CARTESIAN_POINT('Ctrl Pts',(7.89414077561078,1.83872680126976,8.04662057355209));
#19500=CARTESIAN_POINT('Ctrl Pts',(8.1493910837093,0.937988768790909,7.8318867323277));
#19501=CARTESIAN_POINT('Ctrl Pts',(7.90710804710888,1.84220137119571,7.8318867323277));
#19502=CARTESIAN_POINT('Ctrl Pts',(8.17228612371332,0.944123476270666,7.61613341658679));
#19503=CARTESIAN_POINT('Ctrl Pts',(7.9300030871129,1.84833607867547,7.61613341658679));
#19504=CARTESIAN_POINT('Ctrl Pts',(8.20622600615005,0.953217640360794,7.40136016279815));
#19505=CARTESIAN_POINT('Ctrl Pts',(7.96394296954963,1.8574302427656,7.40136016279815));
#19506=CARTESIAN_POINT('Ctrl Pts',(8.2453420896837,0.963698763354704,7.19009032473197));
#19507=CARTESIAN_POINT('Ctrl Pts',(8.00305905308328,1.86791136575951,7.19009032473197));
#19508=CARTESIAN_POINT('Ctrl Pts',(8.27925670391221,0.972786156848846,6.98516923427904));
#19509=CARTESIAN_POINT('Ctrl Pts',(8.03697366731179,1.87699875925365,6.98516923427904));
#19510=CARTESIAN_POINT('Ctrl Pts',(8.2959096461468,0.977248299272207,6.78954489191915));
#19511=CARTESIAN_POINT('Ctrl Pts',(8.05362660954638,1.88146090167701,6.78954489191915));
#19512=CARTESIAN_POINT('Ctrl Pts',(8.28428637053186,0.974133851957781,6.60605451948904));
#19513=CARTESIAN_POINT('Ctrl Pts',(8.04200333393144,1.87834645436258,6.60605451948904));
#19514=CARTESIAN_POINT('Ctrl Pts',(8.23712373470092,0.961496661773958,6.43720976255638));
#19515=CARTESIAN_POINT('Ctrl Pts',(7.9948406981005,1.86570926417876,6.43720976255638));
#19516=CARTESIAN_POINT('Ctrl Pts',(8.15380096293257,0.939170392367506,6.28498018271691));
#19517=CARTESIAN_POINT('Ctrl Pts',(7.91151792633215,1.84338299477231,6.28498018271691));
#19518=CARTESIAN_POINT('Ctrl Pts',(8.03850758899942,0.908277625929457,6.15052660592943));
#19519=CARTESIAN_POINT('Ctrl Pts',(7.796224552399,1.81249022833426,6.15052660592943));
#19520=CARTESIAN_POINT('Ctrl Pts',(7.89808028789632,0.870650244003599,6.03389995867286));
#19521=CARTESIAN_POINT('Ctrl Pts',(7.6557972512959,1.7748628464084,6.03389995867286));
#19522=CARTESIAN_POINT('Ctrl Pts',(7.74010454114588,0.828320770238116,5.93381436957244));
#19523=CARTESIAN_POINT('Ctrl Pts',(7.49782150454546,1.73253337264292,5.93381436957244));
#19524=CARTESIAN_POINT('Ctrl Pts',(7.57055218101304,0.78288935226573,5.84723737025948));
#19525=CARTESIAN_POINT('Ctrl Pts',(7.32826914441262,1.68710195467053,5.84723737025948));
#19526=CARTESIAN_POINT('Ctrl Pts',(7.39335518196344,0.735409559469172,5.76979878895671));
#19527=CARTESIAN_POINT('Ctrl Pts',(7.15107214536302,1.63962216187397,5.76979878895671));
#19528=CARTESIAN_POINT('Ctrl Pts',(7.21101813137776,0.686552494014464,5.69662713609756));
#19529=CARTESIAN_POINT('Ctrl Pts',(6.96873509477734,1.59076509641927,5.69662713609756));
#19530=CARTESIAN_POINT('Ctrl Pts',(7.02491443968342,0.636686160116518,5.62308582598972));
#19531=CARTESIAN_POINT('Ctrl Pts',(6.782631403083,1.54089876252132,5.62308582598972));
#19532=CARTESIAN_POINT('Ctrl Pts',(6.83570432051349,0.585987461485138,5.54547963906641));
#19533=CARTESIAN_POINT('Ctrl Pts',(6.59342128391307,1.49020006388994,5.54547963906641));
#19534=CARTESIAN_POINT('Ctrl Pts',(6.64372373267898,0.53454641801243,5.46195513100458));
#19535=CARTESIAN_POINT('Ctrl Pts',(6.40144069607856,1.43875902041723,5.46195513100458));
#19536=CARTESIAN_POINT('Ctrl Pts',(6.44924787392593,0.482436768712199,5.37226655127806));
#19537=CARTESIAN_POINT('Ctrl Pts',(6.20696483732551,1.386649371117,5.37226655127806));
#19538=CARTESIAN_POINT('Ctrl Pts',(6.25268064673585,0.429766738928191,5.27709955371581));
#19539=CARTESIAN_POINT('Ctrl Pts',(6.01039761013543,1.33397934133299,5.27709955371581));
#19540=CARTESIAN_POINT('Ctrl Pts',(6.05477787526952,0.376738851133908,5.17752467829117));
#19541=CARTESIAN_POINT('Ctrl Pts',(5.8124948386691,1.28095145353871,5.17752467829117));
#19542=CARTESIAN_POINT('Ctrl Pts',(5.85683735121713,0.323700847564676,5.07442896098936));
#19543=CARTESIAN_POINT('Ctrl Pts',(5.61455431461671,1.22791344996948,5.07442896098936));
#19544=CARTESIAN_POINT('Ctrl Pts',(5.66094878108745,0.271212663391943,4.96787993373722));
#19545=CARTESIAN_POINT('Ctrl Pts',(5.41866574448703,1.17542526579675,4.96787993373722));
#19546=CARTESIAN_POINT('Ctrl Pts',(5.47007435852032,0.220068016009324,4.85676111532844));
#19547=CARTESIAN_POINT('Ctrl Pts',(5.2277913219199,1.12428061841413,4.85676111532844));
#19548=CARTESIAN_POINT('Ctrl Pts',(5.28760657209206,0.171175919991177,4.73929437247794));
#19549=CARTESIAN_POINT('Ctrl Pts',(5.04532353549164,1.07538852239598,4.73929437247794));
#19550=CARTESIAN_POINT('Ctrl Pts',(5.11701976703263,0.125467323336097,4.61340315498245));
#19551=CARTESIAN_POINT('Ctrl Pts',(4.87473673043221,1.0296799257409,4.61340315498245));
#19552=CARTESIAN_POINT('Ctrl Pts',(4.96147687848527,0.0837897319614274,
4.47714872481864));
#19553=CARTESIAN_POINT('Ctrl Pts',(4.71919384188485,0.98800233436623,4.47714872481864));
#19554=CARTESIAN_POINT('Ctrl Pts',(4.82347358239015,0.0468118602199075,
4.32911151507775));
#19555=CARTESIAN_POINT('Ctrl Pts',(4.58119054578973,0.95102446262471,4.32911151507775));
#19556=CARTESIAN_POINT('Ctrl Pts',(4.70441812243944,0.0149110458715985,
4.16885849319143));
#19557=CARTESIAN_POINT('Ctrl Pts',(4.46213508583902,0.919123648276401,4.16885849319143));
#19558=CARTESIAN_POINT('Ctrl Pts',(4.60467557542669,-0.0118148890514923,
3.99681013615577));
#19559=CARTESIAN_POINT('Ctrl Pts',(4.36239253882627,0.892397713353311,3.99681013615577));
#19560=CARTESIAN_POINT('Ctrl Pts',(4.52370003996128,-0.0335122183861244,
3.81399668859083));
#19561=CARTESIAN_POINT('Ctrl Pts',(4.28141700336086,0.870700384018679,3.81399668859083));
#19562=CARTESIAN_POINT('Ctrl Pts',(4.46013369607337,-0.050544768896689,
3.62185203209172));
#19563=CARTESIAN_POINT('Ctrl Pts',(4.21785065947295,0.853667833508114,3.62185203209172));
#19564=CARTESIAN_POINT('Ctrl Pts',(4.41192560529702,-0.0634620878888593,
3.42199345348454));
#19565=CARTESIAN_POINT('Ctrl Pts',(4.1696425686966,0.840750514515944,3.42199345348454));
#19566=CARTESIAN_POINT('Ctrl Pts',(4.37642640354991,-0.0729740703289478,
3.21600287470933));
#19567=CARTESIAN_POINT('Ctrl Pts',(4.13414336694949,0.831238532075855,3.21600287470933));
#19568=CARTESIAN_POINT('Ctrl Pts',(4.35069525229582,-0.079868711527804,
3.00529120729351));
#19569=CARTESIAN_POINT('Ctrl Pts',(4.1084122156954,0.824343890876999,3.00529120729351));
#19570=CARTESIAN_POINT('Ctrl Pts',(4.33181651469696,-0.0849272540215386,
2.7909834104826));
#19571=CARTESIAN_POINT('Ctrl Pts',(4.08953347809654,0.819285348383264,2.7909834104826));
#19572=CARTESIAN_POINT('Ctrl Pts',(4.31723390962471,-0.0888346512741886,
2.57377631141663));
#19573=CARTESIAN_POINT('Ctrl Pts',(4.07495087302429,0.815377951130614,2.57377631141663));
#19574=CARTESIAN_POINT('Ctrl Pts',(4.30502995165065,-0.0921046919578018,
2.35385258470204));
#19575=CARTESIAN_POINT('Ctrl Pts',(4.06274691505023,0.812107910447001,2.35385258470204));
#19576=CARTESIAN_POINT('Ctrl Pts',(4.2943487516111,-0.0949667108825953,
2.13065748555701));
#19577=CARTESIAN_POINT('Ctrl Pts',(4.05206571501068,0.809245891522208,2.13065748555701));
#19578=CARTESIAN_POINT('Ctrl Pts',(4.28513087394313,-0.0974366337596561,
1.9033255681334));
#19579=CARTESIAN_POINT('Ctrl Pts',(4.04284783734271,0.806775968645147,1.9033255681334));
#19580=CARTESIAN_POINT('Ctrl Pts',(4.27751484242575,-0.0994773432542665,
1.67142113207676));
#19581=CARTESIAN_POINT('Ctrl Pts',(4.03523180582533,0.804735259150536,1.67142113207676));
#19582=CARTESIAN_POINT('Ctrl Pts',(4.27134337512002,-0.101130982934953,
1.4355810193293));
#19583=CARTESIAN_POINT('Ctrl Pts',(4.0290603385196,0.80308161946985,1.4355810193293));
#19584=CARTESIAN_POINT('Ctrl Pts',(4.26562700176213,-0.102662680559835,
1.19819542279832));
#19585=CARTESIAN_POINT('Ctrl Pts',(4.02334396516171,0.801549921844968,1.19819542279832));
#19586=CARTESIAN_POINT('Ctrl Pts',(4.25802376460729,-0.104699961815337,
0.964078729991153));
#19587=CARTESIAN_POINT('Ctrl Pts',(4.01574072800687,0.799512640589466,0.964078729991153));
#19588=CARTESIAN_POINT('Ctrl Pts',(4.24431754709998,-0.108372531727705,
0.741129277895168));
#19589=CARTESIAN_POINT('Ctrl Pts',(4.00203451049956,0.795840070677098,0.741129277895168));
#19590=CARTESIAN_POINT('Ctrl Pts',(4.21937538292203,-0.115055764476671,
0.538436816836329));
#19591=CARTESIAN_POINT('Ctrl Pts',(3.97709234632161,0.789156837928132,0.538436816836329));
#19592=CARTESIAN_POINT('Ctrl Pts',(4.17810496802208,-0.12611413882041,0.364350357241537));
#19593=CARTESIAN_POINT('Ctrl Pts',(3.93582193142166,0.778098463584393,0.364350357241537));
#19594=CARTESIAN_POINT('Ctrl Pts',(4.11639811270736,-0.142648440869452,
0.224659532804428));
#19595=CARTESIAN_POINT('Ctrl Pts',(3.87411507610694,0.761564161535351,0.224659532804428));
#19596=CARTESIAN_POINT('Ctrl Pts',(4.03211248248857,-0.165232707420125,
0.120497232333236));
#19597=CARTESIAN_POINT('Ctrl Pts',(3.78982944588815,0.738979894984678,0.120497232333236));
#19598=CARTESIAN_POINT('Ctrl Pts',(3.92595070567427,-0.193678669784572,
0.0470540298718229));
#19599=CARTESIAN_POINT('Ctrl Pts',(3.68366766907385,0.710533932620231,0.0470540298718229));
#19600=CARTESIAN_POINT('Ctrl Pts',(3.80196143446354,-0.22690149487561,-0.00118366394786523));
#19601=CARTESIAN_POINT('Ctrl Pts',(3.55967839786312,0.677311107529193,-0.00118366394786523));
#19602=CARTESIAN_POINT('Ctrl Pts',(3.66788485018745,-0.26282720735631,-0.0263068037111615));
#19603=CARTESIAN_POINT('Ctrl Pts',(3.42560181358703,0.641385395048493,-0.0263068037111615));
#19604=CARTESIAN_POINT('Ctrl Pts',(3.53600025575747,-0.29816557792793,-0.0214179570895094));
#19605=CARTESIAN_POINT('Ctrl Pts',(3.29371721915705,0.606047024476873,-0.0214179570895094));
#19606=CARTESIAN_POINT('Ctrl Pts',(3.41952634006544,-0.329374669576901,
0.0241851999814078));
#19607=CARTESIAN_POINT('Ctrl Pts',(3.17724330346502,0.574837932827902,0.0241851999814078));
#19608=CARTESIAN_POINT('Ctrl Pts',(3.32882972793161,-0.3536767535544,0.119017371327004));
#19609=CARTESIAN_POINT('Ctrl Pts',(3.08654669133119,0.550535848850403,0.119017371327004));
#19610=CARTESIAN_POINT('Ctrl Pts',(3.2667798555616,-0.370302966746397,0.262319630540593));
#19611=CARTESIAN_POINT('Ctrl Pts',(3.02449681896118,0.533909635658406,0.262319630540593));
#19612=CARTESIAN_POINT('Ctrl Pts',(3.22950633865455,-0.38029037550071,0.444963858672424));
#19613=CARTESIAN_POINT('Ctrl Pts',(2.98722330205413,0.523922226904093,0.444963858672424));
#19614=CARTESIAN_POINT('Ctrl Pts',(3.20958407929241,-0.385628528808198,
0.65402023086958));
#19615=CARTESIAN_POINT('Ctrl Pts',(2.96730104269199,0.518584073596605,0.65402023086958));
#19616=CARTESIAN_POINT('Ctrl Pts',(3.198274680088,-0.3886588731919,0.875890304828918));
#19617=CARTESIAN_POINT('Ctrl Pts',(2.95599164348758,0.515553729212903,0.875890304828918));
#19618=CARTESIAN_POINT('Ctrl Pts',(3.18852489662177,-0.391271319798056,
1.10060381648398));
#19619=CARTESIAN_POINT('Ctrl Pts',(2.94624186002135,0.512941282606747,1.10060381648398));
#19620=CARTESIAN_POINT('Ctrl Pts',(3.17642047631752,-0.394514689443426,
1.32371934078733));
#19621=CARTESIAN_POINT('Ctrl Pts',(2.9341374397171,0.509697912961377,1.32371934078733));
#19622=CARTESIAN_POINT('Ctrl Pts',(3.15993887152468,-0.398930922137636,
1.54401727992264));
#19623=CARTESIAN_POINT('Ctrl Pts',(2.91765583492426,0.505281680267167,1.54401727992264));
#19624=CARTESIAN_POINT('Ctrl Pts',(3.13827725626916,-0.404735134452108,
1.76209503442146));
#19625=CARTESIAN_POINT('Ctrl Pts',(2.89599421966874,0.499477467952695,1.76209503442146));
#19626=CARTESIAN_POINT('Ctrl Pts',(3.11093634162015,-0.412061110452637,
1.97856787413951));
#19627=CARTESIAN_POINT('Ctrl Pts',(2.86865330501973,0.492151491952166,1.97856787413951));
#19628=CARTESIAN_POINT('Ctrl Pts',(3.07694311050924,-0.421169569276931,
2.19251877196071));
#19629=CARTESIAN_POINT('Ctrl Pts',(2.83466007390882,0.483043033127872,2.19251877196071));
#19630=CARTESIAN_POINT('Ctrl Pts',(3.03392123208049,-0.432697246858785,
2.39962532458029));
#19631=CARTESIAN_POINT('Ctrl Pts',(2.79163819548007,0.471515355546018,2.39962532458029));
#19632=CARTESIAN_POINT('Ctrl Pts',(2.97853194193879,-0.447538762421585,
2.59347738935741));
#19633=CARTESIAN_POINT('Ctrl Pts',(2.73624890533837,0.456673839983218,2.59347738935741));
#19634=CARTESIAN_POINT('Ctrl Pts',(2.90705252751739,-0.466691613791248,
2.7672283971178));
#19635=CARTESIAN_POINT('Ctrl Pts',(2.66476949091697,0.437520988613555,2.7672283971178));
#19636=CARTESIAN_POINT('Ctrl Pts',(2.81590129070493,-0.491115514084246,
2.91510580081997));
#19637=CARTESIAN_POINT('Ctrl Pts',(2.57361825410451,0.413097088320557,2.91510580081997));
#19638=CARTESIAN_POINT('Ctrl Pts',(2.70219622768186,-0.521582693896607,
3.03403241435618));
#19639=CARTESIAN_POINT('Ctrl Pts',(2.45991319108144,0.382629908508196,3.03403241435618));
#19640=CARTESIAN_POINT('Ctrl Pts',(2.56426771086532,-0.558540528590822,
3.12505646843308));
#19641=CARTESIAN_POINT('Ctrl Pts',(2.3219846742649,0.345672073813981,3.12505646843308));
#19642=CARTESIAN_POINT('Ctrl Pts',(2.40152089622015,-0.602148406145732,
3.19196918412265));
#19643=CARTESIAN_POINT('Ctrl Pts',(2.15923785961973,0.302064196259071,3.19196918412265));
#19644=CARTESIAN_POINT('Ctrl Pts',(2.21432867499209,-0.652306410653179,
3.24001322621211));
#19645=CARTESIAN_POINT('Ctrl Pts',(1.97204563839167,0.251906191751624,3.24001322621211));
#19646=CARTESIAN_POINT('Ctrl Pts',(2.00391387642997,-0.708686886003457,
3.27464765209773));
#19647=CARTESIAN_POINT('Ctrl Pts',(1.76163083982955,0.195525716401346,3.27464765209773));
#19648=CARTESIAN_POINT('Ctrl Pts',(1.77223470132232,-0.770765133876661,
3.30006519349576));
#19649=CARTESIAN_POINT('Ctrl Pts',(1.5299516647219,0.133447468528142,3.30006519349576));
#19650=CARTESIAN_POINT('Ctrl Pts',(1.52187623321765,-0.837848483223599,
3.31897283641381));
#19651=CARTESIAN_POINT('Ctrl Pts',(1.27959319661723,0.066364119181204,3.31897283641381));
#19652=CARTESIAN_POINT('Ctrl Pts',(1.25594690908362,-0.909104030869067,
3.33300441174764));
#19653=CARTESIAN_POINT('Ctrl Pts',(1.0136638724832,-0.00489142846426405,
3.33300441174764));
#19654=CARTESIAN_POINT('Ctrl Pts',(0.977973383552497,-0.983586812552364,
3.34293392264922));
#19655=CARTESIAN_POINT('Ctrl Pts',(0.735690346952077,-0.0793742101475611,
3.34293392264922));
#19656=CARTESIAN_POINT('Ctrl Pts',(0.691796115956336,-1.0602677802969,3.34897162637417));
#19657=CARTESIAN_POINT('Ctrl Pts',(0.449513079355916,-0.156055177892097,
3.34897162637417));
#19658=CARTESIAN_POINT('Ctrl Pts',(0.401464687696532,-1.13806185203649,
3.35102435732185));
#19659=CARTESIAN_POINT('Ctrl Pts',(0.159181651096112,-0.233849249631687,
3.35102435732185));
#19660=CARTESIAN_POINT('Ctrl Pts',(0.111133259436734,-1.21585592377608,
3.34897162637426));
#19661=CARTESIAN_POINT('Ctrl Pts',(-0.131149777163686,-0.311643321371277,
3.34897162637426));
#19662=CARTESIAN_POINT('Ctrl Pts',(-0.175044008159397,-1.29253689152061,
3.34293392264938));
#19663=CARTESIAN_POINT('Ctrl Pts',(-0.417327044759817,-0.388324289115807,
3.34293392264938));
#19664=CARTESIAN_POINT('Ctrl Pts',(-0.453017533690513,-1.3670196732039,
3.33300441174785));
#19665=CARTESIAN_POINT('Ctrl Pts',(-0.695300570290933,-0.462807070799097,
3.33300441174785));
#19666=CARTESIAN_POINT('Ctrl Pts',(-0.718946857824558,-1.43827522084937,
3.31897283641402));
#19667=CARTESIAN_POINT('Ctrl Pts',(-0.961229894424978,-0.534062618444567,
3.31897283641402));
#19668=CARTESIAN_POINT('Ctrl Pts',(-0.969305325929253,-1.50535857019632,
3.30006519349591));
#19669=CARTESIAN_POINT('Ctrl Pts',(-1.21158836252967,-0.601145967791517,
3.30006519349591));
#19670=CARTESIAN_POINT('Ctrl Pts',(-1.20098450103692,-1.56743681806953,
3.27464765209779));
#19671=CARTESIAN_POINT('Ctrl Pts',(-1.44326753763734,-0.663224215664727,
3.27464765209779));
#19672=CARTESIAN_POINT('Ctrl Pts',(-1.41139929959904,-1.6238172934198,3.24001322621208));
#19673=CARTESIAN_POINT('Ctrl Pts',(-1.65368233619946,-0.719604691014997,
3.24001322621208));
#19674=CARTESIAN_POINT('Ctrl Pts',(-1.59859152082706,-1.67397529792724,
3.19196918412254));
#19675=CARTESIAN_POINT('Ctrl Pts',(-1.84087455742748,-0.769762695522437,
3.19196918412254));
#19676=CARTESIAN_POINT('Ctrl Pts',(-1.76133833547218,-1.71758317548214,
3.12505646843295));
#19677=CARTESIAN_POINT('Ctrl Pts',(-2.0036213720726,-0.813370573077337,
3.12505646843295));
#19678=CARTESIAN_POINT('Ctrl Pts',(-1.89926685228873,-1.75454101017635,
3.03403241435609));
#19679=CARTESIAN_POINT('Ctrl Pts',(-2.14154988888915,-0.850328407771547,
3.03403241435609));
#19680=CARTESIAN_POINT('Ctrl Pts',(-2.01297191531186,-1.78500818998873,
2.91510580081997));
#19681=CARTESIAN_POINT('Ctrl Pts',(-2.25525495191228,-0.880795587583927,
2.91510580081997));
#19682=CARTESIAN_POINT('Ctrl Pts',(-2.10412315212447,-1.80943209028177,
2.76722839711793));
#19683=CARTESIAN_POINT('Ctrl Pts',(-2.34640618872489,-0.905219487876967,
2.76722839711793));
#19684=CARTESIAN_POINT('Ctrl Pts',(-2.175602566546,-1.82858494165147,2.59347738935767));
#19685=CARTESIAN_POINT('Ctrl Pts',(-2.41788560314642,-0.924372339246667,
2.59347738935767));
#19686=CARTESIAN_POINT('Ctrl Pts',(-2.23099185668774,-1.84342645721428,
2.39962532458057));
#19687=CARTESIAN_POINT('Ctrl Pts',(-2.47327489328816,-0.939213854809477,
2.39962532458057));
#19688=CARTESIAN_POINT('Ctrl Pts',(-2.27401373511641,-1.85495413479611,
2.19251877196088));
#19689=CARTESIAN_POINT('Ctrl Pts',(-2.51629677171683,-0.950741532391307,
2.19251877196088));
#19690=CARTESIAN_POINT('Ctrl Pts',(-2.30800696622711,-1.86406259362035,
1.97856787413951));
#19691=CARTESIAN_POINT('Ctrl Pts',(-2.55029000282753,-0.959849991215547,
1.97856787413951));
#19692=CARTESIAN_POINT('Ctrl Pts',(-2.33534788087584,-1.8713885696208,1.76209503442131));
#19693=CARTESIAN_POINT('Ctrl Pts',(-2.57763091747626,-0.967175967215997,
1.76209503442131));
#19694=CARTESIAN_POINT('Ctrl Pts',(-2.35700949613116,-1.87719278193522,
1.54401727992238));
#19695=CARTESIAN_POINT('Ctrl Pts',(-2.59929253273158,-0.972980179530417,
1.54401727992238));
#19696=CARTESIAN_POINT('Ctrl Pts',(-2.37349110092397,-1.88160901462942,
1.32371934078708));
#19697=CARTESIAN_POINT('Ctrl Pts',(-2.61577413752439,-0.977396412224617,
1.32371934078708));
#19698=CARTESIAN_POINT('Ctrl Pts',(-2.38559552122837,-1.88485238427483,
1.10060381648384));
#19699=CARTESIAN_POINT('Ctrl Pts',(-2.62787855782879,-0.980639781870027,
1.10060381648384));
#19700=CARTESIAN_POINT('Ctrl Pts',(-2.39534530469489,-1.88746483088107,
0.875890304828914));
#19701=CARTESIAN_POINT('Ctrl Pts',(-2.63762834129531,-0.983252228476267,
0.875890304828914));
#19702=CARTESIAN_POINT('Ctrl Pts',(-2.40665470389955,-1.89049517526484,
0.654020230869684));
#19703=CARTESIAN_POINT('Ctrl Pts',(-2.64893774049997,-0.986282572860037,
0.654020230869684));
#19704=CARTESIAN_POINT('Ctrl Pts',(-2.42657696326181,-1.89583332857236,
0.444963858672577));
#19705=CARTESIAN_POINT('Ctrl Pts',(-2.66885999986223,-0.991620726167557,
0.444963858672577));
#19706=CARTESIAN_POINT('Ctrl Pts',(-2.46385048016881,-1.90582073732665,
0.262319630540737));
#19707=CARTESIAN_POINT('Ctrl Pts',(-2.70613351676923,-1.00160813492185,
0.262319630540737));
#19708=CARTESIAN_POINT('Ctrl Pts',(-2.52590035253865,-1.92244695051861,
0.11901737132707));
#19709=CARTESIAN_POINT('Ctrl Pts',(-2.76818338913907,-1.01823434811381,
0.11901737132707));
#19710=CARTESIAN_POINT('Ctrl Pts',(-2.61659696467234,-1.94674903449607,
0.0241851999813871));
#19711=CARTESIAN_POINT('Ctrl Pts',(-2.85888000127276,-1.04253643209127,
0.0241851999813871));
#19712=CARTESIAN_POINT('Ctrl Pts',(-2.73307088036432,-1.97795812614502,
-0.0214179570895714));
#19713=CARTESIAN_POINT('Ctrl Pts',(-2.97535391696474,-1.07374552374022,
-0.0214179570895714));
#19714=CARTESIAN_POINT('Ctrl Pts',(-2.86495547479434,-2.01329649671666,
-0.0263068037112043));
#19715=CARTESIAN_POINT('Ctrl Pts',(-3.10723851139476,-1.10908389431186,
-0.0263068037112043));
#19716=CARTESIAN_POINT('Ctrl Pts',(-2.99903205907052,-2.04922220919738,
-0.00118366394785932));
#19717=CARTESIAN_POINT('Ctrl Pts',(-3.24131509567094,-1.14500960679258,
-0.00118366394785932));
#19718=CARTESIAN_POINT('Ctrl Pts',(-3.12302133028127,-2.08244503428843,
0.0470540298718583));
#19719=CARTESIAN_POINT('Ctrl Pts',(-3.36530436688169,-1.17823243188363,
0.0470540298718583));
#19720=CARTESIAN_POINT('Ctrl Pts',(-3.22918310709556,-2.11089099665287,
0.120497232333251));
#19721=CARTESIAN_POINT('Ctrl Pts',(-3.47146614369598,-1.20667839424807,
0.120497232333251));
#19722=CARTESIAN_POINT('Ctrl Pts',(-3.31346873731432,-2.13347526320353,
0.224659532804408));
#19723=CARTESIAN_POINT('Ctrl Pts',(-3.55575177391474,-1.22926266079873,
0.224659532804408));
#19724=CARTESIAN_POINT('Ctrl Pts',(-3.37517559262903,-2.15000956525257,
0.364350357241515));
#19725=CARTESIAN_POINT('Ctrl Pts',(-3.61745862922945,-1.24579696284777,
0.364350357241515));
#19726=CARTESIAN_POINT('Ctrl Pts',(-3.41644600752903,-2.16106793959632,
0.538436816836325));
#19727=CARTESIAN_POINT('Ctrl Pts',(-3.65872904412945,-1.25685533719152,
0.538436816836325));
#19728=CARTESIAN_POINT('Ctrl Pts',(-3.44138817170702,-2.1677511723453,0.741129277895169));
#19729=CARTESIAN_POINT('Ctrl Pts',(-3.68367120830744,-1.2635385699405,0.741129277895169));
#19730=CARTESIAN_POINT('Ctrl Pts',(-3.45509438921434,-2.17142374225767,
0.964078729991154));
#19731=CARTESIAN_POINT('Ctrl Pts',(-3.69737742581476,-1.26721113985287,
0.964078729991154));
#19732=CARTESIAN_POINT('Ctrl Pts',(-3.46269762636911,-2.17346102351316,
1.1981954227983));
#19733=CARTESIAN_POINT('Ctrl Pts',(-3.70498066296953,-1.26924842110836,
1.1981954227983));
#19734=CARTESIAN_POINT('Ctrl Pts',(-3.46841399972688,-2.174992721138,1.43558101932923));
#19735=CARTESIAN_POINT('Ctrl Pts',(-3.7106970363273,-1.2707801187332,1.43558101932923));
#19736=CARTESIAN_POINT('Ctrl Pts',(-3.47458546703248,-2.17664636081866,
1.67142113207667));
#19737=CARTESIAN_POINT('Ctrl Pts',(-3.7168685036329,-1.27243375841386,1.67142113207667));
#19738=CARTESIAN_POINT('Ctrl Pts',(-3.48220149854979,-2.17868707031325,
1.90332556813333));
#19739=CARTESIAN_POINT('Ctrl Pts',(-3.72448453515021,-1.27447446790845,
1.90332556813333));
#19740=CARTESIAN_POINT('Ctrl Pts',(-3.4914193762178,-2.18115699319032,2.130657485557));
#19741=CARTESIAN_POINT('Ctrl Pts',(-3.73370241281822,-1.27694439078552,
2.130657485557));
#19742=CARTESIAN_POINT('Ctrl Pts',(-3.5021005762575,-2.18401901211515,2.35385258470204));
#19743=CARTESIAN_POINT('Ctrl Pts',(-3.74438361285792,-1.27980640971035,
2.35385258470204));
#19744=CARTESIAN_POINT('Ctrl Pts',(-3.51430453423174,-2.18728905279882,
2.57377631141659));
#19745=CARTESIAN_POINT('Ctrl Pts',(-3.75658757083216,-1.28307645039402,
2.57377631141659));
#19746=CARTESIAN_POINT('Ctrl Pts',(-3.52888713930413,-2.1911964500515,2.7909834104825));
#19747=CARTESIAN_POINT('Ctrl Pts',(-3.77117017590455,-1.2869838476467,2.7909834104825));
#19748=CARTESIAN_POINT('Ctrl Pts',(-3.54776587690305,-2.19625499254525,
3.00529120729338));
#19749=CARTESIAN_POINT('Ctrl Pts',(-3.79004891350347,-1.29204239014045,
3.00529120729338));
#19750=CARTESIAN_POINT('Ctrl Pts',(-3.5734970281571,-2.2031496337441,3.21600287470921));
#19751=CARTESIAN_POINT('Ctrl Pts',(-3.81578006475752,-1.2989370313393,3.21600287470921));
#19752=CARTESIAN_POINT('Ctrl Pts',(-3.6089962299041,-2.21266161618416,3.42199345348447));
#19753=CARTESIAN_POINT('Ctrl Pts',(-3.85127926650452,-1.30844901377936,
3.42199345348447));
#19754=CARTESIAN_POINT('Ctrl Pts',(-3.65720432068032,-2.22557893517629,
3.62185203209171));
#19755=CARTESIAN_POINT('Ctrl Pts',(-3.89948735728074,-1.32136633277149,
3.62185203209171));
#19756=CARTESIAN_POINT('Ctrl Pts',(-3.72077066456812,-2.24261148568683,
3.81399668859083));
#19757=CARTESIAN_POINT('Ctrl Pts',(-3.96305370116854,-1.33839888328203,
3.81399668859083));
#19758=CARTESIAN_POINT('Ctrl Pts',(-3.80174620003347,-2.26430881502145,
3.99681013615577));
#19759=CARTESIAN_POINT('Ctrl Pts',(-4.04402923663389,-1.36009621261665,
3.99681013615577));
#19760=CARTESIAN_POINT('Ctrl Pts',(-3.90148874704625,-2.29103474994454,
4.16885849319142));
#19761=CARTESIAN_POINT('Ctrl Pts',(-4.14377178364667,-1.38682214753974,
4.16885849319142));
#19762=CARTESIAN_POINT('Ctrl Pts',(-4.02054420699703,-2.32293556429287,
4.32911151507774));
#19763=CARTESIAN_POINT('Ctrl Pts',(-4.26282724359745,-1.41872296188807,
4.32911151507774));
#19764=CARTESIAN_POINT('Ctrl Pts',(-4.15854750309224,-2.35991343603441,
4.47714872481861));
#19765=CARTESIAN_POINT('Ctrl Pts',(-4.40083053969266,-1.45570083362961,
4.47714872481861));
#19766=CARTESIAN_POINT('Ctrl Pts',(-4.31409039163966,-2.4015910274091,4.61340315498244));
#19767=CARTESIAN_POINT('Ctrl Pts',(-4.55637342824008,-1.4973784250043,4.61340315498244));
#19768=CARTESIAN_POINT('Ctrl Pts',(-4.48467719669913,-2.44729962406419,
4.73929437247796));
#19769=CARTESIAN_POINT('Ctrl Pts',(-4.72696023329955,-1.54308702165939,
4.73929437247796));
#19770=CARTESIAN_POINT('Ctrl Pts',(-4.66714498312739,-2.49619172008234,
4.8567611153285));
#19771=CARTESIAN_POINT('Ctrl Pts',(-4.90942801972781,-1.59197911767754,
4.8567611153285));
#19772=CARTESIAN_POINT('Ctrl Pts',(-4.85801940569448,-2.54733636746495,
4.96787993373728));
#19773=CARTESIAN_POINT('Ctrl Pts',(-5.1003024422949,-1.64312376506015,4.96787993373728));
#19774=CARTESIAN_POINT('Ctrl Pts',(-5.05390797582409,-2.59982455163766,
5.07442896098937));
#19775=CARTESIAN_POINT('Ctrl Pts',(-5.29619101242451,-1.69561194923286,
5.07442896098937));
#19776=CARTESIAN_POINT('Ctrl Pts',(-5.25184849987638,-2.65286255520687,
5.17752467829109));
#19777=CARTESIAN_POINT('Ctrl Pts',(-5.4941315364768,-1.74864995280207,5.17752467829109));
#19778=CARTESIAN_POINT('Ctrl Pts',(-5.44975127134264,-2.70589044300113,
5.27709955371564));
#19779=CARTESIAN_POINT('Ctrl Pts',(-5.69203430794306,-1.80167784059633,
5.27709955371564));
#19780=CARTESIAN_POINT('Ctrl Pts',(-5.64631849853272,-2.75856047278514,
5.37226655127787));
#19781=CARTESIAN_POINT('Ctrl Pts',(-5.88860153513314,-1.85434787038034,
5.37226655127787));
#19782=CARTESIAN_POINT('Ctrl Pts',(-5.84079435728585,-2.81067012208539,
5.46195513100446));
#19783=CARTESIAN_POINT('Ctrl Pts',(-6.08307739388627,-1.90645751968059,
5.46195513100446));
#19784=CARTESIAN_POINT('Ctrl Pts',(-6.03277494512045,-2.86211116555812,
5.54547963906637));
#19785=CARTESIAN_POINT('Ctrl Pts',(-6.27505798172087,-1.95789856315332,
5.54547963906637));
#19786=CARTESIAN_POINT('Ctrl Pts',(-6.22198506429037,-2.9128098641895,5.62308582598972));
#19787=CARTESIAN_POINT('Ctrl Pts',(-6.46426810089079,-2.0085972617847,5.62308582598972));
#19788=CARTESIAN_POINT('Ctrl Pts',(-6.40808875598458,-2.96267619808741,
5.69662713609756));
#19789=CARTESIAN_POINT('Ctrl Pts',(-6.650371792585,-2.05846359568261,5.69662713609756));
#19790=CARTESIAN_POINT('Ctrl Pts',(-6.59042580657019,-3.0115332635421,5.76979878895672));
#19791=CARTESIAN_POINT('Ctrl Pts',(-6.83270884317061,-2.1073206611373,5.76979878895672));
#19792=CARTESIAN_POINT('Ctrl Pts',(-6.76762280561976,-3.05901305633865,
5.84723737025949));
#19793=CARTESIAN_POINT('Ctrl Pts',(-7.00990584222018,-2.15480045393385,
5.84723737025949));
#19794=CARTESIAN_POINT('Ctrl Pts',(-6.9371751657527,-3.10444447431107,5.93381436957244));
#19795=CARTESIAN_POINT('Ctrl Pts',(-7.17945820235312,-2.20023187190627,
5.93381436957244));
#19796=CARTESIAN_POINT('Ctrl Pts',(-7.09515091250332,-3.1467739480766,6.03389995867283));
#19797=CARTESIAN_POINT('Ctrl Pts',(-7.33743394910374,-2.2425613456718,6.03389995867283));
#19798=CARTESIAN_POINT('Ctrl Pts',(-7.23557821360659,-3.1844013300025,6.15052660592937));
#19799=CARTESIAN_POINT('Ctrl Pts',(-7.47786125020701,-2.2801887275977,6.15052660592937));
#19800=CARTESIAN_POINT('Ctrl Pts',(-7.35087158753979,-3.21529409644056,
6.28498018271686));
#19801=CARTESIAN_POINT('Ctrl Pts',(-7.59315462414021,-2.31108149403576,
6.28498018271686));
#19802=CARTESIAN_POINT('Ctrl Pts',(-7.43419435930806,-3.23762036584699,
6.43720976255636));
#19803=CARTESIAN_POINT('Ctrl Pts',(-7.67647739590848,-2.33340776344219,
6.43720976255636));
#19804=CARTESIAN_POINT('Ctrl Pts',(-7.48135699513883,-3.25025755603077,
6.60605451948903));
#19805=CARTESIAN_POINT('Ctrl Pts',(-7.72364003173925,-2.34604495362597,
6.60605451948903));
#19806=CARTESIAN_POINT('Ctrl Pts',(-7.49298027075354,-3.25337200334513,
6.78954489191904));
#19807=CARTESIAN_POINT('Ctrl Pts',(-7.73526330735396,-2.34915940094033,
6.78954489191904));
#19808=CARTESIAN_POINT('Ctrl Pts',(-7.4763273285188,-3.24890986092173,6.9851692342788));
#19809=CARTESIAN_POINT('Ctrl Pts',(-7.71861036511922,-2.34469725851693,
6.9851692342788));
#19810=CARTESIAN_POINT('Ctrl Pts',(-7.44241271429029,-3.23982246742759,
7.19009032473164));
#19811=CARTESIAN_POINT('Ctrl Pts',(-7.68469575089071,-2.33560986502279,
7.19009032473164));
#19812=CARTESIAN_POINT('Ctrl Pts',(-7.40329663075682,-3.22934134443373,
7.40136016279791));
#19813=CARTESIAN_POINT('Ctrl Pts',(-7.64557966735724,-2.32512874202893,
7.40136016279791));
#19814=CARTESIAN_POINT('Ctrl Pts',(-7.36935674832032,-3.22024718034366,
7.61613341658677));
#19815=CARTESIAN_POINT('Ctrl Pts',(-7.61163978492074,-2.31603457793886,
7.61613341658677));
#19816=CARTESIAN_POINT('Ctrl Pts',(-7.34646170831648,-3.21411247286395,
7.83188673232793));
#19817=CARTESIAN_POINT('Ctrl Pts',(-7.5887447449169,-2.30989987045915,7.83188673232793));
#19818=CARTESIAN_POINT('Ctrl Pts',(-7.33349443681848,-3.21063790293803,
8.04662057355248));
#19819=CARTESIAN_POINT('Ctrl Pts',(-7.5757774734189,-2.30642530053323,8.04662057355248));
#19820=CARTESIAN_POINT('Ctrl Pts',(-7.32478130400418,-3.20830322603689,
8.25883677791483));
#19821=CARTESIAN_POINT('Ctrl Pts',(-7.5670643406046,-2.30409062363209,8.25883677791483));
#19822=CARTESIAN_POINT('Ctrl Pts',(-7.31218544940774,-3.2049281769698,8.46752658699528));
#19823=CARTESIAN_POINT('Ctrl Pts',(-7.55446848600816,-2.300715574565,8.46752658699528));
#19824=CARTESIAN_POINT('Ctrl Pts',(-7.28737839225422,-3.19828114603892,
8.67216210283896));
#19825=CARTESIAN_POINT('Ctrl Pts',(-7.52966142885464,-2.29406854363412,
8.67216210283896));
#19826=CARTESIAN_POINT('Ctrl Pts',(-7.24391800390076,-3.18663597007687,
8.87266947141823));
#19827=CARTESIAN_POINT('Ctrl Pts',(-7.48620104050118,-2.28242336767207,
8.87266947141823));
#19828=CARTESIAN_POINT('Ctrl Pts',(-7.17972079495768,-3.16943437978424,
9.06945407016992));
#19829=CARTESIAN_POINT('Ctrl Pts',(-7.4220038315581,-2.26522177737944,9.06945407016992));
#19830=CARTESIAN_POINT('Ctrl Pts',(-7.09614123761334,-3.14703930489007,
9.26297089919765));
#19831=CARTESIAN_POINT('Ctrl Pts',(-7.33842427421376,-2.24282670248527,
9.26297089919765));
#19832=CARTESIAN_POINT('Ctrl Pts',(-6.99656158928535,-3.12035701853801,
9.4532499945042));
#19833=CARTESIAN_POINT('Ctrl Pts',(-7.23884462588577,-2.21614441613321,
9.4532499945042));
#19834=CARTESIAN_POINT('Ctrl Pts',(-6.88509891533857,-3.09049068506776,
9.63939026966035));
#19835=CARTESIAN_POINT('Ctrl Pts',(-7.12738195193899,-2.18627808266296,
9.63939026966035));
#19836=CARTESIAN_POINT('Ctrl Pts',(-6.76538664525988,-3.05841387897608,
9.81917361987397));
#19837=CARTESIAN_POINT('Ctrl Pts',(-7.0076696818603,-2.15420127657128,9.81917361987397));
#19838=CARTESIAN_POINT('Ctrl Pts',(-6.63901215031964,-3.02455193511295,
9.98835756998572));
#19839=CARTESIAN_POINT('Ctrl Pts',(-6.88129518692006,-2.12033933270815,
9.98835756998572));
#19840=CARTESIAN_POINT('Ctrl Pts',(-6.5056926897586,-2.98882909332026,10.1414720974148));
#19841=CARTESIAN_POINT('Ctrl Pts',(-6.74797572635902,-2.08461649091546,
10.1414720974148));
#19842=CARTESIAN_POINT('Ctrl Pts',(-6.36431879979372,-2.95094807367333,
10.2733319413008));
#19843=CARTESIAN_POINT('Ctrl Pts',(-6.60660183639414,-2.04673547126853,
10.2733319413008));
#19844=CARTESIAN_POINT('Ctrl Pts',(-6.21376535173928,-2.91060739884942,
10.3804015453596));
#19845=CARTESIAN_POINT('Ctrl Pts',(-6.4560483883397,-2.00639479644462,10.3804015453596));
#19846=CARTESIAN_POINT('Ctrl Pts',(-6.05370969899924,-2.86772061595369,
10.4620502678778));
#19847=CARTESIAN_POINT('Ctrl Pts',(-6.29599273559966,-1.96350801354889,
10.4620502678778));
#19848=CARTESIAN_POINT('Ctrl Pts',(-5.88567460802205,-2.82269574902626,
10.522290883026));
#19849=CARTESIAN_POINT('Ctrl Pts',(-6.12795764462247,-1.91848314662146,
10.522290883026));
#19850=CARTESIAN_POINT('Ctrl Pts',(-5.71262166386122,-2.77632635239054,
10.5687216653902));
#19851=CARTESIAN_POINT('Ctrl Pts',(-5.95490470046164,-1.87211374998574,
10.5687216653902));
#19852=CARTESIAN_POINT('Ctrl Pts',(-5.53795302541203,-2.72952403177503,
10.6103475969885));
#19853=CARTESIAN_POINT('Ctrl Pts',(-5.78023606201245,-1.82531142937023,
10.6103475969885));
#19854=CARTESIAN_POINT('Ctrl Pts',(-5.36474479343613,-2.68311302589467,
10.6558377434043));
#19855=CARTESIAN_POINT('Ctrl Pts',(-5.60702783003655,-1.77890042348987,
10.6558377434043));
#19856=CARTESIAN_POINT('Ctrl Pts',(-5.19479751149305,-2.63757578894216,
10.7114411549114));
#19857=CARTESIAN_POINT('Ctrl Pts',(-5.43708054809347,-1.73336318653736,
10.7114411549114));
#19858=CARTESIAN_POINT('Ctrl Pts',(-5.02801887021532,-2.59288758669703,
10.7795199127535));
#19859=CARTESIAN_POINT('Ctrl Pts',(-5.27030190681574,-1.68867498429223,
10.7795199127535));
#19860=CARTESIAN_POINT('Ctrl Pts',(-4.86332857677405,-2.5487589555682,10.8599381259737));
#19861=CARTESIAN_POINT('Ctrl Pts',(-5.10561161337447,-1.6445463531634,10.8599381259737));
#19862=CARTESIAN_POINT('Ctrl Pts',(-4.69942419919693,-2.50484090996048,
10.9511663773826));
#19863=CARTESIAN_POINT('Ctrl Pts',(-4.94170723579735,-1.60062830755568,
10.9511663773826));
#19864=CARTESIAN_POINT('Ctrl Pts',(-4.53550776406181,-2.46091963353984,
11.0513704191329));
#19865=CARTESIAN_POINT('Ctrl Pts',(-4.77779080066223,-1.55670703113504,
11.0513704191329));
#19866=CARTESIAN_POINT('Ctrl Pts',(-4.37225446646398,-2.41717604428678,
11.1598106424589));
#19867=CARTESIAN_POINT('Ctrl Pts',(-4.6145375030644,-1.51296344188198,11.1598106424589));
#19868=CARTESIAN_POINT('Ctrl Pts',(-4.2117643371012,-2.37417284373086,11.2768795166235));
#19869=CARTESIAN_POINT('Ctrl Pts',(-4.45404737370162,-1.46996024132606,
11.2768795166235));
#19870=CARTESIAN_POINT('Ctrl Pts',(-4.05659783059815,-2.33259610362101,
11.4029224160731));
#19871=CARTESIAN_POINT('Ctrl Pts',(-4.29888086719857,-1.42838350121621,
11.4029224160731));
#19872=CARTESIAN_POINT('Ctrl Pts',(-3.90903315889734,-2.29305626900741,
11.5373242211527));
#19873=CARTESIAN_POINT('Ctrl Pts',(-4.15131619549776,-1.38884366660261,
11.5373242211527));
#19874=CARTESIAN_POINT('Ctrl Pts',(-3.77030699189688,-2.25588470459057,
11.6776492463597));
#19875=CARTESIAN_POINT('Ctrl Pts',(-4.0125900284973,-1.35167210218577,11.6776492463597));
#19876=CARTESIAN_POINT('Ctrl Pts',(-3.63967882884875,-2.22088299379307,
11.8183570873721));
#19877=CARTESIAN_POINT('Ctrl Pts',(-3.88196186544917,-1.31667039138827,
11.8183570873721));
#19878=CARTESIAN_POINT('Ctrl Pts',(-3.51435496549085,-2.18730256581397,
11.9514202619522));
#19879=CARTESIAN_POINT('Ctrl Pts',(-3.75663800209127,-1.28308996340917,
11.9514202619522));
#19880=CARTESIAN_POINT('Ctrl Pts',(-3.39011325532028,-2.1540120999075,12.0684942936867));
#19881=CARTESIAN_POINT('Ctrl Pts',(-3.6323962919207,-1.2497994975027,12.0684942936867));
#19882=CARTESIAN_POINT('Ctrl Pts',(-3.26172495134207,-2.11961055753894,
12.1626050652586));
#19883=CARTESIAN_POINT('Ctrl Pts',(-3.50400798794249,-1.21539795513414,
12.1626050652586));
#19884=CARTESIAN_POINT('Ctrl Pts',(-3.12345991910123,-2.08256255380854,
12.2301117722809));
#19885=CARTESIAN_POINT('Ctrl Pts',(-3.36574295570165,-1.17834995140374,
12.2301117722809));
#19886=CARTESIAN_POINT('Ctrl Pts',(-2.96955541126968,-2.04132396522357,
12.2723364229645));
#19887=CARTESIAN_POINT('Ctrl Pts',(-3.2118384478701,-1.13711136281877,12.2723364229645));
#19888=CARTESIAN_POINT('Ctrl Pts',(-2.79463396275701,-1.99445390435572,
12.2938762651139));
#19889=CARTESIAN_POINT('Ctrl Pts',(-3.03691699935743,-1.09024130195092,
12.2938762651139));
#19890=CARTESIAN_POINT('Ctrl Pts',(-2.59413751717341,-1.94073104367628,
12.3010487961981));
#19891=CARTESIAN_POINT('Ctrl Pts',(-2.83642055377383,-1.03651844127148,
12.3010487961981));
#19892=CARTESIAN_POINT('Ctrl Pts',(-2.3647179830369,-1.87925826477648,12.300400839059));
#19893=CARTESIAN_POINT('Ctrl Pts',(-2.60700101963732,-0.975045662371677,
12.300400839059));
#19894=CARTESIAN_POINT('Ctrl Pts',(-2.10473899353102,-1.80959710448932,
12.2969132923574));
#19895=CARTESIAN_POINT('Ctrl Pts',(-2.34702203013144,-0.905384502084517,
12.2969132923574));
#19896=CARTESIAN_POINT('Ctrl Pts',(-1.81431310880745,-1.73177772321654,
12.2935845551224));
#19897=CARTESIAN_POINT('Ctrl Pts',(-2.05659614540787,-0.827565120811737,
12.2935845551224));
#19898=CARTESIAN_POINT('Ctrl Pts',(-1.49502196421663,-1.64622391887302,
12.2919684497906));
#19899=CARTESIAN_POINT('Ctrl Pts',(-1.73730500081705,-0.742011316468217,
12.2919684497906));
#19900=CARTESIAN_POINT('Ctrl Pts',(-1.14973065532629,-1.55370339150237,
12.2924280531798));
#19901=CARTESIAN_POINT('Ctrl Pts',(-1.39201369192671,-0.649490789097567,
12.2924280531798));
#19902=CARTESIAN_POINT('Ctrl Pts',(-0.782363392512268,-1.45526763010572,
12.2945066442122));
#19903=CARTESIAN_POINT('Ctrl Pts',(-1.02464642911269,-0.551055027700917,
12.2945066442122));
#19904=CARTESIAN_POINT('Ctrl Pts',(-0.39769588314259,-1.35219628161563,
12.2972483292773));
#19905=CARTESIAN_POINT('Ctrl Pts',(-0.63997891974301,-0.447983679210827,
12.2972483292773));
#19906=CARTESIAN_POINT('Ctrl Pts',(-0.0804516762334893,-1.26719095257088,
12.299081889758));
#19907=CARTESIAN_POINT('Ctrl Pts',(-0.322734712833909,-0.362978350166077,
12.299081889758));
#19908=CARTESIAN_POINT('Ctrl Pts',(0.160204003053163,-1.20270745765206,
12.2998330708668));
#19909=CARTESIAN_POINT('Ctrl Pts',(-0.0820790335472567,-0.298494855247257,
12.2998330708668));
#19910=CARTESIAN_POINT('Ctrl Pts',(0.321044459482073,-1.15961038724168,
12.2999999999989));
#19911=CARTESIAN_POINT('Ctrl Pts',(0.0787614228816533,-0.255397784836877,
12.2999999999989));
#19912=CARTESIAN_POINT('Ctrl Pts',(0.401464687696516,-1.13806185203649,
12.3));
#19913=CARTESIAN_POINT('Ctrl Pts',(0.159181651096096,-0.233849249631687,
12.3));
#19914=CARTESIAN_POINT('Ctrl Pts',(0.481884915910943,-1.11651331683131,
12.3000000000011));
#19915=CARTESIAN_POINT('Ctrl Pts',(0.239601879310523,-0.212300714426507,
12.3000000000011));
#19916=CARTESIAN_POINT('Ctrl Pts',(0.642725372339789,-1.07341624642095,
12.2998330708736));
#19917=CARTESIAN_POINT('Ctrl Pts',(0.400442335739369,-0.169203644016147,
12.2998330708736));
#19918=CARTESIAN_POINT('Ctrl Pts',(0.883381051626486,-1.00893275150212,
12.2990818897713));
#19919=CARTESIAN_POINT('Ctrl Pts',(0.641098015026066,-0.104720149097317,
12.2990818897713));
#19920=CARTESIAN_POINT('Ctrl Pts',(1.20062525853542,-0.923927422457416,
12.2972483292974));
#19921=CARTESIAN_POINT('Ctrl Pts',(0.958342221935,-0.019714820052613,12.2972483292974));
#19922=CARTESIAN_POINT('Ctrl Pts',(1.58529276790501,-0.82085607396734,12.2945066442369));
#19923=CARTESIAN_POINT('Ctrl Pts',(1.34300973130459,0.083356528437463,12.2945066442369));
#19924=CARTESIAN_POINT('Ctrl Pts',(1.95266003071895,-0.722420312570714,
12.2924280532047));
#19925=CARTESIAN_POINT('Ctrl Pts',(1.71037699411853,0.181792289834089,12.2924280532047));
#19926=CARTESIAN_POINT('Ctrl Pts',(2.29795133960928,-0.629899785200065,
12.291968449812));
#19927=CARTESIAN_POINT('Ctrl Pts',(2.05566830300886,0.274312817204738,12.291968449812));
#19928=CARTESIAN_POINT('Ctrl Pts',(2.61724248420015,-0.544345980856534,
12.2935845551378));
#19929=CARTESIAN_POINT('Ctrl Pts',(2.37495944759973,0.359866621548269,12.2935845551378));
#19930=CARTESIAN_POINT('Ctrl Pts',(2.90766836892382,-0.46652659958373,12.2969132923658));
#19931=CARTESIAN_POINT('Ctrl Pts',(2.6653853323234,0.437686002821073,12.2969132923658));
#19932=CARTESIAN_POINT('Ctrl Pts',(3.16764735842983,-0.396865439296537,
12.3004008390612));
#19933=CARTESIAN_POINT('Ctrl Pts',(2.92536432182941,0.507347163108266,12.3004008390612));
#19934=CARTESIAN_POINT('Ctrl Pts',(3.39706689256644,-0.335392660396708,
12.3010487961961));
#19935=CARTESIAN_POINT('Ctrl Pts',(3.15478385596602,0.568819942008095,12.3010487961961));
#19936=CARTESIAN_POINT('Ctrl Pts',(3.59756333815007,-0.281669799717264,
12.2938762651102));
#19937=CARTESIAN_POINT('Ctrl Pts',(3.35528030154965,0.622542802687539,12.2938762651102));
#19938=CARTESIAN_POINT('Ctrl Pts',(3.77248478666274,-0.234799738849412,
12.2723364229612));
#19939=CARTESIAN_POINT('Ctrl Pts',(3.53020175006232,0.669412863555391,12.2723364229612));
#19940=CARTESIAN_POINT('Ctrl Pts',(3.92638929449424,-0.19356115026445,12.2301117722792));
#19941=CARTESIAN_POINT('Ctrl Pts',(3.68410625789382,0.710651452140353,12.2301117722792));
#19942=CARTESIAN_POINT('Ctrl Pts',(4.06465432673507,-0.156513146534059,
12.1626050652587));
#19943=CARTESIAN_POINT('Ctrl Pts',(3.82237129013465,0.747699455870744,12.1626050652587));
#19944=CARTESIAN_POINT('Ctrl Pts',(4.17641608075606,-0.126566674799447,
12.0806818325566));
#19945=CARTESIAN_POINT('Ctrl Pts',(3.93413304415564,0.777645927605356,12.0806818325566));
#19946=CARTESIAN_POINT('Ctrl Pts',(4.26016995678755,-0.104124891353834,
12.0046763352305));
#19947=CARTESIAN_POINT('Ctrl Pts',(4.01788692018713,0.800087711050969,12.0046763352305));
#19948=CARTESIAN_POINT('Ctrl Pts',(4.31892840257442,-0.0883806132567331,
11.9465013108381));
#19949=CARTESIAN_POINT('Ctrl Pts',(4.076645365974,0.81583198914807,11.9465013108381));
#19950=CARTESIAN_POINT('Ctrl Pts',(4.35289300399361,-0.0792798257352161,
11.9117811315282));
#19951=CARTESIAN_POINT('Ctrl Pts',(4.11060996739319,0.824932776669587,11.9117811315282));
#19952=CARTESIAN_POINT('Ctrl Pts',(4.3617605754817,-0.0769037671161592,
11.9026515720695));
#19953=CARTESIAN_POINT('Ctrl Pts',(4.11947753888128,0.827308835288644,11.9026515720695));
#19954=CARTESIAN_POINT('',(4.40285823325642,0.132224151085944,3.57811407583582));
#19955=CARTESIAN_POINT('Ctrl Pts',(4.40285823325641,0.132224151085904,3.57811407583577));
#19956=CARTESIAN_POINT('Ctrl Pts',(4.43940677028145,0.142017302066303,3.71456495367834));
#19957=CARTESIAN_POINT('Ctrl Pts',(4.53463296379915,0.167533083717659,3.9794750710438));
#19958=CARTESIAN_POINT('Ctrl Pts',(4.76097163197783,0.228180347072074,4.33028299830215));
#19959=CARTESIAN_POINT('Ctrl Pts',(5.06150763834345,0.308708727274215,4.61783411696581));
#19960=CARTESIAN_POINT('Ctrl Pts',(5.40852054959526,0.401690556607312,4.85362603977077));
#19961=CARTESIAN_POINT('Ctrl Pts',(5.77679893037258,0.500370451326437,5.05954568690866));
#19962=CARTESIAN_POINT('Ctrl Pts',(6.28064189604197,0.635374767089651,5.31961833864166));
#19963=CARTESIAN_POINT('Ctrl Pts',(6.81213487368419,0.777787881231695,5.56423083230834));
#19964=CARTESIAN_POINT('Ctrl Pts',(7.25326088523284,0.895987239786518,5.73088688746923));
#19965=CARTESIAN_POINT('Ctrl Pts',(7.60545358372097,0.990356988926552,5.88645382774441));
#19966=CARTESIAN_POINT('Ctrl Pts',(7.89304985394669,1.06741817727973,6.03509348122348));
#19967=CARTESIAN_POINT('Ctrl Pts',(8.13408614953057,1.13200365802803,6.32217794399327));
#19968=CARTESIAN_POINT('Ctrl Pts',(8.21367576229283,1.15332963049358,6.52713122561373));
#19969=CARTESIAN_POINT('Ctrl Pts',(8.24820562306135,1.16258187880126,6.74090493270784));
#19970=CARTESIAN_POINT('Ctrl Pts',(8.22962792994722,1.1576040009341,6.99851570691194));
#19971=CARTESIAN_POINT('Ctrl Pts',(8.15840156120257,1.13851895294917,7.38504607625248));
#19972=CARTESIAN_POINT('Ctrl Pts',(8.08669712828127,1.11930580805417,7.85408399146071));
#19973=CARTESIAN_POINT('Ctrl Pts',(8.08101604477191,1.11778356631571,8.34143039554977));
#19974=CARTESIAN_POINT('Ctrl Pts',(8.03131448784197,1.10446607427376,8.73832152751838));
#19975=CARTESIAN_POINT('Ctrl Pts',(7.92226315679741,1.07524585818683,9.12864980257357));
#19976=CARTESIAN_POINT('Ctrl Pts',(7.69129240392847,1.01335743148039,9.57126835989378));
#19977=CARTESIAN_POINT('Ctrl Pts',(7.4152185798584,0.939383673269444,9.97380310172652));
#19978=CARTESIAN_POINT('Ctrl Pts',(7.1368016643945,0.864782085611728,10.2639387973189));
#19979=CARTESIAN_POINT('Ctrl Pts',(6.88183638015527,0.796464343601853,10.4339697781547));
#19980=CARTESIAN_POINT('Ctrl Pts',(6.60023402171546,0.721009219071207,10.5367578512231));
#19981=CARTESIAN_POINT('Ctrl Pts',(6.22971711106489,0.621729512080313,10.623044675585));
#19982=CARTESIAN_POINT('Ctrl Pts',(5.93468051661777,0.542674694860579,10.7102223023981));
#19983=CARTESIAN_POINT('Ctrl Pts',(5.64132565171833,0.464070495715032,10.8473463161695));
#19984=CARTESIAN_POINT('Ctrl Pts',(5.39460105858856,0.397960840233013,10.9821160664838));
#19985=CARTESIAN_POINT('Ctrl Pts',(5.06953125376008,0.310858648545478,11.1942553330246));
#19986=CARTESIAN_POINT('Ctrl Pts',(4.74015401319374,0.222602282930538,11.4563092607288));
#19987=CARTESIAN_POINT('Ctrl Pts',(4.54249036453264,0.169638467898806,11.6591099894158));
#19988=CARTESIAN_POINT('Ctrl Pts',(4.44483865181741,0.143472770337245,11.7628168777948));
#19989=CARTESIAN_POINT('Ctrl Pts',(4.19359661830351,0.510762161999066,2.99727332026023));
#19990=CARTESIAN_POINT('Ctrl Pts',(4.21373513499808,0.476613798189458,3.09465434585502));
#19991=CARTESIAN_POINT('Ctrl Pts',(4.26953516459727,0.380870576396472,3.3133840657309));
#19992=CARTESIAN_POINT('Ctrl Pts',(4.35198159611048,0.232981640725298,3.49493665183918));
#19993=CARTESIAN_POINT('Ctrl Pts',(4.40285823325642,0.132224151085984,3.57811407583586));
#19994=CARTESIAN_POINT('Ctrl Pts',(4.40285823325641,0.132224151085904,3.57811407583577));
#19995=CARTESIAN_POINT('Ctrl Pts',(4.43940677028145,0.142017302066303,3.71456495367834));
#19996=CARTESIAN_POINT('Ctrl Pts',(4.53463296379915,0.167533083717659,3.9794750710438));
#19997=CARTESIAN_POINT('Ctrl Pts',(4.76097163197783,0.228180347072074,4.33028299830215));
#19998=CARTESIAN_POINT('Ctrl Pts',(5.06150763834345,0.308708727274215,4.61783411696581));
#19999=CARTESIAN_POINT('Ctrl Pts',(5.40852054959526,0.401690556607312,4.85362603977077));
#20000=CARTESIAN_POINT('Ctrl Pts',(5.77679893037258,0.500370451326437,5.05954568690866));
#20001=CARTESIAN_POINT('Ctrl Pts',(6.28064189604197,0.635374767089651,5.31961833864166));
#20002=CARTESIAN_POINT('Ctrl Pts',(6.81213487368419,0.777787881231695,5.56423083230834));
#20003=CARTESIAN_POINT('Ctrl Pts',(7.25326088523284,0.895987239786518,5.73088688746923));
#20004=CARTESIAN_POINT('Ctrl Pts',(7.60545358372097,0.990356988926552,5.88645382774441));
#20005=CARTESIAN_POINT('Ctrl Pts',(7.89304985394669,1.06741817727973,6.03509348122348));
#20006=CARTESIAN_POINT('Ctrl Pts',(8.13408614953057,1.13200365802803,6.32217794399327));
#20007=CARTESIAN_POINT('Ctrl Pts',(8.21367576229283,1.15332963049358,6.52713122561373));
#20008=CARTESIAN_POINT('Ctrl Pts',(8.24820562306135,1.16258187880126,6.74090493270784));
#20009=CARTESIAN_POINT('Ctrl Pts',(8.22962792994722,1.1576040009341,6.99851570691194));
#20010=CARTESIAN_POINT('Ctrl Pts',(8.15840156120257,1.13851895294917,7.38504607625248));
#20011=CARTESIAN_POINT('Ctrl Pts',(8.08669712828127,1.11930580805417,7.85408399146071));
#20012=CARTESIAN_POINT('Ctrl Pts',(8.08101604477191,1.11778356631571,8.34143039554977));
#20013=CARTESIAN_POINT('Ctrl Pts',(8.03131448784197,1.10446607427376,8.73832152751838));
#20014=CARTESIAN_POINT('Ctrl Pts',(7.92226315679741,1.07524585818683,9.12864980257357));
#20015=CARTESIAN_POINT('Ctrl Pts',(7.69129240392847,1.01335743148039,9.57126835989378));
#20016=CARTESIAN_POINT('Ctrl Pts',(7.4152185798584,0.939383673269444,9.97380310172652));
#20017=CARTESIAN_POINT('Ctrl Pts',(7.1368016643945,0.864782085611728,10.2639387973189));
#20018=CARTESIAN_POINT('Ctrl Pts',(6.88183638015527,0.796464343601853,10.4339697781547));
#20019=CARTESIAN_POINT('Ctrl Pts',(6.60023402171546,0.721009219071207,10.5367578512231));
#20020=CARTESIAN_POINT('Ctrl Pts',(6.22971711106489,0.621729512080313,10.623044675585));
#20021=CARTESIAN_POINT('Ctrl Pts',(5.93468051661777,0.542674694860579,10.7102223023981));
#20022=CARTESIAN_POINT('Ctrl Pts',(5.64132565171833,0.464070495715032,10.8473463161695));
#20023=CARTESIAN_POINT('Ctrl Pts',(5.39460105858856,0.397960840233013,10.9821160664838));
#20024=CARTESIAN_POINT('Ctrl Pts',(5.06953125376008,0.310858648545478,11.1942553330246));
#20025=CARTESIAN_POINT('Ctrl Pts',(4.74015401319374,0.222602282930538,11.4563092607288));
#20026=CARTESIAN_POINT('Ctrl Pts',(4.54249036453264,0.169638467898806,11.6591099894158));
#20027=CARTESIAN_POINT('Ctrl Pts',(4.44483865181741,0.143472770337245,11.7628168777948));
#20028=CARTESIAN_POINT('Ctrl Pts',(4.4090533114332,0.109103804573277,3.57811407583577));
#20029=CARTESIAN_POINT('Ctrl Pts',(4.44559813622809,0.118895960864605,3.71455109438044));
#20030=CARTESIAN_POINT('Ctrl Pts',(4.54083607335543,0.14441488920668,3.97948069543409));
#20031=CARTESIAN_POINT('Ctrl Pts',(4.7671666003941,0.205059971149203,4.33027237668467));
#20032=CARTESIAN_POINT('Ctrl Pts',(5.06769840870851,0.285587226486915,4.61782723492783));
#20033=CARTESIAN_POINT('Ctrl Pts',(5.41470997442562,0.378568695285074,4.85362027669949));
#20034=CARTESIAN_POINT('Ctrl Pts',(5.78299034154921,0.477249122244079,5.05954319866726));
#20035=CARTESIAN_POINT('Ctrl Pts',(6.28684021661948,0.612255289375677,5.31961985792902));
#20036=CARTESIAN_POINT('Ctrl Pts',(6.81832385480766,0.754665901018556,5.564227040406));
#20037=CARTESIAN_POINT('Ctrl Pts',(7.25944357588469,0.872863574046589,5.73087878972347));
#20038=CARTESIAN_POINT('Ctrl Pts',(7.61163865214237,0.967233960308051,5.88644101461346));
#20039=CARTESIAN_POINT('Ctrl Pts',(7.89922275747532,1.04429188908804,6.03505547921762));
#20040=CARTESIAN_POINT('Ctrl Pts',(8.14029443856229,1.10888685135331,6.32215841122141));
#20041=CARTESIAN_POINT('Ctrl Pts',(8.21989163690174,1.13021485636814,6.5271379469616));
#20042=CARTESIAN_POINT('Ctrl Pts',(8.25441840505932,1.13946627601322,6.74093595724302));
#20043=CARTESIAN_POINT('Ctrl Pts',(8.23582818046237,1.13448504034536,6.99854971389734));
#20044=CARTESIAN_POINT('Ctrl Pts',(8.16459707704539,1.1153987237088,7.3850681120554));
#20045=CARTESIAN_POINT('Ctrl Pts',(8.09289299023897,1.09618567155501,7.85407732011957));
#20046=CARTESIAN_POINT('Ctrl Pts',(8.0872159078158,1.09466450190436,8.34140461217029));
#20047=CARTESIAN_POINT('Ctrl Pts',(8.03751561754474,1.08134734926263,8.73830742082599));
#20048=CARTESIAN_POINT('Ctrl Pts',(7.92846039739064,1.05212609109194,9.12865849166385));
#20049=CARTESIAN_POINT('Ctrl Pts',(7.69748287548657,0.990235850628008,9.5712757246142));
#20050=CARTESIAN_POINT('Ctrl Pts',(7.42143118324782,0.916268022623389,9.97378978761487));
#20051=CARTESIAN_POINT('Ctrl Pts',(7.14300814718688,0.841664794956637,10.2639374823751));
#20052=CARTESIAN_POINT('Ctrl Pts',(6.88801376154103,0.773339255248362,10.4339879035537));
#20053=CARTESIAN_POINT('Ctrl Pts',(6.60641208432421,0.697884313250866,10.536766070865));
#20054=CARTESIAN_POINT('Ctrl Pts',(6.23589390298475,0.598604265779908,10.6230512239787));
#20055=CARTESIAN_POINT('Ctrl Pts',(5.94087044850798,0.519552969404618,10.7102267075257));
#20056=CARTESIAN_POINT('Ctrl Pts',(5.64752558195459,0.440951449307822,10.8473451314547));
#20057=CARTESIAN_POINT('Ctrl Pts',(5.40080787303593,0.37484363844461,10.9821110393344));
#20058=CARTESIAN_POINT('Ctrl Pts',(5.07572294615792,0.287737394816118,11.1942590991363));
#20059=CARTESIAN_POINT('Ctrl Pts',(4.74634791397138,0.19948162093476,11.4563122548706));
#20060=CARTESIAN_POINT('Ctrl Pts',(4.54868443730922,0.146517851990004,11.6591110571587));
#20061=CARTESIAN_POINT('Ctrl Pts',(4.4510337299942,0.120352423824617,11.7628168777948));
#20062=CARTESIAN_POINT('Ctrl Pts',(4.40106171131969,0.0640775387299355,
3.5834861945331));
#20063=CARTESIAN_POINT('Ctrl Pts',(4.43790303359015,0.0739491412803999,
3.72103016137481));
#20064=CARTESIAN_POINT('Ctrl Pts',(4.53402257603767,0.0997042950560617,
3.98857423439157));
#20065=CARTESIAN_POINT('Ctrl Pts',(4.76306341192281,0.161075602065234,4.34358222601213));
#20066=CARTESIAN_POINT('Ctrl Pts',(5.06667005322962,0.24242675642012,4.63394435000544));
#20067=CARTESIAN_POINT('Ctrl Pts',(5.41565268579315,0.335936370988005,4.87101890352248));
#20068=CARTESIAN_POINT('Ctrl Pts',(5.7849003361388,0.434875980705211,5.07744965319006));
#20069=CARTESIAN_POINT('Ctrl Pts',(6.28913493446496,0.569985234122539,5.33776665098138));
#20070=CARTESIAN_POINT('Ctrl Pts',(6.82196111316944,0.712755578412563,5.58292297422199));
#20071=CARTESIAN_POINT('Ctrl Pts',(7.26330723858452,0.83101391630014,5.74971217255928));
#20072=CARTESIAN_POINT('Ctrl Pts',(7.61396716546967,0.924972960526974,5.90453629054123));
#20073=CARTESIAN_POINT('Ctrl Pts',(7.89891366870189,1.00132414595412,6.05235368516109));
#20074=CARTESIAN_POINT('Ctrl Pts',(8.13437391799379,1.06441552960151,6.33330907644365));
#20075=CARTESIAN_POINT('Ctrl Pts',(8.21170963215847,1.08513757175802,6.53255536921129));
#20076=CARTESIAN_POINT('Ctrl Pts',(8.24550570678105,1.09419320266049,6.74112857932929));
#20077=CARTESIAN_POINT('Ctrl Pts',(8.22735380727456,1.08932941584663,6.99539650801542));
#20078=CARTESIAN_POINT('Ctrl Pts',(8.15627988619041,1.07028521608922,7.38089406911332));
#20079=CARTESIAN_POINT('Ctrl Pts',(8.08417079901181,1.05096364441277,7.8529025756585));
#20080=CARTESIAN_POINT('Ctrl Pts',(8.07851394340125,1.04944789452022,8.34085105008331));
#20081=CARTESIAN_POINT('Ctrl Pts',(8.02910143470183,1.03620785271821,8.73430700697211));
#20082=CARTESIAN_POINT('Ctrl Pts',(7.92127213001242,1.00731507760628,9.12048137472438));
#20083=CARTESIAN_POINT('Ctrl Pts',(7.69186349651382,0.9458452195236,9.56036990607636));
#20084=CARTESIAN_POINT('Ctrl Pts',(7.41674295651521,0.872126893009758,9.96140578441748));
#20085=CARTESIAN_POINT('Ctrl Pts',(7.14117040174745,0.798287449503556,10.2483733431293));
#20086=CARTESIAN_POINT('Ctrl Pts',(6.8902954129788,0.731065698861828,10.4156376689661));
#20087=CARTESIAN_POINT('Ctrl Pts',(6.61225089452466,0.65656389468214,10.5172850890292));
#20088=CARTESIAN_POINT('Ctrl Pts',(6.24261997408572,0.557521588052954,10.603363191263));
#20089=CARTESIAN_POINT('Ctrl Pts',(5.94489265314603,0.477745792842484,10.6912647738558));
#20090=CARTESIAN_POINT('Ctrl Pts',(5.6495876077844,0.398619044416999,10.8293357996365));
#20091=CARTESIAN_POINT('Ctrl Pts',(5.40165483192268,0.332185657347644,10.9647672453765));
#20092=CARTESIAN_POINT('Ctrl Pts',(5.07547427893545,0.244785841587978,11.1776402225937));
#20093=CARTESIAN_POINT('Ctrl Pts',(4.74424250329149,0.156032554796651,11.4411353182047));
#20094=CARTESIAN_POINT('Ctrl Pts',(4.5455807954736,0.102801310619861,11.6449924329457));
#20095=CARTESIAN_POINT('Ctrl Pts',(4.44784978639617,0.076614365662085,11.7487835346862));
#20096=CARTESIAN_POINT('Ctrl Pts',(4.36580935114124,0.0394748386098602,
3.59469433164577));
#20097=CARTESIAN_POINT('Ctrl Pts',(4.40325934412277,0.0495095339858135,
3.73451071920807));
#20098=CARTESIAN_POINT('Ctrl Pts',(4.50124963302018,0.0757659527619658,
4.00756161013495));
#20099=CARTESIAN_POINT('Ctrl Pts',(4.73592335833677,0.13864658794535,4.37132286716819));
#20100=CARTESIAN_POINT('Ctrl Pts',(5.0459339603424,0.221713678397845,4.66755193997466));
#20101=CARTESIAN_POINT('Ctrl Pts',(5.39902533614519,0.316324227398598,4.90730317213381));
#20102=CARTESIAN_POINT('Ctrl Pts',(5.77029639310752,0.415806007284703,5.11480218775024));
#20103=CARTESIAN_POINT('Ctrl Pts',(6.27535213809375,0.551135286286462,5.37563133408309));
#20104=CARTESIAN_POINT('Ctrl Pts',(6.81095435368323,0.694649467417985,5.6219191550161));
#20105=CARTESIAN_POINT('Ctrl Pts',(7.25275601568305,0.81302986596556,5.78898360528629));
#20106=CARTESIAN_POINT('Ctrl Pts',(7.60021943769446,0.906132409292876,5.94225516102438));
#20107=CARTESIAN_POINT('Ctrl Pts',(7.87963043829654,0.981000361260572,6.08834222260924));
#20108=CARTESIAN_POINT('Ctrl Pts',(8.10347789154437,1.04098010558609,6.35652106548154));
#20109=CARTESIAN_POINT('Ctrl Pts',(8.17611563731258,1.0604433309047,6.54387600067759));
#20110=CARTESIAN_POINT('Ctrl Pts',(8.20837895644931,1.06908826121254,6.74161342706472));
#20111=CARTESIAN_POINT('Ctrl Pts',(8.19110804451059,1.06446053430601,6.98890875288788));
#20112=CARTESIAN_POINT('Ctrl Pts',(8.12034939918785,1.04550081243426,7.37224447234147));
#20113=CARTESIAN_POINT('Ctrl Pts',(8.04739626380834,1.025953078724,7.85043380236922));
#20114=CARTESIAN_POINT('Ctrl Pts',(8.0417923087215,1.02445150348406,8.33962717062775));
#20115=CARTESIAN_POINT('Ctrl Pts',(7.99298360150036,1.01137324980055,8.72592300463577));
#20116=CARTESIAN_POINT('Ctrl Pts',(7.88770158869635,0.983163019492191,9.10344425805828));
#20117=CARTESIAN_POINT('Ctrl Pts',(7.66154810789234,0.922565376945272,9.53763621224937));
#20118=CARTESIAN_POINT('Ctrl Pts',(7.38842946831295,0.849383458032085,9.93553277313259));
#20119=CARTESIAN_POINT('Ctrl Pts',(7.11878765582192,0.777133152129452,10.2158975345821));
#20120=CARTESIAN_POINT('Ctrl Pts',(6.87642935703478,0.712193441690456,10.3774010714523));
#20121=CARTESIAN_POINT('Ctrl Pts',(6.60580815001857,0.639680707815727,10.476662862038));
#20122=CARTESIAN_POINT('Ctrl Pts',(6.23802497096264,0.541133501997939,10.5623045135241));
#20123=CARTESIAN_POINT('Ctrl Pts',(5.9346915702303,0.459855562234322,10.6517152633816));
#20124=CARTESIAN_POINT('Ctrl Pts',(5.63532363844642,0.379640166673058,10.7917588039818));
#20125=CARTESIAN_POINT('Ctrl Pts',(5.3848742144548,0.312532445769662,10.9285685208154));
#20126=CARTESIAN_POINT('Ctrl Pts',(5.05636735697362,0.224509298599493,11.1429774479459));
#20127=CARTESIAN_POINT('Ctrl Pts',(4.72126766459807,0.134719606643546,11.4094788749468));
#20128=CARTESIAN_POINT('Ctrl Pts',(4.52052375398258,0.0809304379086621,
11.6155388514382));
#20129=CARTESIAN_POINT('Ctrl Pts',(4.42262789584284,0.0546993217777655,
11.719505024182));
#20130=CARTESIAN_POINT('Ctrl Pts',(4.34909964308327,0.0349974858299679,
3.59949138964752));
#20131=CARTESIAN_POINT('Ctrl Pts',(4.38680976101687,0.0451018814767583,
3.74027893176065));
#20132=CARTESIAN_POINT('Ctrl Pts',(4.48560194249773,0.071573166723062,4.01568874810612));
#20133=CARTESIAN_POINT('Ctrl Pts',(4.72268568825884,0.135099564938299,4.38319469956436));
#20134=CARTESIAN_POINT('Ctrl Pts',(5.0354367362137,0.21890095566979,4.68193520114933));
#20135=CARTESIAN_POINT('Ctrl Pts',(5.39028650561027,0.313982664813972,4.92283216185341));
#20136=CARTESIAN_POINT('Ctrl Pts',(5.76242378203297,0.413696547504953,5.13078873237884));
#20137=CARTESIAN_POINT('Ctrl Pts',(6.26783169213932,0.54912018886625,5.39183749253912));
#20138=CARTESIAN_POINT('Ctrl Pts',(6.8046210773698,0.692952471144354,5.63860904148901));
#20139=CARTESIAN_POINT('Ctrl Pts',(7.24661705601864,0.811384936681117,5.80579085268058));
#20140=CARTESIAN_POINT('Ctrl Pts',(7.59271262743873,0.904120965547118,5.95839742644866));
#20141=CARTESIAN_POINT('Ctrl Pts',(7.8697531842168,0.978353759006469,6.10374129848354));
#20142=CARTESIAN_POINT('Ctrl Pts',(8.08863405403125,1.03700271131187,6.36645372110484));
#20143=CARTESIAN_POINT('Ctrl Pts',(8.15926186591506,1.05592737646932,6.54872190268123));
#20144=CARTESIAN_POINT('Ctrl Pts',(8.19086884853079,1.06439644193639,6.74182415651423));
#20145=CARTESIAN_POINT('Ctrl Pts',(8.17397369844545,1.05986940011502,6.98613553279737));
#20146=CARTESIAN_POINT('Ctrl Pts',(8.10334949970651,1.04094570309683,7.36854474797747));
#20147=CARTESIAN_POINT('Ctrl Pts',(8.03003514943051,1.02130118214676,7.84937648135502));
#20148=CARTESIAN_POINT('Ctrl Pts',(8.02445425036305,1.01980578474859,8.33910068047419));
#20149=CARTESIAN_POINT('Ctrl Pts',(7.97590410013386,1.00679681120227,8.72233320794333));
#20150=CARTESIAN_POINT('Ctrl Pts',(7.87171191954179,0.978878600554987,9.09615331026656));
#20151=CARTESIAN_POINT('Ctrl Pts',(7.64695093531355,0.918654076341007,9.5279070047071));
#20152=CARTESIAN_POINT('Ctrl Pts',(7.37469139866462,0.845702353364252,9.92445780127518));
#20153=CARTESIAN_POINT('Ctrl Pts',(7.10758729640882,0.774132024869772,10.2019978237482));
#20154=CARTESIAN_POINT('Ctrl Pts',(6.86887110582377,0.710168214382273,10.3610377706145));
#20155=CARTESIAN_POINT('Ctrl Pts',(6.60142713036405,0.638506817137273,10.4592774903079));
#20156=CARTESIAN_POINT('Ctrl Pts',(6.23443464884433,0.540171478085771,10.5447321686106));
#20157=CARTESIAN_POINT('Ctrl Pts',(5.92870322026153,0.458250988696196,10.6347886165848));
#20158=CARTESIAN_POINT('Ctrl Pts',(5.62759741836264,0.377569932241062,10.7756758097979));
#20159=CARTESIAN_POINT('Ctrl Pts',(5.37607158806058,0.310173789136056,10.9130750253569));
#20160=CARTESIAN_POINT('Ctrl Pts',(5.04656750998174,0.22188343751207,11.1281422470874));
#20161=CARTESIAN_POINT('Ctrl Pts',(4.70981258666106,0.131650227761089,11.3959302972882));
#20162=CARTESIAN_POINT('Ctrl Pts',(4.50817751566127,0.0776222733209033,
11.6029328940868));
#20163=CARTESIAN_POINT('Ctrl Pts',(4.4102112066954,0.0513722799480404,11.706973886163));
#20164=CARTESIAN_POINT('Origin',(4.32839411947507,0.112271551933094,3.59949138964752));
#20165=CARTESIAN_POINT('Origin',(4.33293714059227,0.0306667563398384,3.08701851589662));
#20166=CARTESIAN_POINT('Ctrl Pts',(4.33135810013194,0.0365598155649942,
11.6149485836148));
#20167=CARTESIAN_POINT('Ctrl Pts',(4.33187792676856,0.0346197961459941,
11.6082911303789));
#20168=CARTESIAN_POINT('Ctrl Pts',(4.33227188276068,0.0331495322847722,
11.6014592124169));
#20169=CARTESIAN_POINT('Ctrl Pts',(4.33280071341379,0.0311759094187438,
11.5876929996279));
#20170=CARTESIAN_POINT('Ctrl Pts',(4.33293714059227,0.0306667563398198,
11.5807132391622));
#20171=CARTESIAN_POINT('Ctrl Pts',(4.33293714059227,0.0306667563398385,
11.5737513317737));
#20172=CARTESIAN_POINT('Origin',(2.05,0.08,1.28));
#20173=CARTESIAN_POINT('',(-2.803641505311,0.,1.28));
#20174=CARTESIAN_POINT('',(2.05,0.,1.28));
#20175=CARTESIAN_POINT('',(-2.803641505311,0.08,1.2));
#20176=CARTESIAN_POINT('Origin',(-2.803641505311,0.08,1.28));
#20177=CARTESIAN_POINT('',(2.05,0.08,1.2));
#20178=CARTESIAN_POINT('Ctrl Pts',(-2.96341860243295,0.00343337974884617,
1.1214615033794));
#20179=CARTESIAN_POINT('Ctrl Pts',(-2.96630515786593,0.00868558376862438,
1.06150427209154));
#20180=CARTESIAN_POINT('Ctrl Pts',(-2.96893720254462,0.0199743192711058,
1.00206230831012));
#20181=CARTESIAN_POINT('Ctrl Pts',(-2.97150840940722,0.0370763911099046,
0.944338416612715));
#20182=CARTESIAN_POINT('Ctrl Pts',(-2.93958582132551,0.00354285648575689,
1.12021175717555));
#20183=CARTESIAN_POINT('Ctrl Pts',(-2.94251954168973,0.00887597719617225,
1.06031972093586));
#20184=CARTESIAN_POINT('Ctrl Pts',(-2.94518955488367,0.0202169542943542,
1.00097374956333));
#20185=CARTESIAN_POINT('Ctrl Pts',(-2.94780986467339,0.0373919530059805,
0.943273314040079));
#20186=CARTESIAN_POINT('Ctrl Pts',(-2.89832135056165,0.0236236998221979,
1.11979038686963));
#20187=CARTESIAN_POINT('Ctrl Pts',(-2.90132976176868,0.0288805527885566,
1.06138252620797));
#20188=CARTESIAN_POINT('Ctrl Pts',(-2.90406886065643,0.0400205415337996,
1.00340420949257));
#20189=CARTESIAN_POINT('Ctrl Pts',(-2.90676750629242,0.0568440093652064,
0.94702993218099));
#20190=CARTESIAN_POINT('Ctrl Pts',(-2.8836123610279,0.0652969522995559,
1.12266369893431));
#20191=CARTESIAN_POINT('Ctrl Pts',(-2.88654643974598,0.0702232785018827,
1.06706918382192));
#20192=CARTESIAN_POINT('Ctrl Pts',(-2.88922109707321,0.0807651986054815,
1.01185481384779));
#20193=CARTESIAN_POINT('Ctrl Pts',(-2.89185038905304,0.096718663397188,
0.958114462937943));
#20194=CARTESIAN_POINT('Ctrl Pts',(-2.88353005387197,0.0831281904378376,
1.12422135153951));
#20195=CARTESIAN_POINT('Ctrl Pts',(-2.88640514642651,0.08791353187808,1.06981058545882));
#20196=CARTESIAN_POINT('Ctrl Pts',(-2.88903159296831,0.0981988242247885,
1.01577166814133));
#20197=CARTESIAN_POINT('Ctrl Pts',(-2.89160384326392,0.113780711900135,
0.963157446086756));
#20198=CARTESIAN_POINT('',(-2.97150840945859,0.0370763914516166,0.944338415459349));
#20199=CARTESIAN_POINT('',(-2.89160384334168,0.113780712456408,0.963157444496232));
#20200=CARTESIAN_POINT('Origin',(-2.97150840940722,0.113780711900135,0.967063890691585));
#20201=CARTESIAN_POINT('',(-2.88353005387197,0.0831281904378376,1.12422135153951));
#20202=CARTESIAN_POINT('Ctrl Pts',(-2.89160384326392,0.113780711900135,
0.963157446086756));
#20203=CARTESIAN_POINT('Ctrl Pts',(-2.88903159296831,0.0981988242247885,
1.01577166814133));
#20204=CARTESIAN_POINT('Ctrl Pts',(-2.88640514642651,0.08791353187808,1.06981058545882));
#20205=CARTESIAN_POINT('Ctrl Pts',(-2.88353005387197,0.0831281904378376,
1.12422135153951));
#20206=CARTESIAN_POINT('',(-2.96341860243295,0.00343337974884617,1.1214615033794));
#20207=CARTESIAN_POINT('Origin',(-2.96341860243295,0.0831281904378376,1.12844270307901));
#20208=CARTESIAN_POINT('Ctrl Pts',(-2.96341860243295,0.00343337974884617,
1.1214615033794));
#20209=CARTESIAN_POINT('Ctrl Pts',(-2.96630515786593,0.00868558376862438,
1.06150427209154));
#20210=CARTESIAN_POINT('Ctrl Pts',(-2.96893720254462,0.0199743192711058,
1.00206230831012));
#20211=CARTESIAN_POINT('Ctrl Pts',(-2.97150840940722,0.0370763911099046,
0.944338416612715));
#20212=CARTESIAN_POINT('Ctrl Pts',(-2.94220556991652,1.38777878078145E-17,
1.19999999999997));
#20213=CARTESIAN_POINT('Ctrl Pts',(-2.95477525929363,7.99204335707293E-16,
1.17610462613062));
#20214=CARTESIAN_POINT('Ctrl Pts',(-2.96209712200597,0.00102889281907461,
1.14891024269609));
#20215=CARTESIAN_POINT('Ctrl Pts',(-2.96341860243295,0.00343337974884619,
1.1214615033794));
#20216=CARTESIAN_POINT('Ctrl Pts',(-2.92147643432527,4.12491330437235E-16,
1.1880320279863));
#20217=CARTESIAN_POINT('Ctrl Pts',(-2.93233653942741,0.0003274672410604,
1.16750429943543));
#20218=CARTESIAN_POINT('Ctrl Pts',(-2.93864796914417,0.00143185455554525,
1.14395403171255));
#20219=CARTESIAN_POINT('Ctrl Pts',(-2.93958582132551,0.00354285648575692,
1.12021175717555));
#20220=CARTESIAN_POINT('Ctrl Pts',(-2.88559036993739,0.0200923283589629,
1.16731319905181));
#20221=CARTESIAN_POINT('Ctrl Pts',(-2.89349138284601,0.0205972730886243,
1.15311091289949));
#20222=CARTESIAN_POINT('Ctrl Pts',(-2.89801951662537,0.0217263036549144,
1.13650101054829));
#20223=CARTESIAN_POINT('Ctrl Pts',(-2.89832153725836,0.0236238550069256,
1.11979041032883));
#20224=CARTESIAN_POINT('Ctrl Pts',(-2.87292353761376,0.0620480419794871,
1.15999999999999));
#20225=CARTESIAN_POINT('Ctrl Pts',(-2.87941161142243,0.0621984441063758,
1.1487678034684));
#20226=CARTESIAN_POINT('Ctrl Pts',(-2.88316790462212,0.0631932819332653,
1.13573901604496));
#20227=CARTESIAN_POINT('Ctrl Pts',(-2.8836123610279,0.0652969522995559,
1.1226636989343));
#20228=CARTESIAN_POINT('Ctrl Pts',(-2.87292353761376,0.08,1.15999999999999));
#20229=CARTESIAN_POINT('Ctrl Pts',(-2.87920838230231,0.0800000000000008,
1.14911432968172));
#20230=CARTESIAN_POINT('Ctrl Pts',(-2.88286931365848,0.0809374356795997,
1.13672577722824));
#20231=CARTESIAN_POINT('Ctrl Pts',(-2.88353005387198,0.0831281904378377,
1.12422135153951));
#20232=CARTESIAN_POINT('',(-2.87292353761376,0.08,1.15999999999998));
#20233=CARTESIAN_POINT('Ctrl Pts',(-2.88353005387198,0.0831281904378377,
1.12422135153951));
#20234=CARTESIAN_POINT('Ctrl Pts',(-2.88286931365848,0.0809374356795997,
1.13672577722824));
#20235=CARTESIAN_POINT('Ctrl Pts',(-2.87917379579497,0.0800000000000008,
1.14909623365625));
#20236=CARTESIAN_POINT('Ctrl Pts',(-2.87291508431494,0.08,1.15999514568442));
#20237=CARTESIAN_POINT('',(-2.94220556991652,1.81603863891322E-17,1.19999999999998));
#20238=CARTESIAN_POINT('Origin',(-2.94220556991652,0.08,1.19999999999997));
#20239=CARTESIAN_POINT('Ctrl Pts',(-2.94220556991652,1.38777878078145E-17,
1.19999999999997));
#20240=CARTESIAN_POINT('Ctrl Pts',(-2.95477525929363,7.99204335707293E-16,
1.17610462613062));
#20241=CARTESIAN_POINT('Ctrl Pts',(-2.96209712200597,0.00102889281907461,
1.14891024269609));
#20242=CARTESIAN_POINT('Ctrl Pts',(-2.96341860243295,0.00343337974884619,
1.1214615033794));
#20243=CARTESIAN_POINT('Ctrl Pts',(-2.97150840951392,0.0370763918196141,
0.944338414217263));
#20244=CARTESIAN_POINT('Ctrl Pts',(-2.9722976916079,0.0423262056041848,
0.926618942442153));
#20245=CARTESIAN_POINT('Ctrl Pts',(-2.9704006751309,0.0481782537629969,
0.908937053039817));
#20246=CARTESIAN_POINT('Ctrl Pts',(-2.96590341962731,0.0542766412925386,
0.892181871007293));
#20247=CARTESIAN_POINT('Ctrl Pts',(-2.94780986478466,0.0373919537646065,
0.943273311490377));
#20248=CARTESIAN_POINT('Ctrl Pts',(-2.94857578158365,0.0419549531652315,
0.927965726332386));
#20249=CARTESIAN_POINT('Ctrl Pts',(-2.9469952950528,0.0469737957410308,
0.912624042243611));
#20250=CARTESIAN_POINT('Ctrl Pts',(-2.94308190554019,0.0521158688929946,
0.89811854438363));
#20251=CARTESIAN_POINT('Ctrl Pts',(-2.90676705829981,0.056843651940239,
0.947029801368067));
#20252=CARTESIAN_POINT('Ctrl Pts',(-2.90748135565274,0.059940306716287,
0.936220750290145));
#20253=CARTESIAN_POINT('Ctrl Pts',(-2.90645413242085,0.0633115026576812,
0.925322801814758));
#20254=CARTESIAN_POINT('Ctrl Pts',(-2.90355489767837,0.0668278028163856,
0.915117754801607));
#20255=CARTESIAN_POINT('Ctrl Pts',(-2.89185038918151,0.0967186642359907,
0.95811446019075));
#20256=CARTESIAN_POINT('Ctrl Pts',(-2.89236030863334,0.0988989884558824,
0.949564065008555));
#20257=CARTESIAN_POINT('Ctrl Pts',(-2.89145639520232,0.101358036048963,
0.940957760954761));
#20258=CARTESIAN_POINT('Ctrl Pts',(-2.88910171978587,0.104230462691718,
0.932989060257172));
#20259=CARTESIAN_POINT('Ctrl Pts',(-2.89160384339595,0.11378071272758,0.963157443386126));
#20260=CARTESIAN_POINT('Ctrl Pts',(-2.89200506610289,0.115786605025646,
0.954950614685553));
#20261=CARTESIAN_POINT('Ctrl Pts',(-2.89106334819291,0.118074599969182,
0.946756646504643));
#20262=CARTESIAN_POINT('Ctrl Pts',(-2.88881405854803,0.120889693311755,
0.939137268222128));
#20263=CARTESIAN_POINT('',(-2.9659034196274,0.0542766412925467,0.892181871007271));
#20264=CARTESIAN_POINT('',(-2.88881405854801,0.120889693312663,0.939137268222463));
#20265=CARTESIAN_POINT('Origin',(-2.96590341962731,0.129452050955424,0.919543482473312));
#20266=CARTESIAN_POINT('Ctrl Pts',(-2.88881405854803,0.120889693311755,
0.939137268222128));
#20267=CARTESIAN_POINT('Ctrl Pts',(-2.89106334819291,0.118074599969182,
0.946756646504643));
#20268=CARTESIAN_POINT('Ctrl Pts',(-2.89200506610289,0.115786605025646,
0.954950614685553));
#20269=CARTESIAN_POINT('Ctrl Pts',(-2.89160384339595,0.11378071272758,0.963157443386126));
#20270=CARTESIAN_POINT('Ctrl Pts',(-2.97150840951392,0.0370763918196141,
0.944338414217263));
#20271=CARTESIAN_POINT('Ctrl Pts',(-2.9722976916079,0.0423262056041848,
0.926618942442153));
#20272=CARTESIAN_POINT('Ctrl Pts',(-2.9704006751309,0.0481782537629969,
0.908937053039817));
#20273=CARTESIAN_POINT('Ctrl Pts',(-2.96590341962731,0.0542766412925386,
0.892181871007293));
#20274=CARTESIAN_POINT('Ctrl Pts',(-2.803641505311,0.,1.28));
#20275=CARTESIAN_POINT('Ctrl Pts',(-2.83156585186791,0.,1.28));
#20276=CARTESIAN_POINT('Ctrl Pts',(-2.8873697166731,0.,1.26501863102788));
#20277=CARTESIAN_POINT('Ctrl Pts',(-2.92824339663807,0.,1.22418319350235));
#20278=CARTESIAN_POINT('Ctrl Pts',(-2.94220556991652,0.,1.19999999999998));
#20279=CARTESIAN_POINT('Ctrl Pts',(-2.803641505311,0.,1.25606405597265));
#20280=CARTESIAN_POINT('Ctrl Pts',(-2.82737027930954,0.,1.25606405597265));
#20281=CARTESIAN_POINT('Ctrl Pts',(-2.87483488599671,1.25420474925568E-17,
1.24330810087636));
#20282=CARTESIAN_POINT('Ctrl Pts',(-2.90961204732599,-6.04209133589596E-17,
1.20858174906972));
#20283=CARTESIAN_POINT('Ctrl Pts',(-2.92147643432527,-4.86342276316735E-17,
1.1880320279863));
#20284=CARTESIAN_POINT('Ctrl Pts',(-2.803641505311,0.0200923513320623,1.21462642566814));
#20285=CARTESIAN_POINT('Ctrl Pts',(-2.8201635207438,0.0200923513320623,
1.21462642566814));
#20286=CARTESIAN_POINT('Ctrl Pts',(-2.85316323302638,0.0200923513320623,
1.20577244147847));
#20287=CARTESIAN_POINT('Ctrl Pts',(-2.87732938609252,0.0200923513320622,
1.18162169792061));
#20288=CARTESIAN_POINT('Ctrl Pts',(-2.88559039380893,0.0200923513320622,
1.16731321283406));
#20289=CARTESIAN_POINT('Ctrl Pts',(-2.803641505311,0.0620480419794869,1.2));
#20290=CARTESIAN_POINT('Ctrl Pts',(-2.81759233090944,0.0620480419794869,
1.2));
#20291=CARTESIAN_POINT('Ctrl Pts',(-2.84549989357585,0.0620480419794869,
1.19249941381066));
#20292=CARTESIAN_POINT('Ctrl Pts',(-2.86594812481452,0.0620480419794869,
1.17208176937204));
#20293=CARTESIAN_POINT('Ctrl Pts',(-2.87292353761376,0.0620480419794869,
1.15999999999999));
#20294=CARTESIAN_POINT('Ctrl Pts',(-2.803641505311,0.08,1.2));
#20295=CARTESIAN_POINT('Ctrl Pts',(-2.81760367858943,0.08,1.2));
#20296=CARTESIAN_POINT('Ctrl Pts',(-2.84550561099204,0.08,1.19250931551394));
#20297=CARTESIAN_POINT('Ctrl Pts',(-2.86594245097452,0.08,1.17209159675119));
#20298=CARTESIAN_POINT('Ctrl Pts',(-2.87292353761376,0.08,1.15999999999999));
#20299=CARTESIAN_POINT('Ctrl Pts',(-2.87292353215132,0.08,1.1600000094612));
#20300=CARTESIAN_POINT('Ctrl Pts',(-2.86594244564417,0.08,1.17209160207655));
#20301=CARTESIAN_POINT('Ctrl Pts',(-2.84550560735334,0.08,1.1925093164908));
#20302=CARTESIAN_POINT('Ctrl Pts',(-2.81760367858943,0.08,1.2));
#20303=CARTESIAN_POINT('Ctrl Pts',(-2.803641505311,0.08,1.2));
#20304=CARTESIAN_POINT('Ctrl Pts',(-2.803641505311,0.,1.28));
#20305=CARTESIAN_POINT('Ctrl Pts',(-2.83156585186791,0.,1.28));
#20306=CARTESIAN_POINT('Ctrl Pts',(-2.8873697166731,0.,1.26501863102788));
#20307=CARTESIAN_POINT('Ctrl Pts',(-2.92824339663807,0.,1.22418319350235));
#20308=CARTESIAN_POINT('Ctrl Pts',(-2.94220556991652,0.,1.19999999999998));
#20309=CARTESIAN_POINT('Ctrl Pts',(-2.87936339380758,0.129452051231406,
0.919543482573353));
#20310=CARTESIAN_POINT('Ctrl Pts',(-2.88146283528349,0.12700291504183,0.922197454617062));
#20311=CARTESIAN_POINT('Ctrl Pts',(-2.88513307556505,0.12490800002558,0.928743709056956));
#20312=CARTESIAN_POINT('Ctrl Pts',(-2.88777400865552,0.122191365716222,
0.935614140915412));
#20313=CARTESIAN_POINT('Ctrl Pts',(-2.88881405885504,0.120889693194046,
0.939137269378581));
#20314=CARTESIAN_POINT('Ctrl Pts',(-2.87936339372816,0.106959621146319,
0.911356907579326));
#20315=CARTESIAN_POINT('Ctrl Pts',(-2.88181984292263,0.104843095498008,
0.91387702531295));
#20316=CARTESIAN_POINT('Ctrl Pts',(-2.88543932888245,0.102667578804832,
0.920501736474717));
#20317=CARTESIAN_POINT('Ctrl Pts',(-2.88815026196516,0.0999776780681394,
0.927409871210725));
#20318=CARTESIAN_POINT('Ctrl Pts',(-2.88919760708753,0.0986773855985862,
0.930939658748897));
#20319=CARTESIAN_POINT('Ctrl Pts',(-2.89636159093292,0.0716838001108839,
0.8871184305754));
#20320=CARTESIAN_POINT('Ctrl Pts',(-2.89953989153624,0.0700649159705931,
0.890573780537225));
#20321=CARTESIAN_POINT('Ctrl Pts',(-2.90406236399545,0.0671359894824263,
0.898820413092617));
#20322=CARTESIAN_POINT('Ctrl Pts',(-2.90746777995082,0.0639291528782548,
0.907488124439835));
#20323=CARTESIAN_POINT('Ctrl Pts',(-2.90878614712001,0.0623073044369298,
0.911931323621345));
#20324=CARTESIAN_POINT('Ctrl Pts',(-2.93185794276191,0.0655906976416168,
0.861096582782205));
#20325=CARTESIAN_POINT('Ctrl Pts',(-2.93571995395406,0.0636246040882168,
0.866508892071219));
#20326=CARTESIAN_POINT('Ctrl Pts',(-2.94222111396444,0.0594240163271901,
0.87804374409531));
#20327=CARTESIAN_POINT('Ctrl Pts',(-2.94693586861888,0.0549402807148656,
0.890358235333227));
#20328=CARTESIAN_POINT('Ctrl Pts',(-2.94878744727228,0.0526560220635993,
0.896634315718971));
#20329=CARTESIAN_POINT('Ctrl Pts',(-2.94704588059102,0.0688641988014324,
0.852102886147849));
#20330=CARTESIAN_POINT('Ctrl Pts',(-2.95120132743568,0.0666088423893841,
0.858299426813201));
#20331=CARTESIAN_POINT('Ctrl Pts',(-2.95854860928908,0.0618941129944658,
0.871253039452356));
#20332=CARTESIAN_POINT('Ctrl Pts',(-2.96382417230887,0.0568458522077424,
0.885123022035033));
#20333=CARTESIAN_POINT('Ctrl Pts',(-2.965903663846,0.0542766635868824,0.892181809755297));
#20334=CARTESIAN_POINT('',(-2.96041704457315,0.0598643409482463,0.876829792382116));
#20335=CARTESIAN_POINT('',(-2.87936339380758,0.129452050955555,0.919543482472952));
#20336=CARTESIAN_POINT('Ctrl Pts',(-2.96041669789433,0.0598642771869273,
0.876829967575949));
#20337=CARTESIAN_POINT('Ctrl Pts',(-2.96041641286921,0.0598644584628993,
0.876829469535466));
#20338=CARTESIAN_POINT('Ctrl Pts',(-2.96041607078052,0.0598646469725351,
0.87682895162779));
#20339=CARTESIAN_POINT('Ctrl Pts',(-2.96041508469685,0.0598650593064606,
0.876827818832396));
#20340=CARTESIAN_POINT('Ctrl Pts',(-2.96041443818893,0.0598652486069508,
0.876827298805383));
#20341=CARTESIAN_POINT('Ctrl Pts',(-2.96041272590323,0.0598655661020481,
0.876826426772454));
#20342=CARTESIAN_POINT('Ctrl Pts',(-2.96041160620732,0.0598656765852475,
0.87682612344575));
#20343=CARTESIAN_POINT('Ctrl Pts',(-2.96040815324349,0.0598658185101067,
0.876825734520681));
#20344=CARTESIAN_POINT('Ctrl Pts',(-2.96040556214768,0.0598657920045578,
0.876825808324795));
#20345=CARTESIAN_POINT('Ctrl Pts',(-2.96039837346811,0.0598655893040655,
0.876826369399628));
#20346=CARTESIAN_POINT('Ctrl Pts',(-2.9603929165739,0.0598653472112175,
0.876827038754178));
#20347=CARTESIAN_POINT('Ctrl Pts',(-2.96037760633566,0.0598646053374691,
0.876829094693984));
#20348=CARTESIAN_POINT('Ctrl Pts',(-2.96036380015299,0.0598638705770211,
0.876831138211164));
#20349=CARTESIAN_POINT('Ctrl Pts',(-2.96033719264881,0.0598624486708876,
0.876835106182144));
#20350=CARTESIAN_POINT('Ctrl Pts',(-2.96031159368107,0.0598610583320029,
0.87683901584924));
#20351=CARTESIAN_POINT('Ctrl Pts',(-2.96025529525252,0.0598580144693806,
0.876847638168764));
#20352=CARTESIAN_POINT('Ctrl Pts',(-2.96021310455862,0.0598557471926268,
0.876854148091574));
#20353=CARTESIAN_POINT('Ctrl Pts',(-2.96008734802608,0.0598490878769054,
0.876873602790802));
#20354=CARTESIAN_POINT('Ctrl Pts',(-2.96000449353606,0.0598448127019288,
0.876886490315284));
#20355=CARTESIAN_POINT('Ctrl Pts',(-2.95975590153061,0.0598323488694641,
0.876925311717692));
#20356=CARTESIAN_POINT('Ctrl Pts',(-2.95959033691541,0.0598245243488887,
0.876951380460641));
#20357=CARTESIAN_POINT('Ctrl Pts',(-2.95909365784188,0.0598024889557596,
0.877030194875114));
#20358=CARTESIAN_POINT('Ctrl Pts',(-2.95876256633421,0.0597897148429793,
0.87708355225251));
#20359=CARTESIAN_POINT('Ctrl Pts',(-2.95776929650042,0.0597571183908872,
0.877246060040826));
#20360=CARTESIAN_POINT('Ctrl Pts',(-2.9571073199902,0.0597430321504992,
0.877357618292709));
#20361=CARTESIAN_POINT('Ctrl Pts',(-2.95512198401899,0.0597235213942096,
0.877701903024172));
#20362=CARTESIAN_POINT('Ctrl Pts',(-2.95380002536389,0.0597408898589351,
0.877944117676307));
#20363=CARTESIAN_POINT('Ctrl Pts',(-2.94984178410647,0.0598827452244851,
0.878707993952471));
#20364=CARTESIAN_POINT('Ctrl Pts',(-2.94721536727803,0.0600971459470857,
0.879266580845324));
#20365=CARTESIAN_POINT('Ctrl Pts',(-2.93941233445455,0.0610887194259119,
0.881080123930645));
#20366=CARTESIAN_POINT('Ctrl Pts',(-2.93430536722629,0.0622152948597964,
0.882474905957679));
#20367=CARTESIAN_POINT('Ctrl Pts',(-2.92116902241244,0.0664103649549747,
0.886626951401218));
#20368=CARTESIAN_POINT('Ctrl Pts',(-2.91200301339737,0.0707140517326124,
0.890125580532118));
#20369=CARTESIAN_POINT('Ctrl Pts',(-2.8961467184212,0.0842530156264676,
0.898723641095627));
#20370=CARTESIAN_POINT('Ctrl Pts',(-2.89019671334679,0.0919560410529159,
0.90303400223478));
#20371=CARTESIAN_POINT('Ctrl Pts',(-2.88388864657462,0.105006472772146,
0.909426649433165));
#20372=CARTESIAN_POINT('Ctrl Pts',(-2.8822163987365,0.109700228982129,0.911582109267249));
#20373=CARTESIAN_POINT('Ctrl Pts',(-2.87995399962771,0.119400639997362,
0.915722468197169));
#20374=CARTESIAN_POINT('Ctrl Pts',(-2.87936339380758,0.124392439973975,
0.917701934678691));
#20375=CARTESIAN_POINT('Ctrl Pts',(-2.87936339380758,0.129452050955555,
0.919543482472953));
#20376=CARTESIAN_POINT('Ctrl Pts',(-2.87936339380758,0.129452050955555,
0.919543482472952));
#20377=CARTESIAN_POINT('Ctrl Pts',(-2.88146283528787,0.127002914770058,
0.922197454515019));
#20378=CARTESIAN_POINT('Ctrl Pts',(-2.88513307538547,0.124907999857464,
0.928743708628879));
#20379=CARTESIAN_POINT('Ctrl Pts',(-2.8877740083963,0.12219136571519,0.935614140128415));
#20380=CARTESIAN_POINT('Ctrl Pts',(-2.88881405854803,0.120889693311755,
0.939137268222128));
#20381=CARTESIAN_POINT('Origin',(-2.81154186539738,0.0396551669818869,0.932354041514756));
#20382=CARTESIAN_POINT('Ctrl Pts',(-2.87936339380758,-3.,1.2));
#20383=CARTESIAN_POINT('Ctrl Pts',(-2.87936339380758,4.2,1.2));
#20384=CARTESIAN_POINT('Ctrl Pts',(-2.88050601962387,-3.,1.18008118002045));
#20385=CARTESIAN_POINT('Ctrl Pts',(-2.88050601962387,4.2,1.18008118002045));
#20386=CARTESIAN_POINT('Ctrl Pts',(-2.88410012960011,-3.,1.11550336602625));
#20387=CARTESIAN_POINT('Ctrl Pts',(-2.88410012960011,4.2,1.11550336602625));
#20388=CARTESIAN_POINT('Ctrl Pts',(-2.88965455295869,-3.,1.00596877194195));
#20389=CARTESIAN_POINT('Ctrl Pts',(-2.88965455295869,4.2,1.00596877194195));
#20390=CARTESIAN_POINT('Ctrl Pts',(-2.89676647174981,-3.,0.851337038635417));
#20391=CARTESIAN_POINT('Ctrl Pts',(-2.89676647174981,4.2,0.851337038635417));
#20392=CARTESIAN_POINT('Ctrl Pts',(-2.90717911786707,-3.,0.654020230869684));
#20393=CARTESIAN_POINT('Ctrl Pts',(-2.90717911786707,4.2,0.654020230869684));
#20394=CARTESIAN_POINT('Ctrl Pts',(-2.92780415844476,-3.,0.444963858672577));
#20395=CARTESIAN_POINT('Ctrl Pts',(-2.92780415844476,4.2,0.444963858672577));
#20396=CARTESIAN_POINT('Ctrl Pts',(-2.96639254265869,-3.,0.262319630540737));
#20397=CARTESIAN_POINT('Ctrl Pts',(-2.96639254265869,4.2,0.262319630540737));
#20398=CARTESIAN_POINT('Ctrl Pts',(-3.03063129752067,-3.,0.11901737132707));
#20399=CARTESIAN_POINT('Ctrl Pts',(-3.03063129752067,4.2,0.11901737132707));
#20400=CARTESIAN_POINT('Ctrl Pts',(-3.12452733970658,-3.,0.0241851999813871));
#20401=CARTESIAN_POINT('Ctrl Pts',(-3.12452733970658,4.2,0.0241851999813871));
#20402=CARTESIAN_POINT('Ctrl Pts',(-3.24511001026157,-3.,-0.0214179570895714));
#20403=CARTESIAN_POINT('Ctrl Pts',(-3.24511001026157,4.2,-0.0214179570895714));
#20404=CARTESIAN_POINT('Ctrl Pts',(-3.38164698943802,-3.,-0.0263068037112043));
#20405=CARTESIAN_POINT('Ctrl Pts',(-3.38164698943802,4.2,-0.0263068037112043));
#20406=CARTESIAN_POINT('Ctrl Pts',(-3.52045328348989,-3.,-0.00118366394785932));
#20407=CARTESIAN_POINT('Ctrl Pts',(-3.52045328348989,4.2,-0.00118366394785932));
#20408=CARTESIAN_POINT('Ctrl Pts',(-3.64881642260079,-3.,0.0470540298718583));
#20409=CARTESIAN_POINT('Ctrl Pts',(-3.64881642260079,4.2,0.0470540298718583));
#20410=CARTESIAN_POINT('Ctrl Pts',(-3.75872318140663,-3.,0.120497232333251));
#20411=CARTESIAN_POINT('Ctrl Pts',(-3.75872318140663,4.2,0.120497232333251));
#20412=CARTESIAN_POINT('Ctrl Pts',(-3.84598208672296,-3.,0.224659532804408));
#20413=CARTESIAN_POINT('Ctrl Pts',(-3.84598208672296,4.2,0.224659532804408));
#20414=CARTESIAN_POINT('Ctrl Pts',(-3.9098657241983,-3.,0.364350357241515));
#20415=CARTESIAN_POINT('Ctrl Pts',(-3.9098657241983,4.2,0.364350357241515));
#20416=CARTESIAN_POINT('Ctrl Pts',(-3.9525920016999,-3.,0.538436816836325));
#20417=CARTESIAN_POINT('Ctrl Pts',(-3.9525920016999,4.2,0.538436816836325));
#20418=CARTESIAN_POINT('Ctrl Pts',(-3.97841403016126,-3.,0.741129277895169));
#20419=CARTESIAN_POINT('Ctrl Pts',(-3.97841403016126,4.2,0.741129277895169));
#20420=CARTESIAN_POINT('Ctrl Pts',(-3.98977740850458,-3.,0.919671129654853));
#20421=CARTESIAN_POINT('Ctrl Pts',(-3.98977740850458,4.2,0.919671129654853));
#20422=CARTESIAN_POINT('Ctrl Pts',(-3.99545186687387,-3.,1.05866205464795));
#20423=CARTESIAN_POINT('Ctrl Pts',(-3.99545186687387,4.2,1.05866205464795));
#20424=CARTESIAN_POINT('Ctrl Pts',(-3.99855414331415,-3.,1.15256872586734));
#20425=CARTESIAN_POINT('Ctrl Pts',(-3.99855414331415,4.2,1.15256872586734));
#20426=CARTESIAN_POINT('Ctrl Pts',(-3.99999413894399,-3.,1.19980766336825));
#20427=CARTESIAN_POINT('Ctrl Pts',(-3.99999413894399,4.2,1.19980766336825));
#20428=CARTESIAN_POINT('Ctrl Pts',(-4.,-3.,1.2));
#20429=CARTESIAN_POINT('Ctrl Pts',(-4.,4.2,1.2));
#20430=CARTESIAN_POINT('',(-2.89158569656657,0.11486454003439,0.963528635709791));
#20431=CARTESIAN_POINT('Origin',(-2.89391657159917,0.129178635160739,0.915904052326592));
#20432=CARTESIAN_POINT('',(-2.8852657140673,0.5,1.09088035845137));
#20433=CARTESIAN_POINT('Ctrl Pts',(-2.8852657140673,0.5,1.09088035845137));
#20434=CARTESIAN_POINT('Ctrl Pts',(-2.88739518236194,0.371284826357953,
1.04939286925411));
#20435=CARTESIAN_POINT('Ctrl Pts',(-2.88948025018409,0.243010859025609,
1.00659623192935));
#20436=CARTESIAN_POINT('Ctrl Pts',(-2.89158569656657,0.114864540034388,
0.963528635709792));
#20437=CARTESIAN_POINT('',(-2.88353005387197,0.5,1.12422135153951));
#20438=CARTESIAN_POINT('Ctrl Pts',(-2.88353005387198,0.500000000000001,
1.12422135153951));
#20439=CARTESIAN_POINT('Ctrl Pts',(-2.88378350828653,0.500000000000001,
1.11942475852518));
#20440=CARTESIAN_POINT('Ctrl Pts',(-2.88413377322526,0.500000000000001,
1.11275818755601));
#20441=CARTESIAN_POINT('Ctrl Pts',(-2.88448145181725,0.500000000000001,
1.10609021938137));
#20442=CARTESIAN_POINT('Ctrl Pts',(-2.88482670797398,0.500000000000001,
1.09942100077238));
#20443=CARTESIAN_POINT('Ctrl Pts',(-2.885169713669,0.500000000000001,1.09275069176305));
#20444=CARTESIAN_POINT('Ctrl Pts',(-2.8852657140673,0.500000000000001,1.09088035845137));
#20445=CARTESIAN_POINT('',(-2.88353005387198,0.0831281904378376,1.12422135153951));
#20446=CARTESIAN_POINT('Ctrl Pts',(-2.87936280293809,0.129463942239828,
0.919546811122371));
#20447=CARTESIAN_POINT('Ctrl Pts',(-2.87936272551578,0.128996507120314,
0.919376678242473));
#20448=CARTESIAN_POINT('Ctrl Pts',(-2.87936729845633,0.128528665510741,
0.919206397636387));
#20449=CARTESIAN_POINT('Ctrl Pts',(-2.87937652870275,0.128060914565431,
0.919036150256641));
#20450=CARTESIAN_POINT('Ctrl Pts',(-2.88800912722877,0.125219614594593,
0.932602973731212));
#20451=CARTESIAN_POINT('Ctrl Pts',(-2.8880161408965,0.124635052899647,0.932396199243668));
#20452=CARTESIAN_POINT('Ctrl Pts',(-2.88802498402021,0.124050831955124,
0.932186275174002));
#20453=CARTESIAN_POINT('Ctrl Pts',(-2.88803574670127,0.123468016182681,
0.931973542850541));
#20454=CARTESIAN_POINT('Ctrl Pts',(-2.8923362255842,0.120058692271535,0.948176288112179));
#20455=CARTESIAN_POINT('Ctrl Pts',(-2.89234848804188,0.119330898552523,
0.947926692856932));
#20456=CARTESIAN_POINT('Ctrl Pts',(-2.8923610549264,0.118605121800164,0.947669421968552));
#20457=CARTESIAN_POINT('Ctrl Pts',(-2.8923740164996,0.117882286794026,0.94740478025217));
#20458=CARTESIAN_POINT('Ctrl Pts',(-2.89158534139673,0.11488616536118,0.963535900827959));
#20459=CARTESIAN_POINT('Ctrl Pts',(-2.89159964786982,0.114014752657563,
0.963243257015774));
#20460=CARTESIAN_POINT('Ctrl Pts',(-2.89161454709808,0.113147190385347,
0.962938501079936));
#20461=CARTESIAN_POINT('Ctrl Pts',(-2.89163003027391,0.1122839746201,0.962621817739011));
#20462=CARTESIAN_POINT('Origin',(-2.81168112317661,0.114864540034389,0.959622339334904));
#20463=CARTESIAN_POINT('Ctrl Pts',(-3.99945760881125,0.13546233783637,0.903030354983468));
#20464=CARTESIAN_POINT('Ctrl Pts',(-3.9973961162676,0.158008411859628,0.841085525707216));
#20465=CARTESIAN_POINT('Ctrl Pts',(-3.99279290514081,0.203310563544645,
0.716618886899923));
#20466=CARTESIAN_POINT('Ctrl Pts',(-3.97849395981051,0.281987502029712,
0.50045577498038));
#20467=CARTESIAN_POINT('Ctrl Pts',(-3.95509656322196,0.35087941221533,0.311176807362298));
#20468=CARTESIAN_POINT('Ctrl Pts',(-3.90963080113393,0.40951907607415,0.150065655025781));
#20469=CARTESIAN_POINT('Ctrl Pts',(-3.8691416736774,0.444506704555304,0.0539379358135427));
#20470=CARTESIAN_POINT('Ctrl Pts',(-3.80820163959337,0.478469777977808,
-0.0393748415100655));
#20471=CARTESIAN_POINT('Ctrl Pts',(-3.72122359734069,0.507285738389506,
-0.118546042061105));
#20472=CARTESIAN_POINT('Ctrl Pts',(-3.58603043474247,0.533328259831995,
-0.190097281670006));
#20473=CARTESIAN_POINT('Ctrl Pts',(-3.44370085318666,0.546103828098339,
-0.225197867002487));
#20474=CARTESIAN_POINT('Ctrl Pts',(-3.29162344210726,0.547685564166839,
-0.229543651134227));
#20475=CARTESIAN_POINT('Ctrl Pts',(-3.18823564478345,0.539575598601234,
-0.207261703870172));
#20476=CARTESIAN_POINT('Ctrl Pts',(-3.11077137978012,0.523493646274472,
-0.163076902991648));
#20477=CARTESIAN_POINT('Ctrl Pts',(-3.04751283334051,0.502320173155856,
-0.104903263706821));
#20478=CARTESIAN_POINT('Ctrl Pts',(-2.97789574195055,0.460397612655845,
0.0102780246326795));
#20479=CARTESIAN_POINT('Ctrl Pts',(-2.91982931246599,0.377551236111436,
0.237896573472077));
#20480=CARTESIAN_POINT('Ctrl Pts',(-2.89832305986079,0.263668991805047,
0.550785468180695));
#20481=CARTESIAN_POINT('Ctrl Pts',(-2.88684765097271,0.174075173876031,
0.796942459863397));
#20482=CARTESIAN_POINT('Ctrl Pts',(-2.87936339380758,0.129452050955555,
0.919543482472953));
#20483=CARTESIAN_POINT('Ctrl Pts',(-3.99945760881125,0.112969907862324,
0.894843779976599));
#20484=CARTESIAN_POINT('Ctrl Pts',(-3.99739609096167,0.13551625865078,0.832898190294214));
#20485=CARTESIAN_POINT('Ctrl Pts',(-3.9927943517283,0.180816769376243,0.708436059986241));
#20486=CARTESIAN_POINT('Ctrl Pts',(-3.97850103889804,0.259491261707806,
0.492279668818216));
#20487=CARTESIAN_POINT('Ctrl Pts',(-3.95511811012035,0.328375650295247,
0.303021366621285));
#20488=CARTESIAN_POINT('Ctrl Pts',(-3.90966176168135,0.387018886385186,
0.141900399660432));
#20489=CARTESIAN_POINT('Ctrl Pts',(-3.8691813956086,0.422008258304128,0.0457678903922369));
#20490=CARTESIAN_POINT('Ctrl Pts',(-3.80822946486193,0.455982725304131,
-0.0475761905282765));
#20491=CARTESIAN_POINT('Ctrl Pts',(-3.72124990150233,0.484803780244265,
-0.126761388181157));
#20492=CARTESIAN_POINT('Ctrl Pts',(-3.58604191832488,0.510849567633407,
-0.198321600904739));
#20493=CARTESIAN_POINT('Ctrl Pts',(-3.44375381289202,0.523625721203665,
-0.233423794346508));
#20494=CARTESIAN_POINT('Ctrl Pts',(-3.29167170986371,0.525210387234294,
-0.237777628483038));
#20495=CARTESIAN_POINT('Ctrl Pts',(-3.18824858312854,0.517100692154883,
-0.215496424373695));
#20496=CARTESIAN_POINT('Ctrl Pts',(-3.11073783195475,0.501008107849723,
-0.171282412374599));
#20497=CARTESIAN_POINT('Ctrl Pts',(-3.04744355689428,0.479821356105204,
-0.11307229036494));
#20498=CARTESIAN_POINT('Ctrl Pts',(-2.97782462588385,0.437884988863251,
0.00214693168628145));
#20499=CARTESIAN_POINT('Ctrl Pts',(-2.91980546068163,0.355046369978444,
0.229744166531096));
#20500=CARTESIAN_POINT('Ctrl Pts',(-2.89831668227606,0.241171500824311,
0.542612798175426));
#20501=CARTESIAN_POINT('Ctrl Pts',(-2.88684752017467,0.151581964049483,
0.788758027483666));
#20502=CARTESIAN_POINT('Ctrl Pts',(-2.87936339380758,0.106959620981509,
0.911356907466083));
#20503=CARTESIAN_POINT('Ctrl Pts',(-3.97937276807867,0.0738190510046144,
0.881262446761113));
#20504=CARTESIAN_POINT('Ctrl Pts',(-3.97731327142506,0.0963432964334023,
0.819377591055264));
#20505=CARTESIAN_POINT('Ctrl Pts',(-3.97270726831941,0.141579135382642,
0.695093144992142));
#20506=CARTESIAN_POINT('Ctrl Pts',(-3.95848366570773,0.219966739110569,
0.479724973784506));
#20507=CARTESIAN_POINT('Ctrl Pts',(-3.93516955254869,0.288360740578814,
0.291813999124357));
#20508=CARTESIAN_POINT('Ctrl Pts',(-3.89045398807751,0.34598040353968,0.133505276222791));
#20509=CARTESIAN_POINT('Ctrl Pts',(-3.85097180237235,0.380059347708762,
0.0398741466393852));
#20510=CARTESIAN_POINT('Ctrl Pts',(-3.79225425972909,0.412734983723264,
-0.0499014254767779));
#20511=CARTESIAN_POINT('Ctrl Pts',(-3.70917100058941,0.440255377838933,
-0.125513086884069));
#20512=CARTESIAN_POINT('Ctrl Pts',(-3.57908941427417,0.465363375357826,
-0.194496743114952));
#20513=CARTESIAN_POINT('Ctrl Pts',(-3.44018820684967,0.477851863444749,
-0.2288085821369));
#20514=CARTESIAN_POINT('Ctrl Pts',(-3.29321826238141,0.479328003623049,
-0.232864243944729));
#20515=CARTESIAN_POINT('Ctrl Pts',(-3.19543503576692,0.471597152685915,
-0.211623905561783));
#20516=CARTESIAN_POINT('Ctrl Pts',(-3.12325058435565,0.456594508464948,
-0.170404479332566));
#20517=CARTESIAN_POINT('Ctrl Pts',(-3.06397256609718,0.436789352841401,
-0.115990261468086));
#20518=CARTESIAN_POINT('Ctrl Pts',(-2.99722044260985,0.396760213362037,
-0.00601110462833348));
#20519=CARTESIAN_POINT('Ctrl Pts',(-2.9398515643179,0.315401605007014,0.217519834705343));
#20520=CARTESIAN_POINT('Ctrl Pts',(-2.91841241808079,0.201953714096476,
0.529215353266799));
#20521=CARTESIAN_POINT('Ctrl Pts',(-2.90691964577141,0.112314614371736,
0.775496755660762));
#20522=CARTESIAN_POINT('Ctrl Pts',(-2.8994250725072,0.0676299841370301,
0.898266768227296));
#20523=CARTESIAN_POINT('Ctrl Pts',(-3.93743988512382,0.0596235975755129,
0.87749122935701));
#20524=CARTESIAN_POINT('Ctrl Pts',(-3.93538453772238,0.0821024635791913,
0.815731052596958));
#20525=CARTESIAN_POINT('Ctrl Pts',(-3.93077373753047,0.127198705107589,
0.691830147295415));
#20526=CARTESIAN_POINT('Ctrl Pts',(-3.9167113835724,0.20498052425003,0.478126355557454));
#20527=CARTESIAN_POINT('Ctrl Pts',(-3.89358129219178,0.272329724497136,
0.293085948660201));
#20528=CARTESIAN_POINT('Ctrl Pts',(-3.8504385811501,0.327822346713796,0.140621222173602));
#20529=CARTESIAN_POINT('Ctrl Pts',(-3.81306481879868,0.360005373332597,
0.0521990832487384));
#20530=CARTESIAN_POINT('Ctrl Pts',(-3.75897902541619,0.390001101649611,
-0.0302135029823513));
#20531=CARTESIAN_POINT('Ctrl Pts',(-3.68402617998296,0.414820200291004,
-0.0984034160707962));
#20532=CARTESIAN_POINT('Ctrl Pts',(-3.56460608864264,0.4379794000974,-0.162032794591505));
#20533=CARTESIAN_POINT('Ctrl Pts',(-3.43289167818615,0.449868936091557,
-0.194699026263248));
#20534=CARTESIAN_POINT('Ctrl Pts',(-3.29658174994825,0.451126668724512,
-0.198154618272002));
#20535=CARTESIAN_POINT('Ctrl Pts',(-3.21047490685931,0.44418751827955,-0.179089459114268));
#20536=CARTESIAN_POINT('Ctrl Pts',(-3.14928099284796,0.431430785935711,
-0.144040625053544));
#20537=CARTESIAN_POINT('Ctrl Pts',(-3.09828842224605,0.414473076814942,
-0.0974497021585525));
#20538=CARTESIAN_POINT('Ctrl Pts',(-3.03751645364449,0.378387318235333,
0.0016951047028135));
#20539=CARTESIAN_POINT('Ctrl Pts',(-2.98163705203391,0.300140293015244,
0.216677039634506));
#20540=CARTESIAN_POINT('Ctrl Pts',(-2.96035026114277,0.187604410632771,
0.52586683535875));
#20541=CARTESIAN_POINT('Ctrl Pts',(-2.94882561743878,0.097873773732583,
0.772399734075299));
#20542=CARTESIAN_POINT('Ctrl Pts',(-2.94130959805507,0.0530612760548464,
0.895521059554243));
#20543=CARTESIAN_POINT('Ctrl Pts',(-3.91949669889834,0.0594316804308482,
0.878018517378383));
#20544=CARTESIAN_POINT('Ctrl Pts',(-3.91744312474473,0.0818911528271679,
0.81631162411663));
#20545=CARTESIAN_POINT('Ctrl Pts',(-3.91283040143456,0.12692751581812,0.692575233744628));
#20546=CARTESIAN_POINT('Ctrl Pts',(-3.89883754199609,0.204449902882089,
0.479584225784152));
#20547=CARTESIAN_POINT('Ctrl Pts',(-3.87578746756243,0.271351367948194,
0.295773961186595));
#20548=CARTESIAN_POINT('Ctrl Pts',(-3.83331861312405,0.325934138527799,
0.14580903152786));
#20549=CARTESIAN_POINT('Ctrl Pts',(-3.7968478216781,0.3573060507223,0.0596154111683547));
#20550=CARTESIAN_POINT('Ctrl Pts',(-3.74474291823659,0.386156042733723,
-0.0196492904344777));
#20551=CARTESIAN_POINT('Ctrl Pts',(-3.67326896340584,0.409819698696741,
-0.0846646508546109));
#20552=CARTESIAN_POINT('Ctrl Pts',(-3.55840964799874,0.432145290546818,
-0.146003710338657));
#20553=CARTESIAN_POINT('Ctrl Pts',(-3.4297741371024,0.443778584954816,-0.177965924038501));
#20554=CARTESIAN_POINT('Ctrl Pts',(-3.29802524363671,0.444943118366151,
-0.181165453290342));
#20555=CARTESIAN_POINT('Ctrl Pts',(-3.21691164450761,0.438342762365917,
-0.163031124219339));
#20556=CARTESIAN_POINT('Ctrl Pts',(-3.16041651707056,0.426546125464733,
-0.13062013070783));
#20557=CARTESIAN_POINT('Ctrl Pts',(-3.11296616528858,0.410805676990282,
-0.087373603952188));
#20558=CARTESIAN_POINT('Ctrl Pts',(-3.05475295808673,0.37640608565689,0.00713849647477464));
#20559=CARTESIAN_POINT('Ctrl Pts',(-2.99951506785369,0.299491197583846,
0.218460414675343));
#20560=CARTESIAN_POINT('Ctrl Pts',(-2.97829500840806,0.187346215163306,
0.526576221580912));
#20561=CARTESIAN_POINT('Ctrl Pts',(-2.96675727674276,0.0975767861342948,
0.773215700795454));
#20562=CARTESIAN_POINT('Ctrl Pts',(-2.95923209202432,0.0527096423040758,
0.896487165344404));
#20563=CARTESIAN_POINT('',(-3.91949669889834,0.0594316804308483,0.878018517378383));
#20564=CARTESIAN_POINT('Ctrl Pts',(-2.96041766193066,0.0598644374565791,
0.876829527222077));
#20565=CARTESIAN_POINT('Ctrl Pts',(-2.96737439864014,0.102348383545406,
0.760105844653699));
#20566=CARTESIAN_POINT('Ctrl Pts',(-2.9787461837485,0.189730612377242,0.52002514407661));
#20567=CARTESIAN_POINT('Ctrl Pts',(-2.99951506785369,0.299491197583846,
0.218460414675343));
#20568=CARTESIAN_POINT('Ctrl Pts',(-3.05475295808673,0.37640608565689,0.00713849647477464));
#20569=CARTESIAN_POINT('Ctrl Pts',(-3.11296616528858,0.410805676990282,
-0.087373603952188));
#20570=CARTESIAN_POINT('Ctrl Pts',(-3.16041651707056,0.426546125464733,
-0.13062013070783));
#20571=CARTESIAN_POINT('Ctrl Pts',(-3.21691164450761,0.438342762365917,
-0.163031124219339));
#20572=CARTESIAN_POINT('Ctrl Pts',(-3.29802524363671,0.444943118366151,
-0.181165453290342));
#20573=CARTESIAN_POINT('Ctrl Pts',(-3.4297741371024,0.443778584954816,-0.177965924038501));
#20574=CARTESIAN_POINT('Ctrl Pts',(-3.55840964799874,0.432145290546818,
-0.146003710338657));
#20575=CARTESIAN_POINT('Ctrl Pts',(-3.67326896340584,0.409819698696741,
-0.0846646508546109));
#20576=CARTESIAN_POINT('Ctrl Pts',(-3.74474291823659,0.386156042733723,
-0.0196492904344777));
#20577=CARTESIAN_POINT('Ctrl Pts',(-3.7968478216781,0.3573060507223,0.0596154111683547));
#20578=CARTESIAN_POINT('Ctrl Pts',(-3.83331861312405,0.325934138527799,
0.14580903152786));
#20579=CARTESIAN_POINT('Ctrl Pts',(-3.87578746756243,0.271351367948194,
0.295773961186595));
#20580=CARTESIAN_POINT('Ctrl Pts',(-3.89883754199609,0.204449902882089,
0.479584225784152));
#20581=CARTESIAN_POINT('Ctrl Pts',(-3.91283040143456,0.12692751581812,0.692575233744628));
#20582=CARTESIAN_POINT('Ctrl Pts',(-3.91744312474473,0.0818911528271679,
0.81631162411663));
#20583=CARTESIAN_POINT('Ctrl Pts',(-3.91949669889834,0.0594316804308482,
0.878018517378383));
#20584=CARTESIAN_POINT('',(-3.99945760881125,0.135462337836371,0.903030354983466));
#20585=CARTESIAN_POINT('Origin',(-3.91949669889834,0.134607090093721,0.905380128844436));
#20586=CARTESIAN_POINT('Ctrl Pts',(-3.99945760881125,0.135462337836371,
0.903030354983466));
#20587=CARTESIAN_POINT('Ctrl Pts',(-3.99823410537672,0.148843515996691,
0.866265870142289));
#20588=CARTESIAN_POINT('Ctrl Pts',(-3.99689944434567,0.162259022242162,
0.829407069662303));
#20589=CARTESIAN_POINT('Ctrl Pts',(-3.99536024116589,0.17567461573747,0.792548029465364));
#20590=CARTESIAN_POINT('Ctrl Pts',(-3.99427372087306,0.185144655017843,
0.766529310381191));
#20591=CARTESIAN_POINT('Ctrl Pts',(-3.99308470617941,0.194614511215692,
0.740511094312118));
#20592=CARTESIAN_POINT('Ctrl Pts',(-3.99175212990483,0.204067318082626,
0.714539720894749));
#20593=CARTESIAN_POINT('Ctrl Pts',(-3.99025895344394,0.214659363710641,
0.685438314705947));
#20594=CARTESIAN_POINT('Ctrl Pts',(-3.98858683641064,0.225229808869164,
0.65639625531932));
#20595=CARTESIAN_POINT('Ctrl Pts',(-3.98665248763581,0.235815021378387,
0.6273136229701));
#20596=CARTESIAN_POINT('Ctrl Pts',(-3.98481642208428,0.245862404919968,
0.599708663565006));
#20597=CARTESIAN_POINT('Ctrl Pts',(-3.98274441730402,0.255923265448313,
0.572066676443098));
#20598=CARTESIAN_POINT('Ctrl Pts',(-3.98034174674877,0.266015499867288,
0.544338490265121));
#20599=CARTESIAN_POINT('Ctrl Pts',(-3.97939553288731,0.269989999025906,
0.533418643573175));
#20600=CARTESIAN_POINT('Ctrl Pts',(-3.97839766833391,0.273969348433885,
0.522485470930634));
#20601=CARTESIAN_POINT('Ctrl Pts',(-3.9773423211157,0.277949779679242,0.511549325964324));
#20602=CARTESIAN_POINT('Ctrl Pts',(-3.97510642880281,0.286382848407637,
0.488379660056349));
#20603=CARTESIAN_POINT('Ctrl Pts',(-3.97261253876767,0.294829085588724,
0.465173814121954));
#20604=CARTESIAN_POINT('Ctrl Pts',(-3.96977215365409,0.303312662508484,
0.441865378098708));
#20605=CARTESIAN_POINT('Ctrl Pts',(-3.96702053057532,0.311531127649501,
0.419285330701187));
#20606=CARTESIAN_POINT('Ctrl Pts',(-3.96394406722112,0.319784800447935,
0.396608551059925));
#20607=CARTESIAN_POINT('Ctrl Pts',(-3.96043598303906,0.328081168873384,
0.373814466147526));
#20608=CARTESIAN_POINT('Ctrl Pts',(-3.95703752648768,0.336118275785539,
0.351732696388639));
#20609=CARTESIAN_POINT('Ctrl Pts',(-3.9532343129631,0.344195585556897,0.329540470181892));
#20610=CARTESIAN_POINT('Ctrl Pts',(-3.94889948313842,0.352303921980112,
0.307262998949767));
#20611=CARTESIAN_POINT('Ctrl Pts',(-3.94595348495836,0.357814436882015,
0.292122983687222));
#20612=CARTESIAN_POINT('Ctrl Pts',(-3.94276133969239,0.363338951078113,
0.276944505679984));
#20613=CARTESIAN_POINT('Ctrl Pts',(-3.93927383281782,0.368869699153342,
0.261748900230602));
#20614=CARTESIAN_POINT('Ctrl Pts',(-3.93612304217305,0.373866457560057,
0.248020419337682));
#20615=CARTESIAN_POINT('Ctrl Pts',(-3.93273246601248,0.378866861656343,
0.234281921994987));
#20616=CARTESIAN_POINT('Ctrl Pts',(-3.92904932269308,0.383874882287698,
0.220522498394176));
#20617=CARTESIAN_POINT('Ctrl Pts',(-3.9242428496489,0.390410309796705,0.202566558886697));
#20618=CARTESIAN_POINT('Ctrl Pts',(-3.91894049307532,0.396957198804506,
0.184579129170088));
#20619=CARTESIAN_POINT('Ctrl Pts',(-3.9130077333512,0.403499782727413,0.166603527577014));
#20620=CARTESIAN_POINT('Ctrl Pts',(-3.90795034653693,0.409077014774833,
0.15128020846367));
#20621=CARTESIAN_POINT('Ctrl Pts',(-3.90243675237154,0.414649019758862,
0.135971250588961));
#20622=CARTESIAN_POINT('Ctrl Pts',(-3.89635541881929,0.420206121603407,
0.120703238753463));
#20623=CARTESIAN_POINT('Ctrl Pts',(-3.8900374447729,0.425979464723838,0.104841108895317));
#20624=CARTESIAN_POINT('Ctrl Pts',(-3.88310583474409,0.431738296312812,
0.0890188491421691));
#20625=CARTESIAN_POINT('Ctrl Pts',(-3.87540089395165,0.437463615370407,
0.0732886643122535));
#20626=CARTESIAN_POINT('Ctrl Pts',(-3.87075334907403,0.440917071792165,
0.0638003707744014));
#20627=CARTESIAN_POINT('Ctrl Pts',(-3.86582311762319,0.444358520125789,
0.0543450691875513));
#20628=CARTESIAN_POINT('Ctrl Pts',(-3.86057143915063,0.447779999038701,
0.0449446331331839));
#20629=CARTESIAN_POINT('Ctrl Pts',(-3.85175601294152,0.453523266651225,
0.0291651350538899));
#20630=CARTESIAN_POINT('Ctrl Pts',(-3.84204078188016,0.459203303127001,
0.0135593630950167));
#20631=CARTESIAN_POINT('Ctrl Pts',(-3.83132752297138,0.464733701807003,
-0.00163528239887109));
#20632=CARTESIAN_POINT('Ctrl Pts',(-3.82441995626527,0.468299525999133,
-0.0114323038484921));
#20633=CARTESIAN_POINT('Ctrl Pts',(-3.8170977510109,0.471803434497092,-0.0210592133264701));
#20634=CARTESIAN_POINT('Ctrl Pts',(-3.80933982107858,0.475226299554347,
-0.0304634577811197));
#20635=CARTESIAN_POINT('Ctrl Pts',(-3.80343570000945,0.477831248281349,
-0.0376204955873941));
#20636=CARTESIAN_POINT('Ctrl Pts',(-3.79727563639941,0.480390662744171,
-0.0446524290310215));
#20637=CARTESIAN_POINT('Ctrl Pts',(-3.79086906934545,0.482891327150591,
-0.0515229480212962));
#20638=CARTESIAN_POINT('Ctrl Pts',(-3.78176306264065,0.486445659238199,
-0.0612883951732427));
#20639=CARTESIAN_POINT('Ctrl Pts',(-3.77216154255004,0.48987894582093,-0.0707212725338115));
#20640=CARTESIAN_POINT('Ctrl Pts',(-3.76213783752762,0.493157146302368,
-0.0797280543330087));
#20641=CARTESIAN_POINT('Ctrl Pts',(-3.75263674507966,0.496264429065319,
-0.0882652435600765));
#20642=CARTESIAN_POINT('Ctrl Pts',(-3.74275660335202,0.499232588020461,
-0.0964201932666809));
#20643=CARTESIAN_POINT('Ctrl Pts',(-3.73258649467787,0.502043996418041,
-0.104144474355898));
#20644=CARTESIAN_POINT('Ctrl Pts',(-3.72556063050263,0.503986214950349,
-0.10948067591706));
#20645=CARTESIAN_POINT('Ctrl Pts',(-3.71839939185283,0.505853269012534,
-0.114610364793813));
#20646=CARTESIAN_POINT('Ctrl Pts',(-3.7111300071802,0.507644171485729,-0.119530828899364));
#20647=CARTESIAN_POINT('Ctrl Pts',(-3.69305477933714,0.512097226552356,
-0.131765497142509));
#20648=CARTESIAN_POINT('Ctrl Pts',(-3.67428822511307,0.516084784645751,
-0.142721222962874));
#20649=CARTESIAN_POINT('Ctrl Pts',(-3.65509432646411,0.519651775395887,
-0.152521449504278));
#20650=CARTESIAN_POINT('Ctrl Pts',(-3.64440611533146,0.521638070673514,
-0.157978750927925));
#20651=CARTESIAN_POINT('Ctrl Pts',(-3.63358642140285,0.523494019649325,
-0.163077928830628));
#20652=CARTESIAN_POINT('Ctrl Pts',(-3.62268697157354,0.525227290438691,
-0.16784005118621));
#20653=CARTESIAN_POINT('Ctrl Pts',(-3.61375034448887,0.526648425901848,
-0.171744588781219));
#20654=CARTESIAN_POINT('Ctrl Pts',(-3.6047674830026,0.52798607554658,-0.175419750975262));
#20655=CARTESIAN_POINT('Ctrl Pts',(-3.59574600476154,0.52924732199469,-0.178884997111813));
#20656=CARTESIAN_POINT('Ctrl Pts',(-3.58013963908983,0.531429167668471,
-0.184879568833261));
#20657=CARTESIAN_POINT('Ctrl Pts',(-3.56441224699608,0.533384292376045,
-0.190251229819538));
#20658=CARTESIAN_POINT('Ctrl Pts',(-3.5485570527871,0.535140904149324,-0.19507748100137));
#20659=CARTESIAN_POINT('Ctrl Pts',(-3.53268239263572,0.53689967257254,-0.199909657530206));
#20660=CARTESIAN_POINT('Ctrl Pts',(-3.51667900179308,0.538459473597168,
-0.204195175624212));
#20661=CARTESIAN_POINT('Ctrl Pts',(-3.50053180651659,0.539831120837288,
-0.207963745443901));
#20662=CARTESIAN_POINT('Ctrl Pts',(-3.48386348055343,0.541247036289682,
-0.21185394117721));
#20663=CARTESIAN_POINT('Ctrl Pts',(-3.46704135193447,0.542462516150015,
-0.215193444647276));
#20664=CARTESIAN_POINT('Ctrl Pts',(-3.45004930524678,0.543469776899708,
-0.217960870812559));
#20665=CARTESIAN_POINT('Ctrl Pts',(-3.43655982054718,0.544269411500601,
-0.220157848822329));
#20666=CARTESIAN_POINT('Ctrl Pts',(-3.42296310261358,0.544937465463458,
-0.221993312000254));
#20667=CARTESIAN_POINT('Ctrl Pts',(-3.40925535079096,0.545461019899046,
-0.223431765989889));
#20668=CARTESIAN_POINT('Ctrl Pts',(-3.39748261302319,0.545910668328423,
-0.224667164896297));
#20669=CARTESIAN_POINT('Ctrl Pts',(-3.38563650689686,0.546253524649681,
-0.225609154897069));
#20670=CARTESIAN_POINT('Ctrl Pts',(-3.3736853870908,0.546476778145907,-0.226222538836764));
#20671=CARTESIAN_POINT('Ctrl Pts',(-3.36016796810983,0.546729290972858,
-0.226916312126935));
#20672=CARTESIAN_POINT('Ctrl Pts',(-3.34651252112207,0.546829337291431,
-0.227191187128114));
#20673=CARTESIAN_POINT('Ctrl Pts',(-3.33267610475802,0.546744862736256,
-0.226959095195251));
#20674=CARTESIAN_POINT('Ctrl Pts',(-3.32110141125817,0.546674196527682,
-0.226764941382877));
#20675=CARTESIAN_POINT('Ctrl Pts',(-3.3094000957189,0.546474225573401,-0.226215525701441));
#20676=CARTESIAN_POINT('Ctrl Pts',(-3.29755962677078,0.546116630947227,
-0.225233042540711));
#20677=CARTESIAN_POINT('Ctrl Pts',(-3.28814851407603,0.545832405437181,
-0.224452139369827));
#20678=CARTESIAN_POINT('Ctrl Pts',(-3.27864397132647,0.545448060082736,
-0.223396159187217));
#20679=CARTESIAN_POINT('Ctrl Pts',(-3.26907623467603,0.544946536842993,
-0.222018235410691));
#20680=CARTESIAN_POINT('Ctrl Pts',(-3.24982747331958,0.543937552011029,
-0.219246072368296));
#20681=CARTESIAN_POINT('Ctrl Pts',(-3.23033080009046,0.542455134615159,
-0.215173164046936));
#20682=CARTESIAN_POINT('Ctrl Pts',(-3.21094931274948,0.540352353894123,
-0.209395821497827));
#20683=CARTESIAN_POINT('Ctrl Pts',(-3.20077276026693,0.539248256051144,
-0.206362337605374));
#20684=CARTESIAN_POINT('Ctrl Pts',(-3.19062885973354,0.537972925085944,
-0.202858394576155));
#20685=CARTESIAN_POINT('Ctrl Pts',(-3.18057391345523,0.536504701365254,
-0.198824483056852));
#20686=CARTESIAN_POINT('Ctrl Pts',(-3.17465003302617,0.535639696070971,
-0.1964479005431));
#20687=CARTESIAN_POINT('Ctrl Pts',(-3.1687549656581,0.534707371098516,-0.193886358733686));
#20688=CARTESIAN_POINT('Ctrl Pts',(-3.16290756953124,0.533704680892061,
-0.191131490032742));
#20689=CARTESIAN_POINT('Ctrl Pts',(-3.15405708743901,0.532187032433883,
-0.186961785163228));
#20690=CARTESIAN_POINT('Ctrl Pts',(-3.14532752481795,0.530508785283586,
-0.182350839013525));
#20691=CARTESIAN_POINT('Ctrl Pts',(-3.13684553141908,0.528682129286832,
-0.177332142909332));
#20692=CARTESIAN_POINT('Ctrl Pts',(-3.12879381283923,0.526948135951016,
-0.172568035373691));
#20693=CARTESIAN_POINT('Ctrl Pts',(-3.12096520761203,0.525080479341376,
-0.167436691011411));
#20694=CARTESIAN_POINT('Ctrl Pts',(-3.11344649454215,0.523102727922514,
-0.162002863646793));
#20695=CARTESIAN_POINT('Ctrl Pts',(-3.10446773365921,0.520740919869617,
-0.155513849352373));
#20696=CARTESIAN_POINT('Ctrl Pts',(-3.0959270560741,0.518221524243454,-0.148591866758818));
#20697=CARTESIAN_POINT('Ctrl Pts',(-3.08787517326817,0.515585575459487,
-0.141349656996029));
#20698=CARTESIAN_POINT('Ctrl Pts',(-3.08147273160297,0.513489605022683,
-0.135591025549066));
#20699=CARTESIAN_POINT('Ctrl Pts',(-3.0753789290815,0.511320332691276,-0.129630998801876));
#20700=CARTESIAN_POINT('Ctrl Pts',(-3.06960775233313,0.509104574416123,
-0.123543252973923));
#20701=CARTESIAN_POINT('Ctrl Pts',(-3.06372377560279,0.506845508249982,
-0.117336519693398));
#20702=CARTESIAN_POINT('Ctrl Pts',(-3.05817974413936,0.504540843174219,
-0.111004504438334));
#20703=CARTESIAN_POINT('Ctrl Pts',(-3.05293955472372,0.502203600541567,
-0.104582983081335));
#20704=CARTESIAN_POINT('Ctrl Pts',(-3.04420284120351,0.498306829320328,
-0.0938766921421992));
#20705=CARTESIAN_POINT('Ctrl Pts',(-3.03630814797779,0.4943198500131,-0.0829225565237586));
#20706=CARTESIAN_POINT('Ctrl Pts',(-3.02909796092231,0.490287466832876,
-0.0718436747895053));
#20707=CARTESIAN_POINT('Ctrl Pts',(-3.02161999941514,0.48610532759407,-0.0603533416658699));
#20708=CARTESIAN_POINT('Ctrl Pts',(-3.01487803363331,0.481874376480483,
-0.0487288990184732));
#20709=CARTESIAN_POINT('Ctrl Pts',(-3.00872169536913,0.477626257281286,
-0.0370572874435275));
#20710=CARTESIAN_POINT('Ctrl Pts',(-3.00349762266516,0.474021438540117,
-0.0271531293509397));
#20711=CARTESIAN_POINT('Ctrl Pts',(-2.99869545470355,0.470403755285769,
-0.0172136262988795));
#20712=CARTESIAN_POINT('Ctrl Pts',(-2.9942367434548,0.466781597354371,-0.00726182917266559));
#20713=CARTESIAN_POINT('Ctrl Pts',(-2.98835950279235,0.462007057651627,
0.00585611084891477));
#20714=CARTESIAN_POINT('Ctrl Pts',(-2.98308260387313,0.457228034424005,
0.0189863692538536));
#20715=CARTESIAN_POINT('Ctrl Pts',(-2.97827812075261,0.452466276252641,
0.0320691923065807));
#20716=CARTESIAN_POINT('Ctrl Pts',(-2.97325578738024,0.447488605111897,
0.045745231367245));
#20717=CARTESIAN_POINT('Ctrl Pts',(-2.96874974008818,0.442529710065418,
0.0593696835328924));
#20718=CARTESIAN_POINT('Ctrl Pts',(-2.9646429990344,0.437597110787006,0.0729218886695459));
#20719=CARTESIAN_POINT('Ctrl Pts',(-2.96031131519025,0.432394333128475,
0.0872164028048048));
#20720=CARTESIAN_POINT('Ctrl Pts',(-2.95642400398736,0.427220699948731,
0.101430843142691));
#20721=CARTESIAN_POINT('Ctrl Pts',(-2.95287408362541,0.422067771173593,
0.115588398596441));
#20722=CARTESIAN_POINT('Ctrl Pts',(-2.9491044072207,0.416595852922409,0.130622370432671));
#20723=CARTESIAN_POINT('Ctrl Pts',(-2.94571535463065,0.411147158745473,
0.145592534649317));
#20724=CARTESIAN_POINT('Ctrl Pts',(-2.942609760046,0.405694490587329,0.160573617289596));
#20725=CARTESIAN_POINT('Ctrl Pts',(-2.93974684524852,0.400667909064796,
0.174384036519804));
#20726=CARTESIAN_POINT('Ctrl Pts',(-2.93712392796838,0.395632789357454,
0.188217914219976));
#20727=CARTESIAN_POINT('Ctrl Pts',(-2.93470339303712,0.390603676173332,
0.202035289133233));
#20728=CARTESIAN_POINT('Ctrl Pts',(-2.93099979535042,0.382908760593194,
0.223176895934272));
#20729=CARTESIAN_POINT('Ctrl Pts',(-2.92776715655637,0.375226020910854,
0.244285049731048));
#20730=CARTESIAN_POINT('Ctrl Pts',(-2.92488564478655,0.367576098718698,
0.265303038214582));
#20731=CARTESIAN_POINT('Ctrl Pts',(-2.92184968434103,0.35951614163992,0.287447588290298));
#20732=CARTESIAN_POINT('Ctrl Pts',(-2.91920364550544,0.351492503454705,
0.309492353026049));
#20733=CARTESIAN_POINT('Ctrl Pts',(-2.91683841522211,0.34351219560062,0.331418068655445));
#20734=CARTESIAN_POINT('Ctrl Pts',(-2.91432245416582,0.335023320788077,
0.354741060519485));
#20735=CARTESIAN_POINT('Ctrl Pts',(-2.91212444088888,0.326583343686617,
0.377929707026459));
#20736=CARTESIAN_POINT('Ctrl Pts',(-2.91014448265287,0.318183739895187,
0.401007428775779));
#20737=CARTESIAN_POINT('Ctrl Pts',(-2.907919558577,0.308744914184863,0.426940389281062));
#20738=CARTESIAN_POINT('Ctrl Pts',(-2.90597008942706,0.29935700917154,0.452733446321151));
#20739=CARTESIAN_POINT('Ctrl Pts',(-2.90419078248043,0.289988480614236,
0.47847326698586));
#20740=CARTESIAN_POINT('Ctrl Pts',(-2.90291344823327,0.283262973025782,
0.496951447219508));
#20741=CARTESIAN_POINT('Ctrl Pts',(-2.90172462797116,0.276547017573975,
0.515403383173411));
#20742=CARTESIAN_POINT('Ctrl Pts',(-2.90059397675046,0.269824323391606,
0.533873833637369));
#20743=CARTESIAN_POINT('Ctrl Pts',(-2.89983485563977,0.265310695332727,
0.546274924808955));
#20744=CARTESIAN_POINT('Ctrl Pts',(-2.89910178887351,0.26079188236583,0.558690261398245));
#20745=CARTESIAN_POINT('Ctrl Pts',(-2.89838906856979,0.256276445704804,
0.571096321663392));
#20746=CARTESIAN_POINT('Ctrl Pts',(-2.89654063821258,0.244565722498618,
0.603271269237869));
#20747=CARTESIAN_POINT('Ctrl Pts',(-2.89482523118125,0.232869975283629,
0.6354050706147));
#20748=CARTESIAN_POINT('Ctrl Pts',(-2.89314446329961,0.221201583373919,
0.667463713907976));
#20749=CARTESIAN_POINT('Ctrl Pts',(-2.89134078182618,0.208679888652084,
0.70186678740952));
#20750=CARTESIAN_POINT('Ctrl Pts',(-2.88957745244866,0.196189464596047,
0.736183945462895));
#20751=CARTESIAN_POINT('Ctrl Pts',(-2.88776644175644,0.183726850734524,
0.770424695634813));
#20752=CARTESIAN_POINT('Ctrl Pts',(-2.88572744403318,0.169695326018192,
0.808975992953454));
#20753=CARTESIAN_POINT('Ctrl Pts',(-2.88362845669159,0.155698865847008,
0.847430951226077));
#20754=CARTESIAN_POINT('Ctrl Pts',(-2.88137742145133,0.141713015122622,
0.885856760283194));
#20755=CARTESIAN_POINT('Ctrl Pts',(-2.88071953338383,0.137625507232499,
0.897087095913149));
#20756=CARTESIAN_POINT('Ctrl Pts',(-2.88004882973202,0.133538801428664,
0.908315227829142));
#20757=CARTESIAN_POINT('Ctrl Pts',(-2.87936339380758,0.129452050955556,
0.919543482472952));
#20758=CARTESIAN_POINT('Origin',(-3.43968169690379,0.263987455675957,0.316006143873413));
#20759=CARTESIAN_POINT('',(-3.91503635643998,0.0542766412926798,0.892181871006905));
#20760=CARTESIAN_POINT('',(-4.5,0.0542766412926824,0.892181871006898));
#20761=CARTESIAN_POINT('Origin',(-4.07070327333776,0.0413242491918032,0.927768275831754));
#20762=CARTESIAN_POINT('Origin',(-3.2,0.9,1.2));
#20763=CARTESIAN_POINT('',(-4.05408422825637,4.03679607859634E-16,1.1999999999999));
#20764=CARTESIAN_POINT('',(-4.5,0.,1.2));
#20765=CARTESIAN_POINT('',(-3.9178024645294,0.00300376380597895,1.12653061234128));
#20766=CARTESIAN_POINT('Ctrl Pts',(-3.91780246453198,0.00300376306932705,
1.12653061227823));
#20767=CARTESIAN_POINT('Ctrl Pts',(-3.91789635426004,0.00299646731275753,
1.1266196870125));
#20768=CARTESIAN_POINT('Ctrl Pts',(-3.91799025015003,0.0029891856217416,
1.12670875309452));
#20769=CARTESIAN_POINT('Ctrl Pts',(-3.93198424061395,0.00190612082577026,
1.13998060667364));
#20770=CARTESIAN_POINT('Ctrl Pts',(-3.95372016194337,0.000728182714508301,
1.16059376321201));
#20771=CARTESIAN_POINT('Ctrl Pts',(-3.98957829615743,0.000138376987816399,
1.18285735678753));
#20772=CARTESIAN_POINT('Ctrl Pts',(-4.00792465999132,1.58115480707647E-5,
1.19293784769595));
#20773=CARTESIAN_POINT('Ctrl Pts',(-4.03839217161777,-9.33473974974476E-7,
1.19912770931096));
#20774=CARTESIAN_POINT('Ctrl Pts',(-4.04624242871877,7.69055196891966E-18,
1.19999825406822));
#20775=CARTESIAN_POINT('Ctrl Pts',(-4.05408422825637,6.93889390390723E-18,
1.19999999999961));
#20776=CARTESIAN_POINT('',(-3.91070419800688,0.0384900677109038,0.939614446316166));
#20777=CARTESIAN_POINT('Ctrl Pts',(-3.91070419800688,0.0384900677109038,
0.939614446316166));
#20778=CARTESIAN_POINT('Ctrl Pts',(-3.91354706175869,0.0201143993533441,
1.00041206192318));
#20779=CARTESIAN_POINT('Ctrl Pts',(-3.91582848502696,0.00819208764812623,
1.06318918889612));
#20780=CARTESIAN_POINT('Ctrl Pts',(-3.91780246457708,0.0030037652751779,
1.1265306125175));
#20781=CARTESIAN_POINT('Ctrl Pts',(-3.91503635643999,0.0542766412926799,
0.892181871006906));
#20782=CARTESIAN_POINT('Ctrl Pts',(-3.91141850629553,0.0486938803101099,
0.90752038074473));
#20783=CARTESIAN_POINT('Ctrl Pts',(-3.90995323778991,0.043344115284559,
0.923554376403128));
#20784=CARTESIAN_POINT('Ctrl Pts',(-3.91070419800688,0.0384900677109053,
0.939614446316161));
#20785=CARTESIAN_POINT('Ctrl Pts',(4.1,0.,11.7890187209237));
#20786=CARTESIAN_POINT('Ctrl Pts',(4.1778740733922,2.3055357147031E-16,
11.7166528289146));
#20787=CARTESIAN_POINT('Ctrl Pts',(4.25493082441583,0.00976502690773917,
11.6434441359381));
#20788=CARTESIAN_POINT('Ctrl Pts',(4.33293714067645,0.0306667563623946,
11.5737513316985));
#20789=CARTESIAN_POINT('Ctrl Pts',(4.11709141945523,0.,11.8057761908248));
#20790=CARTESIAN_POINT('Ctrl Pts',(4.19446713550167,0.00152406851324286,
11.7325672253649));
#20791=CARTESIAN_POINT('Ctrl Pts',(4.27036703049148,0.0125190657257837,
11.6590157024546));
#20792=CARTESIAN_POINT('Ctrl Pts',(4.34699197838351,0.0344327387772118,
11.5891134622547));
#20793=CARTESIAN_POINT('Ctrl Pts',(4.14667038231247,0.0201034459912815,
11.8347772097913));
#20794=CARTESIAN_POINT('Ctrl Pts',(4.22147162288739,0.0224535142329611,
11.7602048577659));
#20795=CARTESIAN_POINT('Ctrl Pts',(4.29413970444214,0.0340349382796113,
11.6860288143997));
#20796=CARTESIAN_POINT('Ctrl Pts',(4.36741004838275,0.0559487962903834,
11.6158150586253));
#20797=CARTESIAN_POINT('Ctrl Pts',(4.15712386170589,0.062048041979487,11.8450264384616));
#20798=CARTESIAN_POINT('Ctrl Pts',(4.22938050951698,0.0627480300001918,
11.7713116264474));
#20799=CARTESIAN_POINT('Ctrl Pts',(4.2996344178864,0.0724531692081621,11.6980817694637));
#20800=CARTESIAN_POINT('Ctrl Pts',(4.3703722128866,0.0923540347180163,11.6287837175683));
#20801=CARTESIAN_POINT('Ctrl Pts',(4.15712386170589,0.0800000000000001,
11.8450264384616));
#20802=CARTESIAN_POINT('Ctrl Pts',(4.22862937879342,0.0800000000000004,
11.7720959308659));
#20803=CARTESIAN_POINT('Ctrl Pts',(4.29822259191301,0.0888970245159395,
11.6995328113185));
#20804=CARTESIAN_POINT('Ctrl Pts',(4.36824305034239,0.107940822463515,11.6308715500256));
#20805=CARTESIAN_POINT('',(4.15712386170589,0.0800000000000001,11.8450264384616));
#20806=CARTESIAN_POINT('Ctrl Pts',(4.23249000178399,0.0834041484552263,
11.7678256594183));
#20807=CARTESIAN_POINT('Ctrl Pts',(4.20753856027708,0.081116204299734,11.7934084522297));
#20808=CARTESIAN_POINT('Ctrl Pts',(4.18245116805733,0.0800000000000002,
11.8191943994319));
#20809=CARTESIAN_POINT('Ctrl Pts',(4.15712386170589,0.0800000000000001,
11.8450264384616));
#20810=CARTESIAN_POINT('',(4.1,0.,11.7890187209237));
#20811=CARTESIAN_POINT('Origin',(4.1,0.0800000000000001,11.7890187209237));
#20812=CARTESIAN_POINT('Ctrl Pts',(4.1,0.,11.7890187209237));
#20813=CARTESIAN_POINT('Ctrl Pts',(4.1778740733922,2.3055357147031E-16,
11.7166528289146));
#20814=CARTESIAN_POINT('Ctrl Pts',(4.25493082441583,0.00976502690773917,
11.6434441359381));
#20815=CARTESIAN_POINT('Ctrl Pts',(4.33293714067645,0.0306667563623946,
11.5737513316985));
#20816=CARTESIAN_POINT('Ctrl Pts',(4.09999999999981,0.08,11.9026515720696));
#20817=CARTESIAN_POINT('Ctrl Pts',(4.06432399954022,0.08,11.9381300567193));
#20818=CARTESIAN_POINT('Ctrl Pts',(3.98818983778508,0.08,12.0113745379845));
#20819=CARTESIAN_POINT('Ctrl Pts',(3.86893999186953,0.08,12.1091025700166));
#20820=CARTESIAN_POINT('Ctrl Pts',(3.73111116955382,0.08,12.1934030676208));
#20821=CARTESIAN_POINT('Ctrl Pts',(3.52459155666187,0.08,12.2691718924221));
#20822=CARTESIAN_POINT('Ctrl Pts',(3.26513646721023,0.08,12.2978239927277));
#20823=CARTESIAN_POINT('Ctrl Pts',(2.86516691280962,0.08,12.3018717460263));
#20824=CARTESIAN_POINT('Ctrl Pts',(2.3724345221647,0.08,12.2928334043575));
#20825=CARTESIAN_POINT('Ctrl Pts',(1.18525410089388,0.0800000000000001,
12.2925039217734));
#20826=CARTESIAN_POINT('Ctrl Pts',(-0.197223498551522,0.08,12.3061838691053));
#20827=CARTESIAN_POINT('Ctrl Pts',(-1.58273390323592,0.08,12.2905351916681));
#20828=CARTESIAN_POINT('Ctrl Pts',(-2.37158423452643,0.08,12.2934900223558));
#20829=CARTESIAN_POINT('Ctrl Pts',(-2.8649548727089,0.08,12.3017730777117));
#20830=CARTESIAN_POINT('Ctrl Pts',(-3.26529575985038,0.08,12.2978370579524));
#20831=CARTESIAN_POINT('Ctrl Pts',(-3.52422781159081,0.08,12.2692312868616));
#20832=CARTESIAN_POINT('Ctrl Pts',(-3.73122681675827,0.08,12.1933713817583));
#20833=CARTESIAN_POINT('Ctrl Pts',(-3.86889459911728,0.08,12.1090065132441));
#20834=CARTESIAN_POINT('Ctrl Pts',(-3.98631749393431,0.08,12.0130274731947));
#20835=CARTESIAN_POINT('Ctrl Pts',(-4.06432399954019,0.08,11.9381300567181));
#20836=CARTESIAN_POINT('Ctrl Pts',(-4.0999999999998,0.08,11.9026515720685));
#20837=CARTESIAN_POINT('Ctrl Pts',(4.09999999999981,0.0560640559726492,
11.9026515720696));
#20838=CARTESIAN_POINT('Ctrl Pts',(4.06432200541893,0.0560640559726492,
11.9381320398003));
#20839=CARTESIAN_POINT('Ctrl Pts',(3.98819817514749,0.0560640559726492,
12.0113732141449));
#20840=CARTESIAN_POINT('Ctrl Pts',(3.86894130022029,0.0560640559726492,
12.1091110958518));
#20841=CARTESIAN_POINT('Ctrl Pts',(3.73109430755215,0.0560640559726492,
12.1934253732652));
#20842=CARTESIAN_POINT('Ctrl Pts',(3.52453032420505,0.0560640559726492,
12.2692082165472));
#20843=CARTESIAN_POINT('Ctrl Pts',(3.26508176198252,0.0560640559726491,
12.2978447746476));
#20844=CARTESIAN_POINT('Ctrl Pts',(2.86512835900754,0.0560640559726492,
12.301883596069));
#20845=CARTESIAN_POINT('Ctrl Pts',(2.37242466553327,0.0560640559726492,
12.2928361559738));
#20846=CARTESIAN_POINT('Ctrl Pts',(1.18525566090828,0.0560640559726493,
12.2925052045904));
#20847=CARTESIAN_POINT('Ctrl Pts',(-0.197226227294698,0.0560640559726492,
12.3061822863099));
#20848=CARTESIAN_POINT('Ctrl Pts',(-1.58273033360394,0.0560640559726493,
12.2905370248849));
#20849=CARTESIAN_POINT('Ctrl Pts',(-2.37157938813513,0.0560640559726492,
12.2934911038005));
#20850=CARTESIAN_POINT('Ctrl Pts',(-2.86490940365101,0.0560640559726493,
12.301787110831));
#20851=CARTESIAN_POINT('Ctrl Pts',(-3.26524117145924,0.0560640559726493,
12.2978577914992));
#20852=CARTESIAN_POINT('Ctrl Pts',(-3.52416558815914,0.0560640559726493,
12.2692679240856));
#20853=CARTESIAN_POINT('Ctrl Pts',(-3.73120976022586,0.0560640559726493,
12.193393737439));
#20854=CARTESIAN_POINT('Ctrl Pts',(-3.86889559828825,0.0560640559726493,
12.1090151471365));
#20855=CARTESIAN_POINT('Ctrl Pts',(-3.98632550448738,0.0560640559726493,
12.0130263967018));
#20856=CARTESIAN_POINT('Ctrl Pts',(-4.0643220054189,0.0560640559726493,
11.9381320397991));
#20857=CARTESIAN_POINT('Ctrl Pts',(-4.0999999999998,0.0560640559726493,
11.9026515720685));
#20858=CARTESIAN_POINT('Ctrl Pts',(4.08582423633291,0.0146397293840558,
11.8883968890952));
#20859=CARTESIAN_POINT('Ctrl Pts',(4.05030551310779,0.0146397293840558,
11.9237189672565));
#20860=CARTESIAN_POINT('Ctrl Pts',(3.9746955606649,0.0146397293840557,11.9964469996915));
#20861=CARTESIAN_POINT('Ctrl Pts',(3.85709175380371,0.0146397293840558,
12.0927851123546));
#20862=CARTESIAN_POINT('Ctrl Pts',(3.72224943041651,0.0146397293840557,
12.1751948890262));
#20863=CARTESIAN_POINT('Ctrl Pts',(3.52063632363833,0.0146397293840557,
12.2492384843966));
#20864=CARTESIAN_POINT('Ctrl Pts',(3.26439578123385,0.0146397293840557,
12.277728740107));
#20865=CARTESIAN_POINT('Ctrl Pts',(2.8655223444065,0.0146397293840557,12.2817567080134));
#20866=CARTESIAN_POINT('Ctrl Pts',(2.37263681728462,0.0146397293840557,
12.2727335042978));
#20867=CARTESIAN_POINT('Ctrl Pts',(1.18492866445151,0.0146397293840561,
12.2723941790853));
#20868=CARTESIAN_POINT('Ctrl Pts',(-0.197082299090637,0.0146397293840558,
12.286086899881));
#20869=CARTESIAN_POINT('Ctrl Pts',(-1.58260309447466,0.0146397293840562,
12.2704270240485));
#20870=CARTESIAN_POINT('Ctrl Pts',(-2.37177693824149,0.0146397293840558,
12.2733925401474));
#20871=CARTESIAN_POINT('Ctrl Pts',(-2.86532165277665,0.0146397293840561,
12.2816543668416));
#20872=CARTESIAN_POINT('Ctrl Pts',(-3.26455165823213,0.0146397293840562,
12.2777430390883));
#20873=CARTESIAN_POINT('Ctrl Pts',(-3.52028225283393,0.0146397293840561,
12.2492943914395));
#20874=CARTESIAN_POINT('Ctrl Pts',(-3.72236259942317,0.0146397293840561,
12.1751643380234));
#20875=CARTESIAN_POINT('Ctrl Pts',(-3.85705264607581,0.014639729384056,
12.0926856460335));
#20876=CARTESIAN_POINT('Ctrl Pts',(-3.97284413197348,0.014639729384056,
11.998081262117));
#20877=CARTESIAN_POINT('Ctrl Pts',(-4.05030551310777,0.0146397293840561,
11.9237189672553));
#20878=CARTESIAN_POINT('Ctrl Pts',(-4.08582423633293,0.0146397293840561,
11.888396889094));
#20879=CARTESIAN_POINT('Ctrl Pts',(4.05624736761446,-1.09923062066103E-16,
11.8586553600413));
#20880=CARTESIAN_POINT('Ctrl Pts',(4.02105560774433,-1.14986681133505E-16,
11.8936522850402));
#20881=CARTESIAN_POINT('Ctrl Pts',(3.94654553093069,-1.32301790805734E-16,
11.9653008115684));
#20882=CARTESIAN_POINT('Ctrl Pts',(3.83237190384969,-1.17548824419341E-16,
12.0587448002228));
#20883=CARTESIAN_POINT('Ctrl Pts',(3.7037499217885,-1.63179123823165E-16,
12.13721789838));
#20884=CARTESIAN_POINT('Ctrl Pts',(3.51234755170784,-1.2488020255128E-16,
12.207670245142));
#20885=CARTESIAN_POINT('Ctrl Pts',(3.26281784836069,-2.24963096574075E-16,
12.2358135780229));
#20886=CARTESIAN_POINT('Ctrl Pts',(2.86624100045032,-1.52293381882714E-16,
12.2397949525638));
#20887=CARTESIAN_POINT('Ctrl Pts',(2.3730530313914,-1.90334102701785E-16,
12.2307979218616));
#20888=CARTESIAN_POINT('Ctrl Pts',(1.18425058894606,2.83933512305755E-16,
12.2304371870165));
#20889=CARTESIAN_POINT('Ctrl Pts',(-0.19678931795809,-5.0793709047756E-17,
12.2441548545081));
#20890=CARTESIAN_POINT('Ctrl Pts',(-1.58232804686594,4.50897213697133E-16,
12.2284736456218));
#20891=CARTESIAN_POINT('Ctrl Pts',(-2.37217612036961,-3.31978508512746E-17,
12.2314610090552));
#20892=CARTESIAN_POINT('Ctrl Pts',(-2.8660598737781,3.25578437998814E-16,
12.2396862466115));
#20893=CARTESIAN_POINT('Ctrl Pts',(-3.26296666832,4.68732183862947E-16,
12.2358304223918));
#20894=CARTESIAN_POINT('Ctrl Pts',(-3.51201307627747,3.5252554681229E-16,
12.2077190621633));
#20895=CARTESIAN_POINT('Ctrl Pts',(-3.70385780448657,3.19211288769243E-16,
12.1371897449525));
#20896=CARTESIAN_POINT('Ctrl Pts',(-3.83234572555419,2.13429601981668E-16,
12.0586382843544));
#20897=CARTESIAN_POINT('Ctrl Pts',(-3.94473754607314,1.88196963216156E-16,
11.9668962614767));
#20898=CARTESIAN_POINT('Ctrl Pts',(-4.02105560774434,2.57336224836312E-16,
11.893652285039));
#20899=CARTESIAN_POINT('Ctrl Pts',(-4.05624736761451,2.50899420937073E-16,
11.8586553600401));
#20900=CARTESIAN_POINT('Ctrl Pts',(4.0435887019288,-1.11022302462516E-16,
11.8459262210355));
#20901=CARTESIAN_POINT('Ctrl Pts',(4.00853667496432,-1.16081809443283E-16,
11.8807841867429));
#20902=CARTESIAN_POINT('Ctrl Pts',(3.93449839739079,-1.33394172299536E-16,
11.9519703536246));
#20903=CARTESIAN_POINT('Ctrl Pts',(3.82179213813238,-1.18666346909376E-16,
12.0441766918018));
#20904=CARTESIAN_POINT('Ctrl Pts',(3.69583054658886,-1.64263096837451E-16,
12.1209663380819));
#20905=CARTESIAN_POINT('Ctrl Pts',(3.50879373356752,-1.2597952000311E-16,
12.1898830987469));
#20906=CARTESIAN_POINT('Ctrl Pts',(3.26213688664597,-2.26051670054873E-16,
12.2178763550172));
#20907=CARTESIAN_POINT('Ctrl Pts',(2.86654461957332,-1.53389929340232E-16,
12.221836870547));
#20908=CARTESIAN_POINT('Ctrl Pts',(2.37323015533067,-1.91431012567934E-16,
12.212850107161));
#20909=CARTESIAN_POINT('Ctrl Pts',(1.18396053823096,2.82832847689486E-16,
12.212480058298));
#20910=CARTESIAN_POINT('Ctrl Pts',(-0.196664204629831,-5.18915455952868E-17,
12.2262081084424));
#20911=CARTESIAN_POINT('Ctrl Pts',(-1.58220996201918,4.49796397254339E-16,
12.2105181200467));
#20912=CARTESIAN_POINT('Ctrl Pts',(-2.37234646937341,-3.42995743393534E-17,
12.2135147567495));
#20913=CARTESIAN_POINT('Ctrl Pts',(-2.86637115626172,3.24464130618306E-16,
12.2217256647492));
#20914=CARTESIAN_POINT('Ctrl Pts',(-3.26228269824909,4.67598234842018E-16,
12.2178942838233));
#20915=CARTESIAN_POINT('Ctrl Pts',(-3.50846754301617,3.51404355795733E-16,
12.1899289134544));
#20916=CARTESIAN_POINT('Ctrl Pts',(-3.69593614680787,3.18100712493542E-16,
12.1209392159371));
#20917=CARTESIAN_POINT('Ctrl Pts',(-3.82177146177483,2.12368510762661E-16,
12.0440671698819));
#20918=CARTESIAN_POINT('Ctrl Pts',(-3.93270897258269,1.87121689875167E-16,
11.9535492174884));
#20919=CARTESIAN_POINT('Ctrl Pts',(-4.00853667496434,2.56231757211128E-16,
11.8807841867417));
#20920=CARTESIAN_POINT('Ctrl Pts',(-4.04358870192886,2.4980018054066E-16,
11.8459262210343));
#20921=CARTESIAN_POINT('',(-4.04358870192886,0.,11.8459262210343));
#20922=CARTESIAN_POINT('Origin',(-4.04358870192886,0.08,11.8459262210343));
#20923=CARTESIAN_POINT('',(4.0435887019288,0.,11.8459262210355));
#20924=CARTESIAN_POINT('Ctrl Pts',(-4.04358870192886,2.4980018054066E-16,
11.8459262210343));
#20925=CARTESIAN_POINT('Ctrl Pts',(-4.00853667496434,2.56231757211128E-16,
11.8807841867417));
#20926=CARTESIAN_POINT('Ctrl Pts',(-3.93270897258269,1.87121689875167E-16,
11.9535492174884));
#20927=CARTESIAN_POINT('Ctrl Pts',(-3.82177146177483,2.12368510762661E-16,
12.0440671698819));
#20928=CARTESIAN_POINT('Ctrl Pts',(-3.69593614680787,3.18100712493542E-16,
12.1209392159371));
#20929=CARTESIAN_POINT('Ctrl Pts',(-3.50846754301617,3.51404355795733E-16,
12.1899289134544));
#20930=CARTESIAN_POINT('Ctrl Pts',(-3.26228269824909,4.67598234842018E-16,
12.2178942838233));
#20931=CARTESIAN_POINT('Ctrl Pts',(-2.86637115626172,3.24464130618306E-16,
12.2217256647492));
#20932=CARTESIAN_POINT('Ctrl Pts',(-2.37234646937341,-3.42995743393534E-17,
12.2135147567495));
#20933=CARTESIAN_POINT('Ctrl Pts',(-1.58220996201918,4.49796397254339E-16,
12.2105181200467));
#20934=CARTESIAN_POINT('Ctrl Pts',(-0.196664204629831,-5.18915455952868E-17,
12.2262081084424));
#20935=CARTESIAN_POINT('Ctrl Pts',(1.18396053823096,2.82832847689486E-16,
12.212480058298));
#20936=CARTESIAN_POINT('Ctrl Pts',(2.37323015533067,-1.91431012567934E-16,
12.212850107161));
#20937=CARTESIAN_POINT('Ctrl Pts',(2.86654461957332,-1.53389929340232E-16,
12.221836870547));
#20938=CARTESIAN_POINT('Ctrl Pts',(3.26213688664597,-2.26051670054873E-16,
12.2178763550172));
#20939=CARTESIAN_POINT('Ctrl Pts',(3.50879373356752,-1.2597952000311E-16,
12.1898830987469));
#20940=CARTESIAN_POINT('Ctrl Pts',(3.69583054658886,-1.64263096837451E-16,
12.1209663380819));
#20941=CARTESIAN_POINT('Ctrl Pts',(3.82179213813238,-1.18666346909376E-16,
12.0441766918018));
#20942=CARTESIAN_POINT('Ctrl Pts',(3.93449839739079,-1.33394172299536E-16,
11.9519703536246));
#20943=CARTESIAN_POINT('Ctrl Pts',(4.00853667496432,-1.16081809443283E-16,
11.8807841867429));
#20944=CARTESIAN_POINT('Ctrl Pts',(4.0435887019288,-1.11022302462516E-16,
11.8459262210355));
#20945=CARTESIAN_POINT('Origin',(4.0435887019288,0.08,11.8459262210355));
#20946=CARTESIAN_POINT('Ctrl Pts',(4.15712386170585,0.08,11.8450264384616));
#20947=CARTESIAN_POINT('Ctrl Pts',(4.13827843210564,0.08,11.8642474273109));
#20948=CARTESIAN_POINT('Ctrl Pts',(4.11927627294067,0.08,11.8834820198546));
#20949=CARTESIAN_POINT('Ctrl Pts',(4.09999999999983,0.08,11.9026515720696));
#20950=CARTESIAN_POINT('Ctrl Pts',(4.15712386170585,0.0560640559726494,
11.8450264384616));
#20951=CARTESIAN_POINT('Ctrl Pts',(4.13827796583819,0.0560640559726494,
11.8642479028703));
#20952=CARTESIAN_POINT('Ctrl Pts',(4.11927735039403,0.0560640559726492,
11.8834809483664));
#20953=CARTESIAN_POINT('Ctrl Pts',(4.09999999999983,0.0560640559726491,
11.9026515720696));
#20954=CARTESIAN_POINT('Ctrl Pts',(4.14276903578864,0.0146397293927042,
11.8309520917479));
#20955=CARTESIAN_POINT('Ctrl Pts',(4.12396038090976,0.0146397293927042,
11.8501355730145));
#20956=CARTESIAN_POINT('Ctrl Pts',(4.10501553004289,0.0146397293927035,
11.8693118456237));
#20957=CARTESIAN_POINT('Ctrl Pts',(4.08582423632785,0.0146397293927031,
11.88839688909));
#20958=CARTESIAN_POINT('Ctrl Pts',(4.11281856459138,1.07485755671115E-15,
11.8015868233495));
#20959=CARTESIAN_POINT('Ctrl Pts',(4.09408636061341,1.00638808982717E-15,
11.8206923301711));
#20960=CARTESIAN_POINT('Ctrl Pts',(4.07526199817246,7.19794876773123E-16,
11.8397460016581));
#20961=CARTESIAN_POINT('Ctrl Pts',(4.05624736761449,-2.53423937412745E-16,
11.8586553600413));
#20962=CARTESIAN_POINT('Ctrl Pts',(4.09999999999996,1.22124532708767E-15,
11.7890187209237));
#20963=CARTESIAN_POINT('Ctrl Pts',(4.0813004685107,1.13295521928305E-15,
11.8080909041462));
#20964=CARTESIAN_POINT('Ctrl Pts',(4.06252783272243,1.14575066216236E-15,
11.8270919444215));
#20965=CARTESIAN_POINT('Ctrl Pts',(4.04358870192882,-1.11022302462516E-16,
11.8459262210355));
#20966=CARTESIAN_POINT('Ctrl Pts',(4.04358870192882,-1.11022302462516E-16,
11.8459262210355));
#20967=CARTESIAN_POINT('Ctrl Pts',(4.06252783272243,1.14575066216236E-15,
11.8270919444215));
#20968=CARTESIAN_POINT('Ctrl Pts',(4.0813004685107,1.13295521928305E-15,
11.8080909041462));
#20969=CARTESIAN_POINT('Ctrl Pts',(4.09999999999996,1.22124532708767E-15,
11.7890187209237));
#20970=CARTESIAN_POINT('Ctrl Pts',(4.15712386170585,0.08,11.8450264384616));
#20971=CARTESIAN_POINT('Ctrl Pts',(4.13827843210564,0.08,11.8642474273109));
#20972=CARTESIAN_POINT('Ctrl Pts',(4.11927627294067,0.08,11.8834820198546));
#20973=CARTESIAN_POINT('Ctrl Pts',(4.09999999999983,0.08,11.9026515720696));
#20974=CARTESIAN_POINT('Ctrl Pts',(-4.26119373042794,0.014552891884149,
11.638842338191));
#20975=CARTESIAN_POINT('Ctrl Pts',(-4.20740273136266,0.00476035687747917,
11.6883109569019));
#20976=CARTESIAN_POINT('Ctrl Pts',(-4.15394513638752,2.66182811039857E-16,
11.7388892266742));
#20977=CARTESIAN_POINT('Ctrl Pts',(-4.1,0.,11.7890187209227));
#20978=CARTESIAN_POINT('Ctrl Pts',(-4.27643939137202,0.017328331476068,
11.6544471019321));
#20979=CARTESIAN_POINT('Ctrl Pts',(-4.2234768418442,0.00670578391947384,
11.7041521797741));
#20980=CARTESIAN_POINT('Ctrl Pts',(-4.17069133240935,0.00105575681647751,
11.7550626804798));
#20981=CARTESIAN_POINT('Ctrl Pts',(-4.1170914194552,0.,11.8057761908238));
#20982=CARTESIAN_POINT('Ctrl Pts',(-4.29989809966375,0.0386834060206609,
11.6815396961087));
#20983=CARTESIAN_POINT('Ctrl Pts',(-4.24916885028947,0.0278752704198574,
11.7316116548977));
#20984=CARTESIAN_POINT('Ctrl Pts',(-4.19848690136659,0.0217313873072571,
11.7831192542213));
#20985=CARTESIAN_POINT('Ctrl Pts',(-4.14667038594628,0.0201034417498351,
11.8347772133533));
#20986=CARTESIAN_POINT('Ctrl Pts',(-4.3051722926355,0.0768991460759326,
11.6936574822235));
#20987=CARTESIAN_POINT('Ctrl Pts',(-4.25617484947063,0.0674142792550516,
11.7430966000368));
#20988=CARTESIAN_POINT('Ctrl Pts',(-4.20717768002144,0.0625329395532443,
11.7939625167387));
#20989=CARTESIAN_POINT('Ctrl Pts',(-4.15712386170579,0.0620480419794868,
11.8450264384607));
#20990=CARTESIAN_POINT('Ctrl Pts',(-4.3036970099402,0.0932593014944473,
11.695146582961));
#20991=CARTESIAN_POINT('Ctrl Pts',(-4.25517797344347,0.0843372140439259,
11.7441200666597));
#20992=CARTESIAN_POINT('Ctrl Pts',(-4.20665735473779,0.0800000000000001,
11.7945058221931));
#20993=CARTESIAN_POINT('Ctrl Pts',(-4.15712386170579,0.0799999999999999,
11.8450264384607));
#20994=CARTESIAN_POINT('Origin',(-4.1,0.0799999999999999,11.7890187209227));
#20995=CARTESIAN_POINT('Ctrl Pts',(-4.0999999999998,0.08,11.9026515720685));
#20996=CARTESIAN_POINT('Ctrl Pts',(-4.11927627294061,0.08,11.8834820198536));
#20997=CARTESIAN_POINT('Ctrl Pts',(-4.13827843210557,0.08,11.8642474273099));
#20998=CARTESIAN_POINT('Ctrl Pts',(-4.15712386170576,0.08,11.8450264384607));
#20999=CARTESIAN_POINT('Ctrl Pts',(-4.0999999999998,0.0560640559726492,
11.9026515720685));
#21000=CARTESIAN_POINT('Ctrl Pts',(-4.11927735039396,0.0560640559726493,
11.8834809483654));
#21001=CARTESIAN_POINT('Ctrl Pts',(-4.13827796583812,0.0560640559726492,
11.8642479028694));
#21002=CARTESIAN_POINT('Ctrl Pts',(-4.15712386170576,0.0560640559726492,
11.8450264384607));
#21003=CARTESIAN_POINT('Ctrl Pts',(-4.08582423632784,0.0146397293927034,
11.8883968890889));
#21004=CARTESIAN_POINT('Ctrl Pts',(-4.10501553004285,0.0146397293927039,
11.8693118456227));
#21005=CARTESIAN_POINT('Ctrl Pts',(-4.12396038090971,0.0146397293927035,
11.8501355730135));
#21006=CARTESIAN_POINT('Ctrl Pts',(-4.14276903578857,0.0146397293927034,
11.830952091747));
#21007=CARTESIAN_POINT('Ctrl Pts',(-4.05624736761451,1.39140256632356E-16,
11.8586553600401));
#21008=CARTESIAN_POINT('Ctrl Pts',(-4.07526199817246,1.14622689682545E-15,
11.839746001657));
#21009=CARTESIAN_POINT('Ctrl Pts',(-4.0940863606134,5.30685220103077E-16,
11.8206923301701));
#21010=CARTESIAN_POINT('Ctrl Pts',(-4.11281856459137,3.64434135141482E-16,
11.8015868233486));
#21011=CARTESIAN_POINT('Ctrl Pts',(-4.04358870192886,2.77555756156289E-16,
11.8459262210343));
#21012=CARTESIAN_POINT('Ctrl Pts',(-4.06252783272245,1.56490939312256E-15,
11.8270919444204));
#21013=CARTESIAN_POINT('Ctrl Pts',(-4.08130046851071,8.50913911948276E-16,
11.8080909041452));
#21014=CARTESIAN_POINT('Ctrl Pts',(-4.09999999999997,6.38378239159465E-16,
11.7890187209227));
#21015=CARTESIAN_POINT('Ctrl Pts',(-4.09999999999997,6.38378239159465E-16,
11.7890187209227));
#21016=CARTESIAN_POINT('Ctrl Pts',(-4.08130046851071,8.50913911948276E-16,
11.8080909041452));
#21017=CARTESIAN_POINT('Ctrl Pts',(-4.06252783272245,1.56490939312256E-15,
11.8270919444204));
#21018=CARTESIAN_POINT('Ctrl Pts',(-4.04358870192886,2.77555756156289E-16,
11.8459262210343));
#21019=CARTESIAN_POINT('Origin',(4.1,0.9,6.5));
#21020=CARTESIAN_POINT('',(4.10000000000037,6.53231808922516E-18,3.51568653184868));
#21021=CARTESIAN_POINT('',(4.1,0.,-0.5));
#21022=CARTESIAN_POINT('Ctrl Pts',(4.33293714059217,0.0306667563398109,
3.61523506307459));
#21023=CARTESIAN_POINT('Ctrl Pts',(4.31105117291262,0.0248024289745047,
3.63206334799651));
#21024=CARTESIAN_POINT('Ctrl Pts',(4.25303821911669,0.0114738356156513,
3.65326412679659));
#21025=CARTESIAN_POINT('Ctrl Pts',(4.15558369197843,0.000126613028484238,
3.61126292396189));
#21026=CARTESIAN_POINT('Ctrl Pts',(4.11687019564162,1.39427594163973E-14,
3.55256131194227));
#21027=CARTESIAN_POINT('Ctrl Pts',(4.10000000000067,1.11022302462516E-15,
3.51568653184854));
#21028=CARTESIAN_POINT('Origin',(0.,0.,6.75052439809906));
#21029=CARTESIAN_POINT('',(4.02,0.,1.28));
#21030=CARTESIAN_POINT('',(2.05,0.,1.28));
#21031=CARTESIAN_POINT('',(4.02,0.,3.08202325217412));
#21032=CARTESIAN_POINT('',(4.02,0.,9.32658798508426));
#21033=CARTESIAN_POINT('',(4.0212525797096,0.,3.10200465730851));
#21034=CARTESIAN_POINT('Origin',(4.18005218222794,-2.82131847876398E-16,
3.08201998101282));
#21035=CARTESIAN_POINT('',(4.08065440441665,0.,3.45401819866313));
#21036=CARTESIAN_POINT('Ctrl Pts',(4.08065440441665,-1.66533453693773E-16,
3.45401819866313));
#21037=CARTESIAN_POINT('Ctrl Pts',(4.0550039783989,-1.5992419952717E-16,
3.33776776889323));
#21038=CARTESIAN_POINT('Ctrl Pts',(4.03612145990415,4.46335323570744E-16,
3.22013430623041));
#21039=CARTESIAN_POINT('Ctrl Pts',(4.02125257970961,4.44089209850063E-16,
3.10200465730851));
#21040=CARTESIAN_POINT('Origin',(4.41014376905476,-1.89597157664411E-14,
3.2836903911759));
#21041=CARTESIAN_POINT('',(-4.1,-3.46944695195361E-18,1.26933116532693));
#21042=CARTESIAN_POINT('',(-4.1,0.,-0.5));
#21043=CARTESIAN_POINT('',(-4.05989131075898,5.20211316432632E-18,1.20000798754555));
#21044=CARTESIAN_POINT('Ctrl Pts',(-4.05990512546201,5.20005590072221E-18,
1.20001597509111));
#21045=CARTESIAN_POINT('Ctrl Pts',(-4.07021467126473,5.64716117898825E-18,
1.20597960426501));
#21046=CARTESIAN_POINT('Ctrl Pts',(-4.09130896359301,6.56198028176264E-18,
1.22537277009846));
#21047=CARTESIAN_POINT('Ctrl Pts',(-4.1,6.93889390390737E-18,1.25328382445493));
#21048=CARTESIAN_POINT('Ctrl Pts',(-4.1,6.93889390390723E-18,1.26933116532693));
#21049=CARTESIAN_POINT('',(-4.5,0.,1.2));
#21050=CARTESIAN_POINT('',(-3.3,0.,10.7));
#21051=CARTESIAN_POINT('Origin',(-3.,0.,10.7));
#21052=CARTESIAN_POINT('',(2.64,0.,11.7));
#21053=CARTESIAN_POINT('Origin',(3.,0.,11.7));
#21054=CARTESIAN_POINT('',(-3.36,0.,11.7));
#21055=CARTESIAN_POINT('Origin',(-3.,0.,11.7));
#21056=CARTESIAN_POINT('',(2.7,0.,10.7));
#21057=CARTESIAN_POINT('Origin',(3.,0.,10.7));
#21058=CARTESIAN_POINT('Origin',(2.05,0.08,1.28));
#21059=CARTESIAN_POINT('',(4.02,0.08,1.2));
#21060=CARTESIAN_POINT('',(2.05,0.08,1.2));
#21061=CARTESIAN_POINT('Origin',(4.02,0.08,1.28));
#21062=CARTESIAN_POINT('Origin',(4.02,0.,1.28));
#21063=CARTESIAN_POINT('',(4.1,0.08,1.28));
#21064=CARTESIAN_POINT('Origin',(4.02,0.08,1.28));
#21065=CARTESIAN_POINT('',(4.02,0.42,1.2));
#21066=CARTESIAN_POINT('',(4.02,0.,1.2));
#21067=CARTESIAN_POINT('',(4.1,0.42,1.28));
#21068=CARTESIAN_POINT('Origin',(4.02,0.42,1.28));
#21069=CARTESIAN_POINT('',(4.1,0.,1.28));
#21070=CARTESIAN_POINT('Origin',(2.05,0.42,1.28));
#21071=CARTESIAN_POINT('',(4.02,0.5,1.28));
#21072=CARTESIAN_POINT('',(2.05,0.5,1.28));
#21073=CARTESIAN_POINT('Origin',(4.02,0.42,1.28));
#21074=CARTESIAN_POINT('',(2.05,0.42,1.2));
#21075=CARTESIAN_POINT('Origin',(4.02,0.42,1.28));
#21076=CARTESIAN_POINT('Origin',(4.02,0.42,1.28));
#21077=CARTESIAN_POINT('Origin',(4.02,0.08,1.28));
#21078=CARTESIAN_POINT('Origin',(4.02,0.08,1.28));
#21079=CARTESIAN_POINT('Origin',(4.02,0.08,9.32658798508426));
#21080=CARTESIAN_POINT('',(4.1,0.08,3.08202325217433));
#21081=CARTESIAN_POINT('',(4.1,0.08,9.32658798508426));
#21082=CARTESIAN_POINT('Origin',(4.02,0.08,3.08202325217412));
#21083=CARTESIAN_POINT('Origin',(4.1,0.,11.9026515720695));
#21084=CARTESIAN_POINT('',(4.09999995360518,0.420060922767902,2.91110490125779));
#21085=CARTESIAN_POINT('',(4.1,0.42,9.32658798508426));
#21086=CARTESIAN_POINT('',(4.10001562649967,0.307717888808026,3.08199713129763));
#21087=CARTESIAN_POINT('Ctrl Pts',(4.1,0.420108484733097,2.91112675763541));
#21088=CARTESIAN_POINT('Ctrl Pts',(4.1,0.403846880854867,2.94612344156548));
#21089=CARTESIAN_POINT('Ctrl Pts',(4.10000000001308,0.38486882493947,2.98262906973082));
#21090=CARTESIAN_POINT('Ctrl Pts',(4.10000000001308,0.354969676766091,3.02928232732464));
#21091=CARTESIAN_POINT('Ctrl Pts',(4.09999999999961,0.344338937185448,3.04446410228447));
#21092=CARTESIAN_POINT('Ctrl Pts',(4.09999999999961,0.327298117371871,3.06460863705819));
#21093=CARTESIAN_POINT('Ctrl Pts',(4.1,0.317366554193231,3.07555920769984));
#21094=CARTESIAN_POINT('Ctrl Pts',(4.1,0.307684300216189,3.08193081722902));
#21095=CARTESIAN_POINT('',(4.1,0.08,3.08202325217412));
#21096=CARTESIAN_POINT('Origin',(4.02,0.42,9.32658798508426));
#21097=CARTESIAN_POINT('',(4.02,0.5,9.32658798508426));
#21098=CARTESIAN_POINT('Ctrl Pts',(4.08072994232021,0.472075657516576,2.72825956479583));
#21099=CARTESIAN_POINT('Ctrl Pts',(4.08122454955537,0.471498853107479,2.73157912921552));
#21100=CARTESIAN_POINT('Ctrl Pts',(4.0817174163307,0.470907450992412,2.73489656248772));
#21101=CARTESIAN_POINT('Ctrl Pts',(4.08632402965424,0.465210421595644,2.76604215816752));
#21102=CARTESIAN_POINT('Ctrl Pts',(4.090310411307,0.459013812808448,2.79397090075911));
#21103=CARTESIAN_POINT('Ctrl Pts',(4.09495793357299,0.448192539461495,2.83357438640932));
#21104=CARTESIAN_POINT('Ctrl Pts',(4.09626884293072,0.444498335917193,2.84600777143549));
#21105=CARTESIAN_POINT('Ctrl Pts',(4.09809490830362,0.43761039207076,2.86702885206655));
#21106=CARTESIAN_POINT('Ctrl Pts',(4.09874538136808,0.434501757347987,2.87590964228465));
#21107=CARTESIAN_POINT('Ctrl Pts',(4.09945899238873,0.429453602695266,2.88918275571946));
#21108=CARTESIAN_POINT('Ctrl Pts',(4.09965766008674,0.427632208943707,2.89377446083871));
#21109=CARTESIAN_POINT('Ctrl Pts',(4.09992238135085,0.423953166512825,2.9025897644674));
#21110=CARTESIAN_POINT('Ctrl Pts',(4.09999693148384,0.422075613013451,2.90688508225406));
#21111=CARTESIAN_POINT('Ctrl Pts',(4.09999990721035,0.420121845535804,2.91109776321207));
#21112=CARTESIAN_POINT('Origin',(0.,0.5,6.75052439809906));
#21113=CARTESIAN_POINT('',(-2.87936339380758,0.5,1.05441190629352));
#21114=CARTESIAN_POINT('',(-2.88715652190429,0.5,0.898556263634797));
#21115=CARTESIAN_POINT('Ctrl Pts',(-2.87936339380758,0.5,1.05441190629352));
#21116=CARTESIAN_POINT('Ctrl Pts',(-2.88225640305787,0.5,1.00074289678204));
#21117=CARTESIAN_POINT('Ctrl Pts',(-2.88479548403111,0.5,0.94877882392077));
#21118=CARTESIAN_POINT('Ctrl Pts',(-2.88715652190429,0.5,0.898556263634797));
#21119=CARTESIAN_POINT('',(-2.89976430745756,0.500020637206737,1.05079292247917));
#21120=CARTESIAN_POINT('Ctrl Pts',(-2.88715652190429,0.5,0.898556263634783));
#21121=CARTESIAN_POINT('Ctrl Pts',(-2.88603713588444,0.5,0.924909290748928));
#21122=CARTESIAN_POINT('Ctrl Pts',(-2.886491373252,0.499999999978573,0.951912747979301));
#21123=CARTESIAN_POINT('Ctrl Pts',(-2.89056682713583,0.499999999978573,
1.00214907554527));
#21124=CARTESIAN_POINT('Ctrl Pts',(-2.89410001522392,0.5,1.02750911559584));
#21125=CARTESIAN_POINT('Ctrl Pts',(-2.89983611779302,0.5,1.05077445318157));
#21126=CARTESIAN_POINT('',(-2.94907641594456,0.5,1.2));
#21127=CARTESIAN_POINT('Ctrl Pts',(-2.89974754967704,0.5,1.05079644977824));
#21128=CARTESIAN_POINT('Ctrl Pts',(-2.90603688042105,0.5,1.0759238598806));
#21129=CARTESIAN_POINT('Ctrl Pts',(-2.91415049349688,0.499999999999601,
1.10134719163055));
#21130=CARTESIAN_POINT('Ctrl Pts',(-2.93088651158465,0.499999999999601,
1.15007567318975));
#21131=CARTESIAN_POINT('Ctrl Pts',(-2.93983934236369,0.5,1.17435149002438));
#21132=CARTESIAN_POINT('Ctrl Pts',(-2.94896009810987,0.5,1.19967694937972));
#21133=CARTESIAN_POINT('Ctrl Pts',(-2.94901825916661,0.499999999999999,
1.19983846830976));
#21134=CARTESIAN_POINT('Ctrl Pts',(-2.94907641594456,0.499999999999999,
1.2));
#21135=CARTESIAN_POINT('',(-3.91996273602064,0.5,1.19999999999642));
#21136=CARTESIAN_POINT('',(-4.5,0.5,1.2));
#21137=CARTESIAN_POINT('',(-3.9565294294013,0.499872084413071,1.10578825936713));
#21138=CARTESIAN_POINT('Ctrl Pts',(-3.95639036913989,0.5,1.10574453980859));
#21139=CARTESIAN_POINT('Ctrl Pts',(-3.95076346391642,0.5,1.12156459291084));
#21140=CARTESIAN_POINT('Ctrl Pts',(-3.94468196650963,0.5,1.13750333307378));
#21141=CARTESIAN_POINT('Ctrl Pts',(-3.93253478628767,0.5,1.16853559910449));
#21142=CARTESIAN_POINT('Ctrl Pts',(-3.92630639980323,0.5,1.18405004798573));
#21143=CARTESIAN_POINT('Ctrl Pts',(-3.92009288044491,0.5,1.19967272770361));
#21144=CARTESIAN_POINT('Ctrl Pts',(-3.92002780536768,0.5,1.19983636257788));
#21145=CARTESIAN_POINT('Ctrl Pts',(-3.91996273602209,0.5,1.199999999997));
#21146=CARTESIAN_POINT('',(-4.05976551316264,0.500000001208332,1.2));
#21147=CARTESIAN_POINT('Ctrl Pts',(-4.05976550743572,0.5,1.2));
#21148=CARTESIAN_POINT('Ctrl Pts',(-4.04742877842025,0.5,1.19999809186902));
#21149=CARTESIAN_POINT('Ctrl Pts',(-4.035091497052,0.5,1.19762022778872));
#21150=CARTESIAN_POINT('Ctrl Pts',(-4.007915635338,0.5,1.18794866440528));
#21151=CARTESIAN_POINT('Ctrl Pts',(-3.99341012555002,0.500000000024842,
1.1792057307165));
#21152=CARTESIAN_POINT('Ctrl Pts',(-3.97352459100036,0.500000000024842,
1.1611448793698));
#21153=CARTESIAN_POINT('Ctrl Pts',(-3.96617262558927,0.5,1.15272746382386));
#21154=CARTESIAN_POINT('Ctrl Pts',(-3.95707696368493,0.5,1.13661229032071));
#21155=CARTESIAN_POINT('Ctrl Pts',(-3.95543177553355,0.5,1.13081595575233));
#21156=CARTESIAN_POINT('Ctrl Pts',(-3.95416491149362,0.5,1.12308915103081));
#21157=CARTESIAN_POINT('Ctrl Pts',(-3.9540319481804,0.5,1.11975105593971));
#21158=CARTESIAN_POINT('Ctrl Pts',(-3.95465641496988,0.5,1.11277077485612));
#21159=CARTESIAN_POINT('Ctrl Pts',(-3.95546639835865,0.5,1.10925940502722));
#21160=CARTESIAN_POINT('Ctrl Pts',(-3.95666399897708,0.5,1.10584429672409));
#21161=CARTESIAN_POINT('',(-4.05989131075939,0.499999999999496,1.20000798754579));
#21162=CARTESIAN_POINT('',(-4.5,0.5,1.2));
#21163=CARTESIAN_POINT('',(-4.1,0.5,1.26933116532693));
#21164=CARTESIAN_POINT('Ctrl Pts',(-4.1,0.5,1.26933116532693));
#21165=CARTESIAN_POINT('Ctrl Pts',(-4.1,0.5,1.25328382445493));
#21166=CARTESIAN_POINT('Ctrl Pts',(-4.09130896359301,0.5,1.22537277009847));
#21167=CARTESIAN_POINT('Ctrl Pts',(-4.07021467126473,0.5,1.20597960426501));
#21168=CARTESIAN_POINT('Ctrl Pts',(-4.05990512546201,0.5,1.20001597509111));
#21169=CARTESIAN_POINT('',(-4.1,0.5,-0.5));
#21170=CARTESIAN_POINT('',(-4.1,0.5,-0.5));
#21171=CARTESIAN_POINT('',(4.1,0.5,11.7890187209237));
#21172=CARTESIAN_POINT('Ctrl Pts',(4.09999999999996,0.499999999999999,11.7890187209237));
#21173=CARTESIAN_POINT('Ctrl Pts',(4.08130046851069,0.499999999999999,11.8080909041462));
#21174=CARTESIAN_POINT('Ctrl Pts',(4.06252783272241,0.5,11.8270919444215));
#21175=CARTESIAN_POINT('Ctrl Pts',(4.0435887019288,0.500000000000001,11.8459262210355));
#21176=CARTESIAN_POINT('',(4.1,0.5,-0.5));
#21177=CARTESIAN_POINT('',(-4.5,0.5,1.2));
#21178=CARTESIAN_POINT('',(-2.803641505311,0.5,1.2));
#21179=CARTESIAN_POINT('',(-4.5,0.5,1.2));
#21180=CARTESIAN_POINT('Ctrl Pts',(-2.803641505311,0.5,1.2));
#21181=CARTESIAN_POINT('Ctrl Pts',(-2.82677300877682,0.5,1.2));
#21182=CARTESIAN_POINT('Ctrl Pts',(-2.86687236848074,0.5,1.18130984727687));
#21183=CARTESIAN_POINT('Ctrl Pts',(-2.88261462067416,0.5,1.14154581001999));
#21184=CARTESIAN_POINT('Ctrl Pts',(-2.88353005387198,0.5,1.12422135153951));
#21185=CARTESIAN_POINT('Ctrl Pts',(-2.8852657140673,0.5,1.09088035845137));
#21186=CARTESIAN_POINT('Ctrl Pts',(-2.88558432089061,0.5,1.0846730825913));
#21187=CARTESIAN_POINT('Ctrl Pts',(-2.88523738147895,0.500000000000113,
1.07842688666836));
#21188=CARTESIAN_POINT('Ctrl Pts',(-2.88325561528678,0.500000000000113,
1.06618259874669));
#21189=CARTESIAN_POINT('Ctrl Pts',(-2.88162442549406,0.5,1.0601716794206));
#21190=CARTESIAN_POINT('Ctrl Pts',(-2.87936339380758,0.5,1.05441190629352));
#21191=CARTESIAN_POINT('',(2.7,0.5,10.7));
#21192=CARTESIAN_POINT('Origin',(3.,0.5,10.7));
#21193=CARTESIAN_POINT('',(-3.36,0.5,11.7));
#21194=CARTESIAN_POINT('Origin',(-3.,0.5,11.7));
#21195=CARTESIAN_POINT('',(2.64,0.5,11.7));
#21196=CARTESIAN_POINT('Origin',(3.,0.5,11.7));
#21197=CARTESIAN_POINT('',(-3.3,0.5,10.7));
#21198=CARTESIAN_POINT('Origin',(-3.,0.5,10.7));
#21199=CARTESIAN_POINT('Ctrl Pts',(4.1,0.08,3.08202325217412));
#21200=CARTESIAN_POINT('Ctrl Pts',(4.1,0.08,3.08536220394432));
#21201=CARTESIAN_POINT('Ctrl Pts',(4.10020930892952,0.08,3.08870114236636));
#21202=CARTESIAN_POINT('Ctrl Pts',(4.1006262898548,0.08,3.09201395474132));
#21203=CARTESIAN_POINT('Ctrl Pts',(4.1,0.0560640559726492,3.08202325217412));
#21204=CARTESIAN_POINT('Ctrl Pts',(4.1,0.0560640559726492,3.08535153317887));
#21205=CARTESIAN_POINT('Ctrl Pts',(4.10021064153507,0.0560640559726493,
3.0887117295944));
#21206=CARTESIAN_POINT('Ctrl Pts',(4.1006262898548,0.0560640559726493,3.09201395474132));
#21207=CARTESIAN_POINT('Ctrl Pts',(4.07990169691163,0.0146335669363464,
3.08202325217412));
#21208=CARTESIAN_POINT('Ctrl Pts',(4.07990169691163,0.0146335669363464,
3.08620381196858));
#21209=CARTESIAN_POINT('Ctrl Pts',(4.08016324468958,0.0146335669363467,
3.09037607507745));
#21210=CARTESIAN_POINT('Ctrl Pts',(4.08068532880797,0.0146335669363467,
3.09452390684458));
#21211=CARTESIAN_POINT('Ctrl Pts',(4.03795195802051,-4.05341230270309E-17,
3.08202325217412));
#21212=CARTESIAN_POINT('Ctrl Pts',(4.03795195802051,-4.05341230270405E-17,
3.08795342935058));
#21213=CARTESIAN_POINT('Ctrl Pts',(4.03832341566108,4.19890745630692E-16,
3.09387899684106));
#21214=CARTESIAN_POINT('Ctrl Pts',(4.03906399861534,4.17432874630846E-16,
3.09976274889499));
#21215=CARTESIAN_POINT('Ctrl Pts',(4.02,-4.16333634234434E-17,3.08202325217412));
#21216=CARTESIAN_POINT('Ctrl Pts',(4.02,-4.16333634234529E-17,3.08870115571451));
#21217=CARTESIAN_POINT('Ctrl Pts',(4.02041861785905,4.18789509235301E-16,
3.0953790325586));
#21218=CARTESIAN_POINT('Ctrl Pts',(4.0212525797096,4.16333634234434E-16,
3.10200465730851));
#21219=CARTESIAN_POINT('',(4.10062628985479,0.08,3.09201395474128));
#21220=CARTESIAN_POINT('Origin',(4.0212525797096,0.08,3.10200465730851));
#21221=CARTESIAN_POINT('Origin',(4.18002609111314,0.08,3.08202161659353));
#21222=CARTESIAN_POINT('Ctrl Pts',(4.1006262898548,0.08,3.09201395474132));
#21223=CARTESIAN_POINT('Ctrl Pts',(4.11526689217912,0.08,3.20832999131892));
#21224=CARTESIAN_POINT('Ctrl Pts',(4.13379447775995,0.08,3.32356514996729));
#21225=CARTESIAN_POINT('Ctrl Pts',(4.15877532388868,0.08,3.43678097322386));
#21226=CARTESIAN_POINT('Ctrl Pts',(4.1006262898548,0.0560640559726493,3.09201395474132));
#21227=CARTESIAN_POINT('Ctrl Pts',(4.1152661626389,0.0560640559726493,3.20832419529872));
#21228=CARTESIAN_POINT('Ctrl Pts',(4.13379661763211,0.0560640559726492,
3.32357484809309));
#21229=CARTESIAN_POINT('Ctrl Pts',(4.15877532388868,0.0560640559726492,
3.43678097322386));
#21230=CARTESIAN_POINT('Ctrl Pts',(4.08068487271943,0.0146341184962319,
3.09452396425207));
#21231=CARTESIAN_POINT('Ctrl Pts',(4.09538301420591,0.0146341184962319,
3.2112971355255));
#21232=CARTESIAN_POINT('Ctrl Pts',(4.11399903223575,0.0146341184962314,
3.32713084077746));
#21233=CARTESIAN_POINT('Ctrl Pts',(4.13914865103515,0.0146341184962313,
3.44111155953654));
#21234=CARTESIAN_POINT('Ctrl Pts',(4.03906399861534,4.45188450246475E-16,
3.09976274889499));
#21235=CARTESIAN_POINT('Ctrl Pts',(4.05388175816077,4.47436389483802E-16,
3.2174862566513));
#21236=CARTESIAN_POINT('Ctrl Pts',(4.07268421775703,-1.58819587495572E-16,
3.33457931569976));
#21237=CARTESIAN_POINT('Ctrl Pts',(4.09818469775272,-1.65434213297361E-16,
3.45015017431968));
#21238=CARTESIAN_POINT('Ctrl Pts',(4.02125257970961,4.44089209850063E-16,
3.10200465730851));
#21239=CARTESIAN_POINT('Ctrl Pts',(4.03612145990415,4.46335323570744E-16,
3.22013430623041));
#21240=CARTESIAN_POINT('Ctrl Pts',(4.0550039783989,-1.5992419952717E-16,
3.33776776889323));
#21241=CARTESIAN_POINT('Ctrl Pts',(4.08065440441665,-1.66533453693773E-16,
3.45401819866313));
#21242=CARTESIAN_POINT('',(4.15877532388652,0.0799994042033401,3.43678097322434));
#21243=CARTESIAN_POINT('Origin',(4.08065440441665,0.08,3.45401819866313));
#21244=CARTESIAN_POINT('Ctrl Pts',(4.1006262898548,0.08,3.09201395474132));
#21245=CARTESIAN_POINT('Ctrl Pts',(4.11526645524359,0.08,3.20832651997201));
#21246=CARTESIAN_POINT('Ctrl Pts',(4.13379337188534,0.08,3.32355827178816));
#21247=CARTESIAN_POINT('Ctrl Pts',(4.15877308731365,0.08,3.43677083674693));
#21248=CARTESIAN_POINT('Ctrl Pts',(4.17250638811433,0.0648543434789084,
3.48546348151857));
#21249=CARTESIAN_POINT('Ctrl Pts',(4.18266052260979,0.0556405700559915,
3.51444097567126));
#21250=CARTESIAN_POINT('Ctrl Pts',(4.20433589890911,0.0406236453241535,
3.56000713380897));
#21251=CARTESIAN_POINT('Ctrl Pts',(4.25199456808014,0.0336163065688034,
3.59330578207307));
#21252=CARTESIAN_POINT('Ctrl Pts',(4.27729012420774,0.0439150199095526,
3.57845771566606));
#21253=CARTESIAN_POINT('Ctrl Pts',(4.28625335961854,0.0503448666167723,
3.56616535738233));
#21254=CARTESIAN_POINT('Ctrl Pts',(4.16929027892073,0.0467828333657603,
3.48680406174265));
#21255=CARTESIAN_POINT('Ctrl Pts',(4.17796988891339,0.0397461385215758,
3.51697746443788));
#21256=CARTESIAN_POINT('Ctrl Pts',(4.1988611271974,0.0290109791845337,3.56548110876311));
#21257=CARTESIAN_POINT('Ctrl Pts',(4.25263440860521,0.0269453546316361,
3.60149225779319));
#21258=CARTESIAN_POINT('Ctrl Pts',(4.28279509833513,0.036739599270244,3.58519594631708));
#21259=CARTESIAN_POINT('Ctrl Pts',(4.29328883703346,0.0422568691806583,
3.57193401843471));
#21260=CARTESIAN_POINT('Ctrl Pts',(4.15087621691878,0.013238281675356,3.49447964919285));
#21261=CARTESIAN_POINT('Ctrl Pts',(4.16005024766761,0.0114887305890716,
3.52731328970503));
#21262=CARTESIAN_POINT('Ctrl Pts',(4.1844192175266,0.00938090938160887,
3.58082600653567));
#21263=CARTESIAN_POINT('Ctrl Pts',(4.25361565342529,0.0161067146530447,
3.62047517370959));
#21264=CARTESIAN_POINT('Ctrl Pts',(4.29453368233821,0.0258216733838189,
3.60185180708036));
#21265=CARTESIAN_POINT('Ctrl Pts',(4.30919086234588,0.0301620716842713,
3.58693685155031));
#21266=CARTESIAN_POINT('Ctrl Pts',(4.11698762514124,1.35575488646911E-14,
3.50860553025727));
#21267=CARTESIAN_POINT('Ctrl Pts',(4.1313452462753,0.000358144080936645,
3.54413845042102));
#21268=CARTESIAN_POINT('Ctrl Pts',(4.16538066436182,0.00107821606618538,
3.60111646091567));
#21269=CARTESIAN_POINT('Ctrl Pts',(4.25343337329451,0.0118887454562876,
3.64233796301702));
#21270=CARTESIAN_POINT('Ctrl Pts',(4.30590173066008,0.0236297726512944,
3.62199161527088));
#21271=CARTESIAN_POINT('Ctrl Pts',(4.325507636067,0.0286760266021307,3.6057994627788));
#21272=CARTESIAN_POINT('Ctrl Pts',(4.10000000000067,1.11022302462516E-15,
3.51568653184854));
#21273=CARTESIAN_POINT('Ctrl Pts',(4.11687019564162,1.39427594163973E-14,
3.55256131194227));
#21274=CARTESIAN_POINT('Ctrl Pts',(4.15558369197843,0.000126613028484238,
3.61126292396189));
#21275=CARTESIAN_POINT('Ctrl Pts',(4.25303821911669,0.0114738356156513,
3.65326412679659));
#21276=CARTESIAN_POINT('Ctrl Pts',(4.31105117291262,0.0248024289745047,
3.63206334799651));
#21277=CARTESIAN_POINT('Ctrl Pts',(4.33293714059217,0.0306667563398109,
3.61523506307459));
#21278=CARTESIAN_POINT('',(4.17250638811433,0.0648543434789084,3.48546348151857));
#21279=CARTESIAN_POINT('Origin',(4.10000000000061,0.0800000000000007,3.51568653184854));
#21280=CARTESIAN_POINT('',(4.28625335961854,0.0503448666167723,3.56616535738233));
#21281=CARTESIAN_POINT('Ctrl Pts',(4.17250638811433,0.0648543434789084,
3.48546348151857));
#21282=CARTESIAN_POINT('Ctrl Pts',(4.18266052260979,0.0556405700559915,
3.51444097567126));
#21283=CARTESIAN_POINT('Ctrl Pts',(4.20433589890911,0.0406236453241535,
3.56000713380897));
#21284=CARTESIAN_POINT('Ctrl Pts',(4.25199456808014,0.0336163065688034,
3.59330578207307));
#21285=CARTESIAN_POINT('Ctrl Pts',(4.27729012420774,0.0439150199095526,
3.57845771566606));
#21286=CARTESIAN_POINT('Ctrl Pts',(4.28625335961854,0.0503448666167723,
3.56616535738233));
#21287=CARTESIAN_POINT('Origin',(4.31223161698397,0.107940822442937,3.6152350630746));
#21288=CARTESIAN_POINT('Ctrl Pts',(4.15877532388868,0.0800000000000003,
3.43678097322386));
#21289=CARTESIAN_POINT('Ctrl Pts',(4.16246506407796,0.0749031082315837,
3.45350326401334));
#21290=CARTESIAN_POINT('Ctrl Pts',(4.16702335990291,0.069829595641864,3.46981621803132));
#21291=CARTESIAN_POINT('Ctrl Pts',(4.17250638811433,0.064854343478907,3.48546348151857));
#21292=CARTESIAN_POINT('Ctrl Pts',(4.15877532388868,0.0560640559726496,
3.43678097322386));
#21293=CARTESIAN_POINT('Ctrl Pts',(4.16092731617209,0.0519427537625869,
3.45382800899325));
#21294=CARTESIAN_POINT('Ctrl Pts',(4.16431986899145,0.0479680589322419,
3.47067724603867));
#21295=CARTESIAN_POINT('Ctrl Pts',(4.16883083475021,0.0442011890638705,
3.48699557320324));
#21296=CARTESIAN_POINT('Ctrl Pts',(4.13914860105817,0.0146341799039232,
3.44111157056385));
#21297=CARTESIAN_POINT('Ctrl Pts',(4.14071345514682,0.0133927789551764,
3.45945075426926));
#21298=CARTESIAN_POINT('Ctrl Pts',(4.14379087487777,0.0122539493399985,
3.4777024640668));
#21299=CARTESIAN_POINT('Ctrl Pts',(4.14857154686496,0.0111913457409417,
3.49544031156815));
#21300=CARTESIAN_POINT('Ctrl Pts',(4.09818469775272,5.82845227735974E-16,
3.45015017431968));
#21301=CARTESIAN_POINT('Ctrl Pts',(4.10191329035582,1.31426440172898E-5,
3.47039859381559));
#21302=CARTESIAN_POINT('Ctrl Pts',(4.10731252271732,-7.72394405668259E-6,
3.49035786986458));
#21303=CARTESIAN_POINT('Ctrl Pts',(4.11456082154968,8.4635003401468E-17,
3.50961710191317));
#21304=CARTESIAN_POINT('Ctrl Pts',(4.08065440441665,5.82867087928207E-16,
3.45401819866313));
#21305=CARTESIAN_POINT('Ctrl Pts',(4.08530246872869,6.1214364716609E-16,
3.47508371521632));
#21306=CARTESIAN_POINT('Ctrl Pts',(4.0917001731762,2.63948896849449E-16,
3.49577489293594));
#21307=CARTESIAN_POINT('Ctrl Pts',(4.10000000000061,8.32667268468867E-17,
3.51568653184854));
#21308=CARTESIAN_POINT('Origin',(4.24802043123848,0.0859220706677168,3.38337978260087));
#21309=CARTESIAN_POINT('Ctrl Pts',(4.28625335961854,0.0503448666167712,
3.56616535738233));
#21310=CARTESIAN_POINT('Ctrl Pts',(4.28883173298406,0.0521944828250372,
3.56262932516341));
#21311=CARTESIAN_POINT('Ctrl Pts',(4.29121124271805,0.0540999851939356,
3.55876018527392));
#21312=CARTESIAN_POINT('Ctrl Pts',(4.29338985935164,0.0560360920070411,
3.55463300336248));
#21313=CARTESIAN_POINT('Ctrl Pts',(4.30032431444838,0.0341688717445422,
3.5777026794871));
#21314=CARTESIAN_POINT('Ctrl Pts',(4.30358042720995,0.0355310056620428,
3.57365818981285));
#21315=CARTESIAN_POINT('Ctrl Pts',(4.30657676601693,0.0369119378047956,
3.5692595980189));
#21316=CARTESIAN_POINT('Ctrl Pts',(4.30926534633513,0.0382206091540884,
3.56457879573332));
#21317=CARTESIAN_POINT('Ctrl Pts',(4.31807813154184,0.026685296864449,3.59636386248302));
#21318=CARTESIAN_POINT('Ctrl Pts',(4.32262354005804,0.02789161406842,3.59191453262352));
#21319=CARTESIAN_POINT('Ctrl Pts',(4.32687322788778,0.029057244381936,3.58706864094837));
#21320=CARTESIAN_POINT('Ctrl Pts',(4.33079072300035,0.0300916254794634,
3.58191136456955));
#21321=CARTESIAN_POINT('Ctrl Pts',(4.33293714059217,0.0306667563398117,
3.6152350630746));
#21322=CARTESIAN_POINT('Ctrl Pts',(4.33867325889683,0.0322037446072338,
3.61039422161037));
#21323=CARTESIAN_POINT('Ctrl Pts',(4.34406623569343,0.0336487883846835,
3.60510985574939));
#21324=CARTESIAN_POINT('Ctrl Pts',(4.34909964308337,0.0349974858299939,
3.59949138964762));
#21325=CARTESIAN_POINT('',(4.29338985926344,0.0560360920135354,3.55463300342316));
#21326=CARTESIAN_POINT('Origin',(4.32839411947511,0.112271551933105,3.59949138964768));
#21327=CARTESIAN_POINT('Origin',(4.23862664689032,0.0738535158890165,3.44885235882043));
#21328=CARTESIAN_POINT('Origin',(4.32839411947511,0.112271551933102,3.59949138964768));
#21329=CARTESIAN_POINT('Origin',(4.32839411947511,0.112271551933102,3.59949138964768));
#21330=CARTESIAN_POINT('Ctrl Pts',(4.1,0.,11.9026515720695));
#21331=CARTESIAN_POINT('Ctrl Pts',(4.1,0.8496,11.9026515720695));
#21332=CARTESIAN_POINT('Ctrl Pts',(4.11686402271798,0.,11.8858809149492));
#21333=CARTESIAN_POINT('Ctrl Pts',(4.11686402271798,0.8496,11.8858809149492));
#21334=CARTESIAN_POINT('Ctrl Pts',(4.15991130277621,0.,11.842517268502));
#21335=CARTESIAN_POINT('Ctrl Pts',(4.15991130277621,0.8496,11.842517268502));
#21336=CARTESIAN_POINT('Ctrl Pts',(4.22986670297865,0.,11.7703786717735));
#21337=CARTESIAN_POINT('Ctrl Pts',(4.22986670297865,0.8496,11.7703786717735));
#21338=CARTESIAN_POINT('Ctrl Pts',(4.32906075669879,0.,11.667756621275));
#21339=CARTESIAN_POINT('Ctrl Pts',(4.32906075669879,0.8496,11.667756621275));
#21340=CARTESIAN_POINT('Ctrl Pts',(4.46255574628753,0.,11.5373242211525));
#21341=CARTESIAN_POINT('Ctrl Pts',(4.46255574628753,0.8496,11.5373242211525));
#21342=CARTESIAN_POINT('Ctrl Pts',(4.61532593596939,0.,11.4029224160728));
#21343=CARTESIAN_POINT('Ctrl Pts',(4.61532593596939,0.8496,11.4029224160728));
#21344=CARTESIAN_POINT('Ctrl Pts',(4.77596612414944,0.,11.2768795166233));
#21345=CARTESIAN_POINT('Ctrl Pts',(4.77596612414944,0.8496,11.2768795166233));
#21346=CARTESIAN_POINT('Ctrl Pts',(4.94211773226968,0.,11.1598106424589));
#21347=CARTESIAN_POINT('Ctrl Pts',(4.94211773226968,0.8496,11.1598106424589));
#21348=CARTESIAN_POINT('Ctrl Pts',(5.11112998264613,0.,11.051370419133));
#21349=CARTESIAN_POINT('Ctrl Pts',(5.11112998264613,0.8496,11.051370419133));
#21350=CARTESIAN_POINT('Ctrl Pts',(5.28082876351925,0.,10.9511663773825));
#21351=CARTESIAN_POINT('Ctrl Pts',(5.28082876351925,0.8496,10.9511663773825));
#21352=CARTESIAN_POINT('Ctrl Pts',(5.45051506148977,0.,10.8599381259735));
#21353=CARTESIAN_POINT('Ctrl Pts',(5.45051506148977,0.8496,10.8599381259735));
#21354=CARTESIAN_POINT('Ctrl Pts',(5.62101499943423,0.,10.7795199127532));
#21355=CARTESIAN_POINT('Ctrl Pts',(5.62101499943423,0.8496,10.7795199127532));
#21356=CARTESIAN_POINT('Ctrl Pts',(5.7936769541502,0.,10.7114411549111));
#21357=CARTESIAN_POINT('Ctrl Pts',(5.7936769541502,0.8496,10.7114411549111));
#21358=CARTESIAN_POINT('Ctrl Pts',(5.96961932707136,0.,10.6558377434042));
#21359=CARTESIAN_POINT('Ctrl Pts',(5.96961932707136,0.8496,10.6558377434042));
#21360=CARTESIAN_POINT('Ctrl Pts',(6.14893768388704,0.,10.6103475969888));
#21361=CARTESIAN_POINT('Ctrl Pts',(6.14893768388704,0.8496,10.6103475969888));
#21362=CARTESIAN_POINT('Ctrl Pts',(6.32976796473819,0.,10.5687216653907));
#21363=CARTESIAN_POINT('Ctrl Pts',(6.32976796473819,0.8496,10.5687216653907));
#21364=CARTESIAN_POINT('Ctrl Pts',(6.50892555577775,0.,10.5222908830264));
#21365=CARTESIAN_POINT('Ctrl Pts',(6.50892555577775,0.8496,10.5222908830264));
#21366=CARTESIAN_POINT('Ctrl Pts',(6.68288828293941,0.,10.462050267878));
#21367=CARTESIAN_POINT('Ctrl Pts',(6.68288828293941,0.8496,10.462050267878));
#21368=CARTESIAN_POINT('Ctrl Pts',(6.84859008776107,0.,10.3804015453596));
#21369=CARTESIAN_POINT('Ctrl Pts',(6.84859008776107,0.8496,10.3804015453596));
#21370=CARTESIAN_POINT('Ctrl Pts',(7.00445448641038,0.,10.2733319413005));
#21371=CARTESIAN_POINT('Ctrl Pts',(7.00445448641038,0.8496,10.2733319413005));
#21372=CARTESIAN_POINT('Ctrl Pts',(7.15081550722288,0.,10.1414720974144));
#21373=CARTESIAN_POINT('Ctrl Pts',(7.15081550722288,0.8496,10.1414720974144));
#21374=CARTESIAN_POINT('Ctrl Pts',(7.28883796912684,0.,9.98835756998534));
#21375=CARTESIAN_POINT('Ctrl Pts',(7.28883796912684,0.8496,9.98835756998534));
#21376=CARTESIAN_POINT('Ctrl Pts',(7.41967047354988,0.,9.81917361987377));
#21377=CARTESIAN_POINT('Ctrl Pts',(7.41967047354988,0.8496,9.81917361987377));
#21378=CARTESIAN_POINT('Ctrl Pts',(7.54360573526532,0.,9.63939026966049));
#21379=CARTESIAN_POINT('Ctrl Pts',(7.54360573526532,0.8496,9.63939026966049));
#21380=CARTESIAN_POINT('Ctrl Pts',(7.6590003866074,0.,9.45324999450471));
#21381=CARTESIAN_POINT('Ctrl Pts',(7.6590003866074,0.8496,9.45324999450471));
#21382=CARTESIAN_POINT('Ctrl Pts',(7.76209282457502,0.,9.26297089919836));
#21383=CARTESIAN_POINT('Ctrl Pts',(7.76209282457502,0.8496,9.26297089919836));
#21384=CARTESIAN_POINT('Ctrl Pts',(7.84862074946283,0.,9.06945407017055));
#21385=CARTESIAN_POINT('Ctrl Pts',(7.84862074946283,0.8496,9.06945407017055));
#21386=CARTESIAN_POINT('Ctrl Pts',(7.91508259073031,0.,8.87266947141857));
#21387=CARTESIAN_POINT('Ctrl Pts',(7.91508259073031,0.8496,8.87266947141857));
#21388=CARTESIAN_POINT('Ctrl Pts',(7.96007609558387,0.,8.67216210283894));
#21389=CARTESIAN_POINT('Ctrl Pts',(7.96007609558387,0.8496,8.67216210283894));
#21390=CARTESIAN_POINT('Ctrl Pts',(7.98575825096082,0.,8.46752658699496));
#21391=CARTESIAN_POINT('Ctrl Pts',(7.98575825096082,0.8496,8.46752658699496));
#21392=CARTESIAN_POINT('Ctrl Pts',(7.9987984391963,0.,8.25883677791438));
#21393=CARTESIAN_POINT('Ctrl Pts',(7.9987984391963,0.8496,8.25883677791438));
#21394=CARTESIAN_POINT('Ctrl Pts',(8.00781893805568,0.,8.04662057355209));
#21395=CARTESIAN_POINT('Ctrl Pts',(8.00781893805568,0.8496,8.04662057355209));
#21396=CARTESIAN_POINT('Ctrl Pts',(8.02124364536257,0.,7.8318867323277));
#21397=CARTESIAN_POINT('Ctrl Pts',(8.02124364536257,0.8496,7.8318867323277));
#21398=CARTESIAN_POINT('Ctrl Pts',(8.04494633492827,0.,7.61613341658679));
#21399=CARTESIAN_POINT('Ctrl Pts',(8.04494633492827,0.8496,7.61613341658679));
#21400=CARTESIAN_POINT('Ctrl Pts',(8.08008348678094,0.,7.40136016279815));
#21401=CARTESIAN_POINT('Ctrl Pts',(8.08008348678094,0.8496,7.40136016279815));
#21402=CARTESIAN_POINT('Ctrl Pts',(8.12057943633426,0.,7.19009032473197));
#21403=CARTESIAN_POINT('Ctrl Pts',(8.12057943633426,0.8496,7.19009032473197));
#21404=CARTESIAN_POINT('Ctrl Pts',(8.15569042861283,0.,6.98516923427904));
#21405=CARTESIAN_POINT('Ctrl Pts',(8.15569042861283,0.8496,6.98516923427904));
#21406=CARTESIAN_POINT('Ctrl Pts',(8.17293082304204,0.,6.78954489191915));
#21407=CARTESIAN_POINT('Ctrl Pts',(8.17293082304204,0.8496,6.78954489191915));
#21408=CARTESIAN_POINT('Ctrl Pts',(8.16089752265956,0.,6.60605451948904));
#21409=CARTESIAN_POINT('Ctrl Pts',(8.16089752265956,0.8496,6.60605451948904));
#21410=CARTESIAN_POINT('Ctrl Pts',(8.11207116917844,0.,6.43720976255638));
#21411=CARTESIAN_POINT('Ctrl Pts',(8.11207116917844,0.8496,6.43720976255638));
#21412=CARTESIAN_POINT('Ctrl Pts',(8.02580908828092,0.,6.28498018271691));
#21413=CARTESIAN_POINT('Ctrl Pts',(8.02580908828092,0.8496,6.28498018271691));
#21414=CARTESIAN_POINT('Ctrl Pts',(7.90644860448881,0.,6.15052660592943));
#21415=CARTESIAN_POINT('Ctrl Pts',(7.90644860448881,0.8496,6.15052660592943));
#21416=CARTESIAN_POINT('Ctrl Pts',(7.76106756457749,0.,6.03389995867286));
#21417=CARTESIAN_POINT('Ctrl Pts',(7.76106756457749,0.8496,6.03389995867286));
#21418=CARTESIAN_POINT('Ctrl Pts',(7.59751903688427,0.,5.93381436957244));
#21419=CARTESIAN_POINT('Ctrl Pts',(7.59751903688427,0.8496,5.93381436957244));
#21420=CARTESIAN_POINT('Ctrl Pts',(7.42198551710643,0.,5.84723737025948));
#21421=CARTESIAN_POINT('Ctrl Pts',(7.42198551710643,0.8496,5.84723737025948));
#21422=CARTESIAN_POINT('Ctrl Pts',(7.23853768475023,0.,5.76979878895671));
#21423=CARTESIAN_POINT('Ctrl Pts',(7.23853768475023,0.8496,5.76979878895671));
#21424=CARTESIAN_POINT('Ctrl Pts',(7.04976847947264,0.,5.69662713609756));
#21425=CARTESIAN_POINT('Ctrl Pts',(7.04976847947264,0.8496,5.69662713609756));
#21426=CARTESIAN_POINT('Ctrl Pts',(6.85709976037512,0.,5.62308582598972));
#21427=CARTESIAN_POINT('Ctrl Pts',(6.85709976037512,0.8496,5.62308582598972));
#21428=CARTESIAN_POINT('Ctrl Pts',(6.66121503090593,0.,5.54547963906641));
#21429=CARTESIAN_POINT('Ctrl Pts',(6.66121503090593,0.8496,5.54547963906641));
#21430=CARTESIAN_POINT('Ctrl Pts',(6.46246210121974,0.,5.46195513100458));
#21431=CARTESIAN_POINT('Ctrl Pts',(6.46246210121974,0.8496,5.46195513100458));
#21432=CARTESIAN_POINT('Ctrl Pts',(6.26112587698791,0.,5.37226655127806));
#21433=CARTESIAN_POINT('Ctrl Pts',(6.26112587698791,0.8496,5.37226655127806));
#21434=CARTESIAN_POINT('Ctrl Pts',(6.05762450882876,0.,5.27709955371581));
#21435=CARTESIAN_POINT('Ctrl Pts',(6.05762450882876,0.8496,5.27709955371581));
#21436=CARTESIAN_POINT('Ctrl Pts',(5.85274048349253,0.,5.17752467829117));
#21437=CARTESIAN_POINT('Ctrl Pts',(5.85274048349253,0.8496,5.17752467829117));
#21438=CARTESIAN_POINT('Ctrl Pts',(5.6478173738032,0.,5.07442896098936));
#21439=CARTESIAN_POINT('Ctrl Pts',(5.6478173738032,0.8496,5.07442896098936));
#21440=CARTESIAN_POINT('Ctrl Pts',(5.44501860313336,0.,4.96787993373722));
#21441=CARTESIAN_POINT('Ctrl Pts',(5.44501860313336,0.8496,4.96787993373722));
#21442=CARTESIAN_POINT('Ctrl Pts',(5.24741086000008,0.,4.85676111532844));
#21443=CARTESIAN_POINT('Ctrl Pts',(5.24741086000008,0.8496,4.85676111532844));
#21444=CARTESIAN_POINT('Ctrl Pts',(5.05850630701875,0.,4.73929437247794));
#21445=CARTESIAN_POINT('Ctrl Pts',(5.05850630701875,0.8496,4.73929437247794));
#21446=CARTESIAN_POINT('Ctrl Pts',(4.88190185104846,0.,4.61340315498245));
#21447=CARTESIAN_POINT('Ctrl Pts',(4.88190185104846,0.8496,4.61340315498245));
#21448=CARTESIAN_POINT('Ctrl Pts',(4.7208720035032,0.,4.47714872481864));
#21449=CARTESIAN_POINT('Ctrl Pts',(4.7208720035032,0.8496,4.47714872481864));
#21450=CARTESIAN_POINT('Ctrl Pts',(4.57800047823784,0.,4.32911151507775));
#21451=CARTESIAN_POINT('Ctrl Pts',(4.57800047823784,0.8496,4.32911151507775));
#21452=CARTESIAN_POINT('Ctrl Pts',(4.4547451964031,0.,4.16885849319143));
#21453=CARTESIAN_POINT('Ctrl Pts',(4.4547451964031,0.8496,4.16885849319143));
#21454=CARTESIAN_POINT('Ctrl Pts',(4.35148411330737,0.,3.99681013615577));
#21455=CARTESIAN_POINT('Ctrl Pts',(4.35148411330737,0.8496,3.99681013615577));
#21456=CARTESIAN_POINT('Ctrl Pts',(4.26765207024408,0.,3.81399668859083));
#21457=CARTESIAN_POINT('Ctrl Pts',(4.26765207024408,0.8496,3.81399668859083));
#21458=CARTESIAN_POINT('Ctrl Pts',(4.20184334854117,0.,3.62185203209172));
#21459=CARTESIAN_POINT('Ctrl Pts',(4.20184334854117,0.8496,3.62185203209172));
#21460=CARTESIAN_POINT('Ctrl Pts',(4.15193466045737,0.,3.42199345348454));
#21461=CARTESIAN_POINT('Ctrl Pts',(4.15193466045737,0.8496,3.42199345348454));
#21462=CARTESIAN_POINT('Ctrl Pts',(4.11518318246501,0.,3.21600287470933));
#21463=CARTESIAN_POINT('Ctrl Pts',(4.11518318246501,0.8496,3.21600287470933));
#21464=CARTESIAN_POINT('Ctrl Pts',(4.08854433447712,0.,3.00529120729351));
#21465=CARTESIAN_POINT('Ctrl Pts',(4.08854433447712,0.8496,3.00529120729351));
#21466=CARTESIAN_POINT('Ctrl Pts',(4.06899962712481,0.,2.7909834104826));
#21467=CARTESIAN_POINT('Ctrl Pts',(4.06899962712481,0.8496,2.7909834104826));
#21468=CARTESIAN_POINT('Ctrl Pts',(4.05390260344518,0.,2.57377631141663));
#21469=CARTESIAN_POINT('Ctrl Pts',(4.05390260344518,0.8496,2.57377631141663));
#21470=CARTESIAN_POINT('Ctrl Pts',(4.04126813644791,0.,2.35385258470204));
#21471=CARTESIAN_POINT('Ctrl Pts',(4.04126813644791,0.8496,2.35385258470204));
#21472=CARTESIAN_POINT('Ctrl Pts',(4.03021014446877,0.,2.13065748555701));
#21473=CARTESIAN_POINT('Ctrl Pts',(4.03021014446877,0.8496,2.13065748555701));
#21474=CARTESIAN_POINT('Ctrl Pts',(4.02066709528519,0.,1.9033255681334));
#21475=CARTESIAN_POINT('Ctrl Pts',(4.02066709528519,0.8496,1.9033255681334));
#21476=CARTESIAN_POINT('Ctrl Pts',(4.012782399266,0.,1.67142113207676));
#21477=CARTESIAN_POINT('Ctrl Pts',(4.012782399266,0.8496,1.67142113207676));
#21478=CARTESIAN_POINT('Ctrl Pts',(4.00639322616619,0.,1.4355810193293));
#21479=CARTESIAN_POINT('Ctrl Pts',(4.00639322616619,0.8496,1.4355810193293));
#21480=CARTESIAN_POINT('Ctrl Pts',(4.00047520099043,0.,1.19819542279832));
#21481=CARTESIAN_POINT('Ctrl Pts',(4.00047520099043,0.8496,1.19819542279832));
#21482=CARTESIAN_POINT('Ctrl Pts',(3.99260375067002,0.,0.964078729991153));
#21483=CARTESIAN_POINT('Ctrl Pts',(3.99260375067002,0.8496,0.964078729991153));
#21484=CARTESIAN_POINT('Ctrl Pts',(3.97841403016118,0.,0.741129277895168));
#21485=CARTESIAN_POINT('Ctrl Pts',(3.97841403016118,0.8496,0.741129277895168));
#21486=CARTESIAN_POINT('Ctrl Pts',(3.95259200169988,0.,0.538436816836329));
#21487=CARTESIAN_POINT('Ctrl Pts',(3.95259200169988,0.8496,0.538436816836329));
#21488=CARTESIAN_POINT('Ctrl Pts',(3.90986572419832,0.,0.364350357241537));
#21489=CARTESIAN_POINT('Ctrl Pts',(3.90986572419832,0.8496,0.364350357241537));
#21490=CARTESIAN_POINT('Ctrl Pts',(3.84598208672298,0.,0.224659532804428));
#21491=CARTESIAN_POINT('Ctrl Pts',(3.84598208672298,0.8496,0.224659532804428));
#21492=CARTESIAN_POINT('Ctrl Pts',(3.75872318140661,0.,0.120497232333236));
#21493=CARTESIAN_POINT('Ctrl Pts',(3.75872318140661,0.8496,0.120497232333236));
#21494=CARTESIAN_POINT('Ctrl Pts',(3.64881642260075,0.,0.0470540298718229));
#21495=CARTESIAN_POINT('Ctrl Pts',(3.64881642260075,0.8496,0.0470540298718229));
#21496=CARTESIAN_POINT('Ctrl Pts',(3.52045328348988,0.,-0.00118366394786523));
#21497=CARTESIAN_POINT('Ctrl Pts',(3.52045328348988,0.8496,-0.00118366394786523));
#21498=CARTESIAN_POINT('Ctrl Pts',(3.3816469894381,0.,-0.0263068037111615));
#21499=CARTESIAN_POINT('Ctrl Pts',(3.3816469894381,0.8496,-0.0263068037111615));
#21500=CARTESIAN_POINT('Ctrl Pts',(3.2451100102617,0.,-0.0214179570895094));
#21501=CARTESIAN_POINT('Ctrl Pts',(3.2451100102617,0.8496,-0.0214179570895094));
#21502=CARTESIAN_POINT('Ctrl Pts',(3.12452733970665,0.,0.0241851999814078));
#21503=CARTESIAN_POINT('Ctrl Pts',(3.12452733970665,0.8496,0.0241851999814078));
#21504=CARTESIAN_POINT('Ctrl Pts',(3.03063129752059,0.,0.119017371327004));
#21505=CARTESIAN_POINT('Ctrl Pts',(3.03063129752059,0.8496,0.119017371327004));
#21506=CARTESIAN_POINT('Ctrl Pts',(2.96639254265844,0.,0.262319630540593));
#21507=CARTESIAN_POINT('Ctrl Pts',(2.96639254265844,0.8496,0.262319630540593));
#21508=CARTESIAN_POINT('Ctrl Pts',(2.92780415844446,0.,0.444963858672424));
#21509=CARTESIAN_POINT('Ctrl Pts',(2.92780415844446,0.8496,0.444963858672424));
#21510=CARTESIAN_POINT('Ctrl Pts',(2.90717911786689,0.,0.65402023086958));
#21511=CARTESIAN_POINT('Ctrl Pts',(2.90717911786689,0.8496,0.65402023086958));
#21512=CARTESIAN_POINT('Ctrl Pts',(2.89547076625581,0.,0.875890304828918));
#21513=CARTESIAN_POINT('Ctrl Pts',(2.89547076625581,0.8496,0.875890304828918));
#21514=CARTESIAN_POINT('Ctrl Pts',(2.88537704766906,0.,1.10060381648398));
#21515=CARTESIAN_POINT('Ctrl Pts',(2.88537704766906,0.8496,1.10060381648398));
#21516=CARTESIAN_POINT('Ctrl Pts',(2.8728456296504,0.,1.32371934078733));
#21517=CARTESIAN_POINT('Ctrl Pts',(2.8728456296504,0.8496,1.32371934078733));
#21518=CARTESIAN_POINT('Ctrl Pts',(2.85578261679345,0.,1.54401727992264));
#21519=CARTESIAN_POINT('Ctrl Pts',(2.85578261679345,0.8496,1.54401727992264));
#21520=CARTESIAN_POINT('Ctrl Pts',(2.83335686249019,0.,1.76209503442146));
#21521=CARTESIAN_POINT('Ctrl Pts',(2.83335686249019,0.8496,1.76209503442146));
#21522=CARTESIAN_POINT('Ctrl Pts',(2.80505146480345,0.,1.97856787413951));
#21523=CARTESIAN_POINT('Ctrl Pts',(2.80505146480345,0.8496,1.97856787413951));
#21524=CARTESIAN_POINT('Ctrl Pts',(2.76985908233915,0.,2.19251877196071));
#21525=CARTESIAN_POINT('Ctrl Pts',(2.76985908233915,0.8496,2.19251877196071));
#21526=CARTESIAN_POINT('Ctrl Pts',(2.72531955636536,0.,2.39962532458029));
#21527=CARTESIAN_POINT('Ctrl Pts',(2.72531955636536,0.8496,2.39962532458029));
#21528=CARTESIAN_POINT('Ctrl Pts',(2.66797634363184,0.,2.59347738935741));
#21529=CARTESIAN_POINT('Ctrl Pts',(2.66797634363184,0.8496,2.59347738935741));
#21530=CARTESIAN_POINT('Ctrl Pts',(2.59397540849171,0.,2.7672283971178));
#21531=CARTESIAN_POINT('Ctrl Pts',(2.59397540849171,0.8496,2.7672283971178));
#21532=CARTESIAN_POINT('Ctrl Pts',(2.49960870420485,0.,2.91510580081997));
#21533=CARTESIAN_POINT('Ctrl Pts',(2.49960870420485,0.8496,2.91510580081997));
#21534=CARTESIAN_POINT('Ctrl Pts',(2.38189256086504,0.,3.03403241435618));
#21535=CARTESIAN_POINT('Ctrl Pts',(2.38189256086504,0.8496,3.03403241435618));
#21536=CARTESIAN_POINT('Ctrl Pts',(2.23909845280558,0.,3.12505646843308));
#21537=CARTESIAN_POINT('Ctrl Pts',(2.23909845280558,0.8496,3.12505646843308));
#21538=CARTESIAN_POINT('Ctrl Pts',(2.07061055216582,0.,3.19196918412265));
#21539=CARTESIAN_POINT('Ctrl Pts',(2.07061055216582,0.8496,3.19196918412265));
#21540=CARTESIAN_POINT('Ctrl Pts',(1.87681490437036,0.,3.24001322621211));
#21541=CARTESIAN_POINT('Ctrl Pts',(1.87681490437036,0.8496,3.24001322621211));
#21542=CARTESIAN_POINT('Ctrl Pts',(1.65897747541321,0.,3.27464765209773));
#21543=CARTESIAN_POINT('Ctrl Pts',(1.65897747541321,0.8496,3.27464765209773));
#21544=CARTESIAN_POINT('Ctrl Pts',(1.4191255439272,0.,3.30006519349576));
#21545=CARTESIAN_POINT('Ctrl Pts',(1.4191255439272,0.8496,3.30006519349576));
#21546=CARTESIAN_POINT('Ctrl Pts',(1.15993538533448,0.,3.31897283641381));
#21547=CARTESIAN_POINT('Ctrl Pts',(1.15993538533448,0.8496,3.31897283641381));
#21548=CARTESIAN_POINT('Ctrl Pts',(0.884625090385968,0.,3.33300441174764));
#21549=CARTESIAN_POINT('Ctrl Pts',(0.884625090385968,0.8496,3.33300441174764));
#21550=CARTESIAN_POINT('Ctrl Pts',(0.596845720618978,0.,3.34293392264922));
#21551=CARTESIAN_POINT('Ctrl Pts',(0.596845720618978,0.8496,3.34293392264922));
#21552=CARTESIAN_POINT('Ctrl Pts',(0.30057321210183,0.,3.34897162637417));
#21553=CARTESIAN_POINT('Ctrl Pts',(0.30057321210183,0.8496,3.34897162637417));
#21554=CARTESIAN_POINT('Ctrl Pts',(1.66741620510891E-14,0.,3.35102435732185));
#21555=CARTESIAN_POINT('Ctrl Pts',(1.66741620510891E-14,0.8496,3.35102435732185));
#21556=CARTESIAN_POINT('Ctrl Pts',(-0.300573212101791,0.,3.34897162637426));
#21557=CARTESIAN_POINT('Ctrl Pts',(-0.300573212101791,0.8496,3.34897162637426));
#21558=CARTESIAN_POINT('Ctrl Pts',(-0.596845720618908,0.,3.34293392264938));
#21559=CARTESIAN_POINT('Ctrl Pts',(-0.596845720618908,0.8496,3.34293392264938));
#21560=CARTESIAN_POINT('Ctrl Pts',(-0.884625090385886,0.,3.33300441174785));
#21561=CARTESIAN_POINT('Ctrl Pts',(-0.884625090385886,0.8496,3.33300441174785));
#21562=CARTESIAN_POINT('Ctrl Pts',(-1.15993538533442,0.,3.31897283641402));
#21563=CARTESIAN_POINT('Ctrl Pts',(-1.15993538533442,0.8496,3.31897283641402));
#21564=CARTESIAN_POINT('Ctrl Pts',(-1.41912554392716,0.,3.30006519349591));
#21565=CARTESIAN_POINT('Ctrl Pts',(-1.41912554392716,0.8496,3.30006519349591));
#21566=CARTESIAN_POINT('Ctrl Pts',(-1.65897747541319,0.,3.27464765209779));
#21567=CARTESIAN_POINT('Ctrl Pts',(-1.65897747541319,0.8496,3.27464765209779));
#21568=CARTESIAN_POINT('Ctrl Pts',(-1.87681490437034,0.,3.24001322621208));
#21569=CARTESIAN_POINT('Ctrl Pts',(-1.87681490437034,0.8496,3.24001322621208));
#21570=CARTESIAN_POINT('Ctrl Pts',(-2.07061055216576,0.,3.19196918412254));
#21571=CARTESIAN_POINT('Ctrl Pts',(-2.07061055216576,0.8496,3.19196918412254));
#21572=CARTESIAN_POINT('Ctrl Pts',(-2.23909845280547,0.,3.12505646843295));
#21573=CARTESIAN_POINT('Ctrl Pts',(-2.23909845280547,0.8496,3.12505646843295));
#21574=CARTESIAN_POINT('Ctrl Pts',(-2.38189256086493,0.,3.03403241435609));
#21575=CARTESIAN_POINT('Ctrl Pts',(-2.38189256086493,0.8496,3.03403241435609));
#21576=CARTESIAN_POINT('Ctrl Pts',(-2.49960870420481,0.,2.91510580081997));
#21577=CARTESIAN_POINT('Ctrl Pts',(-2.49960870420481,0.8496,2.91510580081997));
#21578=CARTESIAN_POINT('Ctrl Pts',(-2.59397540849182,0.,2.76722839711793));
#21579=CARTESIAN_POINT('Ctrl Pts',(-2.59397540849182,0.8496,2.76722839711793));
#21580=CARTESIAN_POINT('Ctrl Pts',(-2.66797634363209,0.,2.59347738935767));
#21581=CARTESIAN_POINT('Ctrl Pts',(-2.66797634363209,0.8496,2.59347738935767));
#21582=CARTESIAN_POINT('Ctrl Pts',(-2.72531955636566,0.,2.39962532458057));
#21583=CARTESIAN_POINT('Ctrl Pts',(-2.72531955636566,0.8496,2.39962532458057));
#21584=CARTESIAN_POINT('Ctrl Pts',(-2.76985908233936,0.,2.19251877196088));
#21585=CARTESIAN_POINT('Ctrl Pts',(-2.76985908233936,0.8496,2.19251877196088));
#21586=CARTESIAN_POINT('Ctrl Pts',(-2.80505146480344,0.,1.97856787413951));
#21587=CARTESIAN_POINT('Ctrl Pts',(-2.80505146480344,0.8496,1.97856787413951));
#21588=CARTESIAN_POINT('Ctrl Pts',(-2.8333568624899,0.,1.76209503442131));
#21589=CARTESIAN_POINT('Ctrl Pts',(-2.8333568624899,0.8496,1.76209503442131));
#21590=CARTESIAN_POINT('Ctrl Pts',(-2.85578261679294,0.,1.54401727992238));
#21591=CARTESIAN_POINT('Ctrl Pts',(-2.85578261679294,0.8496,1.54401727992238));
#21592=CARTESIAN_POINT('Ctrl Pts',(-2.87284562964987,0.,1.32371934078708));
#21593=CARTESIAN_POINT('Ctrl Pts',(-2.87284562964987,0.8496,1.32371934078708));
#21594=CARTESIAN_POINT('Ctrl Pts',(-2.88537704766869,0.,1.10060381648384));
#21595=CARTESIAN_POINT('Ctrl Pts',(-2.88537704766869,0.8496,1.10060381648384));
#21596=CARTESIAN_POINT('Ctrl Pts',(-2.89547076625573,0.,0.875890304828914));
#21597=CARTESIAN_POINT('Ctrl Pts',(-2.89547076625573,0.8496,0.875890304828914));
#21598=CARTESIAN_POINT('Ctrl Pts',(-2.90717911786707,0.,0.654020230869684));
#21599=CARTESIAN_POINT('Ctrl Pts',(-2.90717911786707,0.8496,0.654020230869684));
#21600=CARTESIAN_POINT('Ctrl Pts',(-2.92780415844476,0.,0.444963858672577));
#21601=CARTESIAN_POINT('Ctrl Pts',(-2.92780415844476,0.8496,0.444963858672577));
#21602=CARTESIAN_POINT('Ctrl Pts',(-2.96639254265869,0.,0.262319630540737));
#21603=CARTESIAN_POINT('Ctrl Pts',(-2.96639254265869,0.8496,0.262319630540737));
#21604=CARTESIAN_POINT('Ctrl Pts',(-3.03063129752067,0.,0.11901737132707));
#21605=CARTESIAN_POINT('Ctrl Pts',(-3.03063129752067,0.8496,0.11901737132707));
#21606=CARTESIAN_POINT('Ctrl Pts',(-3.12452733970658,0.,0.0241851999813871));
#21607=CARTESIAN_POINT('Ctrl Pts',(-3.12452733970658,0.8496,0.0241851999813871));
#21608=CARTESIAN_POINT('Ctrl Pts',(-3.24511001026157,0.,-0.0214179570895714));
#21609=CARTESIAN_POINT('Ctrl Pts',(-3.24511001026157,0.8496,-0.0214179570895714));
#21610=CARTESIAN_POINT('Ctrl Pts',(-3.38164698943802,0.,-0.0263068037112043));
#21611=CARTESIAN_POINT('Ctrl Pts',(-3.38164698943802,0.8496,-0.0263068037112043));
#21612=CARTESIAN_POINT('Ctrl Pts',(-3.52045328348989,0.,-0.00118366394785932));
#21613=CARTESIAN_POINT('Ctrl Pts',(-3.52045328348989,0.8496,-0.00118366394785932));
#21614=CARTESIAN_POINT('Ctrl Pts',(-3.64881642260079,0.,0.0470540298718583));
#21615=CARTESIAN_POINT('Ctrl Pts',(-3.64881642260079,0.8496,0.0470540298718583));
#21616=CARTESIAN_POINT('Ctrl Pts',(-3.75872318140663,0.,0.120497232333251));
#21617=CARTESIAN_POINT('Ctrl Pts',(-3.75872318140663,0.8496,0.120497232333251));
#21618=CARTESIAN_POINT('Ctrl Pts',(-3.84598208672296,0.,0.224659532804408));
#21619=CARTESIAN_POINT('Ctrl Pts',(-3.84598208672296,0.8496,0.224659532804408));
#21620=CARTESIAN_POINT('Ctrl Pts',(-3.9098657241983,0.,0.364350357241515));
#21621=CARTESIAN_POINT('Ctrl Pts',(-3.9098657241983,0.8496,0.364350357241515));
#21622=CARTESIAN_POINT('Ctrl Pts',(-3.9525920016999,0.,0.538436816836325));
#21623=CARTESIAN_POINT('Ctrl Pts',(-3.9525920016999,0.8496,0.538436816836325));
#21624=CARTESIAN_POINT('Ctrl Pts',(-3.97841403016126,0.,0.741129277895169));
#21625=CARTESIAN_POINT('Ctrl Pts',(-3.97841403016126,0.8496,0.741129277895169));
#21626=CARTESIAN_POINT('Ctrl Pts',(-3.99260375067011,0.,0.964078729991154));
#21627=CARTESIAN_POINT('Ctrl Pts',(-3.99260375067011,0.8496,0.964078729991154));
#21628=CARTESIAN_POINT('Ctrl Pts',(-4.00047520099045,0.,1.1981954227983));
#21629=CARTESIAN_POINT('Ctrl Pts',(-4.00047520099045,0.8496,1.1981954227983));
#21630=CARTESIAN_POINT('Ctrl Pts',(-4.00639322616607,0.,1.43558101932923));
#21631=CARTESIAN_POINT('Ctrl Pts',(-4.00639322616607,0.8496,1.43558101932923));
#21632=CARTESIAN_POINT('Ctrl Pts',(-4.01278239926574,0.,1.67142113207667));
#21633=CARTESIAN_POINT('Ctrl Pts',(-4.01278239926574,0.8496,1.67142113207667));
#21634=CARTESIAN_POINT('Ctrl Pts',(-4.02066709528487,0.,1.90332556813333));
#21635=CARTESIAN_POINT('Ctrl Pts',(-4.02066709528487,0.8496,1.90332556813333));
#21636=CARTESIAN_POINT('Ctrl Pts',(-4.0302101444685,0.,2.130657485557));
#21637=CARTESIAN_POINT('Ctrl Pts',(-4.0302101444685,0.8496,2.130657485557));
#21638=CARTESIAN_POINT('Ctrl Pts',(-4.04126813644779,0.,2.35385258470204));
#21639=CARTESIAN_POINT('Ctrl Pts',(-4.04126813644779,0.8496,2.35385258470204));
#21640=CARTESIAN_POINT('Ctrl Pts',(-4.05390260344525,0.,2.57377631141659));
#21641=CARTESIAN_POINT('Ctrl Pts',(-4.05390260344525,0.8496,2.57377631141659));
#21642=CARTESIAN_POINT('Ctrl Pts',(-4.06899962712502,0.,2.7909834104825));
#21643=CARTESIAN_POINT('Ctrl Pts',(-4.06899962712502,0.8496,2.7909834104825));
#21644=CARTESIAN_POINT('Ctrl Pts',(-4.08854433447739,0.,3.00529120729338));
#21645=CARTESIAN_POINT('Ctrl Pts',(-4.08854433447739,0.8496,3.00529120729338));
#21646=CARTESIAN_POINT('Ctrl Pts',(-4.11518318246524,0.,3.21600287470921));
#21647=CARTESIAN_POINT('Ctrl Pts',(-4.11518318246524,0.8496,3.21600287470921));
#21648=CARTESIAN_POINT('Ctrl Pts',(-4.15193466045748,0.,3.42199345348447));
#21649=CARTESIAN_POINT('Ctrl Pts',(-4.15193466045748,0.8496,3.42199345348447));
#21650=CARTESIAN_POINT('Ctrl Pts',(-4.20184334854115,0.,3.62185203209171));
#21651=CARTESIAN_POINT('Ctrl Pts',(-4.20184334854115,0.8496,3.62185203209171));
#21652=CARTESIAN_POINT('Ctrl Pts',(-4.26765207024395,0.,3.81399668859083));
#21653=CARTESIAN_POINT('Ctrl Pts',(-4.26765207024395,0.8496,3.81399668859083));
#21654=CARTESIAN_POINT('Ctrl Pts',(-4.35148411330718,0.,3.99681013615577));
#21655=CARTESIAN_POINT('Ctrl Pts',(-4.35148411330718,0.8496,3.99681013615577));
#21656=CARTESIAN_POINT('Ctrl Pts',(-4.45474519640294,0.,4.16885849319142));
#21657=CARTESIAN_POINT('Ctrl Pts',(-4.45474519640294,0.8496,4.16885849319142));
#21658=CARTESIAN_POINT('Ctrl Pts',(-4.57800047823775,0.,4.32911151507774));
#21659=CARTESIAN_POINT('Ctrl Pts',(-4.57800047823775,0.8496,4.32911151507774));
#21660=CARTESIAN_POINT('Ctrl Pts',(-4.7208720035032,0.,4.47714872481861));
#21661=CARTESIAN_POINT('Ctrl Pts',(-4.7208720035032,0.8496,4.47714872481861));
#21662=CARTESIAN_POINT('Ctrl Pts',(-4.88190185104852,0.,4.61340315498244));
#21663=CARTESIAN_POINT('Ctrl Pts',(-4.88190185104852,0.8496,4.61340315498244));
#21664=CARTESIAN_POINT('Ctrl Pts',(-5.05850630701885,0.,4.73929437247796));
#21665=CARTESIAN_POINT('Ctrl Pts',(-5.05850630701885,0.8496,4.73929437247796));
#21666=CARTESIAN_POINT('Ctrl Pts',(-5.24741086000019,0.,4.8567611153285));
#21667=CARTESIAN_POINT('Ctrl Pts',(-5.24741086000019,0.8496,4.8567611153285));
#21668=CARTESIAN_POINT('Ctrl Pts',(-5.44501860313342,0.,4.96787993373728));
#21669=CARTESIAN_POINT('Ctrl Pts',(-5.44501860313342,0.8496,4.96787993373728));
#21670=CARTESIAN_POINT('Ctrl Pts',(-5.64781737380319,0.,5.07442896098937));
#21671=CARTESIAN_POINT('Ctrl Pts',(-5.64781737380319,0.8496,5.07442896098937));
#21672=CARTESIAN_POINT('Ctrl Pts',(-5.85274048349242,0.,5.17752467829109));
#21673=CARTESIAN_POINT('Ctrl Pts',(-5.85274048349242,0.8496,5.17752467829109));
#21674=CARTESIAN_POINT('Ctrl Pts',(-6.05762450882858,0.,5.27709955371564));
#21675=CARTESIAN_POINT('Ctrl Pts',(-6.05762450882858,0.8496,5.27709955371564));
#21676=CARTESIAN_POINT('Ctrl Pts',(-6.26112587698772,0.,5.37226655127787));
#21677=CARTESIAN_POINT('Ctrl Pts',(-6.26112587698772,0.8496,5.37226655127787));
#21678=CARTESIAN_POINT('Ctrl Pts',(-6.46246210121964,0.,5.46195513100446));
#21679=CARTESIAN_POINT('Ctrl Pts',(-6.46246210121964,0.8496,5.46195513100446));
#21680=CARTESIAN_POINT('Ctrl Pts',(-6.66121503090592,0.,5.54547963906637));
#21681=CARTESIAN_POINT('Ctrl Pts',(-6.66121503090592,0.8496,5.54547963906637));
#21682=CARTESIAN_POINT('Ctrl Pts',(-6.8570997603751,0.,5.62308582598972));
#21683=CARTESIAN_POINT('Ctrl Pts',(-6.8570997603751,0.8496,5.62308582598972));
#21684=CARTESIAN_POINT('Ctrl Pts',(-7.04976847947249,0.,5.69662713609756));
#21685=CARTESIAN_POINT('Ctrl Pts',(-7.04976847947249,0.8496,5.69662713609756));
#21686=CARTESIAN_POINT('Ctrl Pts',(-7.23853768475,0.,5.76979878895672));
#21687=CARTESIAN_POINT('Ctrl Pts',(-7.23853768475,0.8496,5.76979878895672));
#21688=CARTESIAN_POINT('Ctrl Pts',(-7.42198551710617,0.,5.84723737025949));
#21689=CARTESIAN_POINT('Ctrl Pts',(-7.42198551710617,0.8496,5.84723737025949));
#21690=CARTESIAN_POINT('Ctrl Pts',(-7.59751903688412,0.,5.93381436957244));
#21691=CARTESIAN_POINT('Ctrl Pts',(-7.59751903688412,0.8496,5.93381436957244));
#21692=CARTESIAN_POINT('Ctrl Pts',(-7.76106756457753,0.,6.03389995867283));
#21693=CARTESIAN_POINT('Ctrl Pts',(-7.76106756457753,0.8496,6.03389995867283));
#21694=CARTESIAN_POINT('Ctrl Pts',(-7.90644860448901,0.,6.15052660592937));
#21695=CARTESIAN_POINT('Ctrl Pts',(-7.90644860448901,0.8496,6.15052660592937));
#21696=CARTESIAN_POINT('Ctrl Pts',(-8.02580908828117,0.,6.28498018271686));
#21697=CARTESIAN_POINT('Ctrl Pts',(-8.02580908828117,0.8496,6.28498018271686));
#21698=CARTESIAN_POINT('Ctrl Pts',(-8.11207116917861,0.,6.43720976255636));
#21699=CARTESIAN_POINT('Ctrl Pts',(-8.11207116917861,0.8496,6.43720976255636));
#21700=CARTESIAN_POINT('Ctrl Pts',(-8.16089752265956,0.,6.60605451948903));
#21701=CARTESIAN_POINT('Ctrl Pts',(-8.16089752265956,0.8496,6.60605451948903));
#21702=CARTESIAN_POINT('Ctrl Pts',(-8.17293082304181,0.,6.78954489191904));
#21703=CARTESIAN_POINT('Ctrl Pts',(-8.17293082304181,0.8496,6.78954489191904));
#21704=CARTESIAN_POINT('Ctrl Pts',(-8.15569042861244,0.,6.9851692342788));
#21705=CARTESIAN_POINT('Ctrl Pts',(-8.15569042861244,0.8496,6.9851692342788));
#21706=CARTESIAN_POINT('Ctrl Pts',(-8.12057943633387,0.,7.19009032473164));
#21707=CARTESIAN_POINT('Ctrl Pts',(-8.12057943633387,0.8496,7.19009032473164));
#21708=CARTESIAN_POINT('Ctrl Pts',(-8.08008348678073,0.,7.40136016279791));
#21709=CARTESIAN_POINT('Ctrl Pts',(-8.08008348678073,0.8496,7.40136016279791));
#21710=CARTESIAN_POINT('Ctrl Pts',(-8.04494633492831,0.,7.61613341658677));
#21711=CARTESIAN_POINT('Ctrl Pts',(-8.04494633492831,0.8496,7.61613341658677));
#21712=CARTESIAN_POINT('Ctrl Pts',(-8.02124364536279,0.,7.83188673232793));
#21713=CARTESIAN_POINT('Ctrl Pts',(-8.02124364536279,0.8496,7.83188673232793));
#21714=CARTESIAN_POINT('Ctrl Pts',(-8.007818938056,0.,8.04662057355248));
#21715=CARTESIAN_POINT('Ctrl Pts',(-8.007818938056,0.8496,8.04662057355248));
#21716=CARTESIAN_POINT('Ctrl Pts',(-7.99879843919661,0.,8.25883677791483));
#21717=CARTESIAN_POINT('Ctrl Pts',(-7.99879843919661,0.8496,8.25883677791483));
#21718=CARTESIAN_POINT('Ctrl Pts',(-7.98575825096101,0.,8.46752658699528));
#21719=CARTESIAN_POINT('Ctrl Pts',(-7.98575825096101,0.8496,8.46752658699528));
#21720=CARTESIAN_POINT('Ctrl Pts',(-7.96007609558389,0.,8.67216210283896));
#21721=CARTESIAN_POINT('Ctrl Pts',(-7.96007609558389,0.8496,8.67216210283896));
#21722=CARTESIAN_POINT('Ctrl Pts',(-7.91508259073019,0.,8.87266947141823));
#21723=CARTESIAN_POINT('Ctrl Pts',(-7.91508259073019,0.8496,8.87266947141823));
#21724=CARTESIAN_POINT('Ctrl Pts',(-7.84862074946261,0.,9.06945407016992));
#21725=CARTESIAN_POINT('Ctrl Pts',(-7.84862074946261,0.8496,9.06945407016992));
#21726=CARTESIAN_POINT('Ctrl Pts',(-7.76209282457479,0.,9.26297089919765));
#21727=CARTESIAN_POINT('Ctrl Pts',(-7.76209282457479,0.8496,9.26297089919765));
#21728=CARTESIAN_POINT('Ctrl Pts',(-7.65900038660722,0.,9.4532499945042));
#21729=CARTESIAN_POINT('Ctrl Pts',(-7.65900038660722,0.8496,9.4532499945042));
#21730=CARTESIAN_POINT('Ctrl Pts',(-7.5436057352653,0.,9.63939026966035));
#21731=CARTESIAN_POINT('Ctrl Pts',(-7.5436057352653,0.8496,9.63939026966035));
#21732=CARTESIAN_POINT('Ctrl Pts',(-7.41967047355001,0.,9.81917361987397));
#21733=CARTESIAN_POINT('Ctrl Pts',(-7.41967047355001,0.8496,9.81917361987397));
#21734=CARTESIAN_POINT('Ctrl Pts',(-7.28883796912703,0.,9.98835756998572));
#21735=CARTESIAN_POINT('Ctrl Pts',(-7.28883796912703,0.8496,9.98835756998572));
#21736=CARTESIAN_POINT('Ctrl Pts',(-7.15081550722306,0.,10.1414720974148));
#21737=CARTESIAN_POINT('Ctrl Pts',(-7.15081550722306,0.8496,10.1414720974148));
#21738=CARTESIAN_POINT('Ctrl Pts',(-7.0044544864105,0.,10.2733319413008));
#21739=CARTESIAN_POINT('Ctrl Pts',(-7.0044544864105,0.8496,10.2733319413008));
#21740=CARTESIAN_POINT('Ctrl Pts',(-6.84859008776113,0.,10.3804015453596));
#21741=CARTESIAN_POINT('Ctrl Pts',(-6.84859008776113,0.8496,10.3804015453596));
#21742=CARTESIAN_POINT('Ctrl Pts',(-6.68288828293938,0.,10.4620502678778));
#21743=CARTESIAN_POINT('Ctrl Pts',(-6.68288828293938,0.8496,10.4620502678778));
#21744=CARTESIAN_POINT('Ctrl Pts',(-6.50892555577766,0.,10.522290883026));
#21745=CARTESIAN_POINT('Ctrl Pts',(-6.50892555577766,0.8496,10.522290883026));
#21746=CARTESIAN_POINT('Ctrl Pts',(-6.32976796473811,0.,10.5687216653902));
#21747=CARTESIAN_POINT('Ctrl Pts',(-6.32976796473811,0.8496,10.5687216653902));
#21748=CARTESIAN_POINT('Ctrl Pts',(-6.14893768388701,0.,10.6103475969885));
#21749=CARTESIAN_POINT('Ctrl Pts',(-6.14893768388701,0.8496,10.6103475969885));
#21750=CARTESIAN_POINT('Ctrl Pts',(-5.96961932707142,0.,10.6558377434043));
#21751=CARTESIAN_POINT('Ctrl Pts',(-5.96961932707142,0.8496,10.6558377434043));
#21752=CARTESIAN_POINT('Ctrl Pts',(-5.79367695415031,0.,10.7114411549114));
#21753=CARTESIAN_POINT('Ctrl Pts',(-5.79367695415031,0.8496,10.7114411549114));
#21754=CARTESIAN_POINT('Ctrl Pts',(-5.62101499943431,0.,10.7795199127535));
#21755=CARTESIAN_POINT('Ctrl Pts',(-5.62101499943431,0.8496,10.7795199127535));
#21756=CARTESIAN_POINT('Ctrl Pts',(-5.45051506148982,0.,10.8599381259737));
#21757=CARTESIAN_POINT('Ctrl Pts',(-5.45051506148982,0.8496,10.8599381259737));
#21758=CARTESIAN_POINT('Ctrl Pts',(-5.28082876351929,0.,10.9511663773826));
#21759=CARTESIAN_POINT('Ctrl Pts',(-5.28082876351929,0.8496,10.9511663773826));
#21760=CARTESIAN_POINT('Ctrl Pts',(-5.11112998264616,0.,11.0513704191329));
#21761=CARTESIAN_POINT('Ctrl Pts',(-5.11112998264616,0.8496,11.0513704191329));
#21762=CARTESIAN_POINT('Ctrl Pts',(-4.94211773226973,0.,11.1598106424589));
#21763=CARTESIAN_POINT('Ctrl Pts',(-4.94211773226973,0.8496,11.1598106424589));
#21764=CARTESIAN_POINT('Ctrl Pts',(-4.77596612414951,0.,11.2768795166235));
#21765=CARTESIAN_POINT('Ctrl Pts',(-4.77596612414951,0.8496,11.2768795166235));
#21766=CARTESIAN_POINT('Ctrl Pts',(-4.61532593596946,0.,11.4029224160731));
#21767=CARTESIAN_POINT('Ctrl Pts',(-4.61532593596946,0.8496,11.4029224160731));
#21768=CARTESIAN_POINT('Ctrl Pts',(-4.46255574628757,0.,11.5373242211527));
#21769=CARTESIAN_POINT('Ctrl Pts',(-4.46255574628757,0.8496,11.5373242211527));
#21770=CARTESIAN_POINT('Ctrl Pts',(-4.31893584999241,0.,11.6776492463597));
#21771=CARTESIAN_POINT('Ctrl Pts',(-4.31893584999241,0.8496,11.6776492463597));
#21772=CARTESIAN_POINT('Ctrl Pts',(-4.18369962429796,0.,11.8183570873721));
#21773=CARTESIAN_POINT('Ctrl Pts',(-4.18369962429796,0.8496,11.8183570873721));
#21774=CARTESIAN_POINT('Ctrl Pts',(-4.05395481372655,0.,11.9514202619522));
#21775=CARTESIAN_POINT('Ctrl Pts',(-4.05395481372655,0.8496,11.9514202619522));
#21776=CARTESIAN_POINT('Ctrl Pts',(-3.92533033057354,0.,12.0684942936867));
#21777=CARTESIAN_POINT('Ctrl Pts',(-3.92533033057354,0.8496,12.0684942936867));
#21778=CARTESIAN_POINT('Ctrl Pts',(-3.79241297762166,0.,12.1626050652586));
#21779=CARTESIAN_POINT('Ctrl Pts',(-3.79241297762166,0.8496,12.1626050652586));
#21780=CARTESIAN_POINT('Ctrl Pts',(-3.64927048315908,0.,12.2301117722809));
#21781=CARTESIAN_POINT('Ctrl Pts',(-3.64927048315908,0.8496,12.2301117722809));
#21782=CARTESIAN_POINT('Ctrl Pts',(-3.48993681214334,0.,12.2723364229645));
#21783=CARTESIAN_POINT('Ctrl Pts',(-3.48993681214334,0.8496,12.2723364229645));
#21784=CARTESIAN_POINT('Ctrl Pts',(-3.30884480305534,0.,12.2938762651139));
#21785=CARTESIAN_POINT('Ctrl Pts',(-3.30884480305534,0.8496,12.2938762651139));
#21786=CARTESIAN_POINT('Ctrl Pts',(-3.10127560868576,0.,12.3010487961981));
#21787=CARTESIAN_POINT('Ctrl Pts',(-3.10127560868576,0.8496,12.3010487961981));
#21788=CARTESIAN_POINT('Ctrl Pts',(-2.86376302967345,0.,12.300400839059));
#21789=CARTESIAN_POINT('Ctrl Pts',(-2.86376302967345,0.8496,12.300400839059));
#21790=CARTESIAN_POINT('Ctrl Pts',(-2.59461297443094,0.,12.2969132923574));
#21791=CARTESIAN_POINT('Ctrl Pts',(-2.59461297443094,0.8496,12.2969132923574));
#21792=CARTESIAN_POINT('Ctrl Pts',(-2.29394197380209,0.,12.2935845551224));
#21793=CARTESIAN_POINT('Ctrl Pts',(-2.29394197380209,0.8496,12.2935845551224));
#21794=CARTESIAN_POINT('Ctrl Pts',(-1.96338745719135,0.,12.2919684497906));
#21795=CARTESIAN_POINT('Ctrl Pts',(-1.96338745719135,0.8496,12.2919684497906));
#21796=CARTESIAN_POINT('Ctrl Pts',(-1.60591558979456,0.,12.2924280531798));
#21797=CARTESIAN_POINT('Ctrl Pts',(-1.60591558979456,0.8496,12.2924280531798));
#21798=CARTESIAN_POINT('Ctrl Pts',(-1.22558901314075,0.,12.2945066442122));
#21799=CARTESIAN_POINT('Ctrl Pts',(-1.22558901314075,0.8496,12.2945066442122));
#21800=CARTESIAN_POINT('Ctrl Pts',(-0.827351903312651,0.,12.2972483292773));
#21801=CARTESIAN_POINT('Ctrl Pts',(-0.827351903312651,0.8496,12.2972483292773));
#21802=CARTESIAN_POINT('Ctrl Pts',(-0.498916532526571,0.,12.299081889758));
#21803=CARTESIAN_POINT('Ctrl Pts',(-0.498916532526571,0.8496,12.299081889758));
#21804=CARTESIAN_POINT('Ctrl Pts',(-0.249771440080693,0.,12.2998330708668));
#21805=CARTESIAN_POINT('Ctrl Pts',(-0.249771440080693,0.8496,12.2998330708668));
#21806=CARTESIAN_POINT('Ctrl Pts',(-0.0832571466935557,0.,12.2999999999989));
#21807=CARTESIAN_POINT('Ctrl Pts',(-0.0832571466935557,0.8496,12.2999999999989));
#21808=CARTESIAN_POINT('Ctrl Pts',(0.,0.,12.3));
#21809=CARTESIAN_POINT('Ctrl Pts',(0.,0.8496,12.3));
#21810=CARTESIAN_POINT('Ctrl Pts',(0.0832571466935396,0.,12.3000000000011));
#21811=CARTESIAN_POINT('Ctrl Pts',(0.0832571466935396,0.8496,12.3000000000011));
#21812=CARTESIAN_POINT('Ctrl Pts',(0.24977144008061,0.,12.2998330708736));
#21813=CARTESIAN_POINT('Ctrl Pts',(0.24977144008061,0.8496,12.2998330708736));
#21814=CARTESIAN_POINT('Ctrl Pts',(0.498916532526534,0.,12.2990818897713));
#21815=CARTESIAN_POINT('Ctrl Pts',(0.498916532526534,0.8496,12.2990818897713));
#21816=CARTESIAN_POINT('Ctrl Pts',(0.827351903312438,0.,12.2972483292974));
#21817=CARTESIAN_POINT('Ctrl Pts',(0.827351903312438,0.8496,12.2972483292974));
#21818=CARTESIAN_POINT('Ctrl Pts',(1.22558901314046,0.,12.2945066442369));
#21819=CARTESIAN_POINT('Ctrl Pts',(1.22558901314046,0.8496,12.2945066442369));
#21820=CARTESIAN_POINT('Ctrl Pts',(1.60591558979418,0.,12.2924280532047));
#21821=CARTESIAN_POINT('Ctrl Pts',(1.60591558979418,0.8496,12.2924280532047));
#21822=CARTESIAN_POINT('Ctrl Pts',(1.96338745719096,0.,12.291968449812));
#21823=CARTESIAN_POINT('Ctrl Pts',(1.96338745719096,0.8496,12.291968449812));
#21824=CARTESIAN_POINT('Ctrl Pts',(2.29394197380175,0.,12.2935845551378));
#21825=CARTESIAN_POINT('Ctrl Pts',(2.29394197380175,0.8496,12.2935845551378));
#21826=CARTESIAN_POINT('Ctrl Pts',(2.59461297443069,0.,12.2969132923658));
#21827=CARTESIAN_POINT('Ctrl Pts',(2.59461297443069,0.8496,12.2969132923658));
#21828=CARTESIAN_POINT('Ctrl Pts',(2.86376302967335,0.,12.3004008390612));
#21829=CARTESIAN_POINT('Ctrl Pts',(2.86376302967335,0.8496,12.3004008390612));
#21830=CARTESIAN_POINT('Ctrl Pts',(3.10127560868576,0.,12.3010487961961));
#21831=CARTESIAN_POINT('Ctrl Pts',(3.10127560868576,0.8496,12.3010487961961));
#21832=CARTESIAN_POINT('Ctrl Pts',(3.30884480305537,0.,12.2938762651102));
#21833=CARTESIAN_POINT('Ctrl Pts',(3.30884480305537,0.8496,12.2938762651102));
#21834=CARTESIAN_POINT('Ctrl Pts',(3.48993681214337,0.,12.2723364229612));
#21835=CARTESIAN_POINT('Ctrl Pts',(3.48993681214337,0.8496,12.2723364229612));
#21836=CARTESIAN_POINT('Ctrl Pts',(3.64927048315907,0.,12.2301117722792));
#21837=CARTESIAN_POINT('Ctrl Pts',(3.64927048315907,0.8496,12.2301117722792));
#21838=CARTESIAN_POINT('Ctrl Pts',(3.79241297762162,0.,12.1626050652587));
#21839=CARTESIAN_POINT('Ctrl Pts',(3.79241297762162,0.8496,12.1626050652587));
#21840=CARTESIAN_POINT('Ctrl Pts',(3.90811725944041,0.,12.0806818325566));
#21841=CARTESIAN_POINT('Ctrl Pts',(3.90811725944041,0.8496,12.0806818325566));
#21842=CARTESIAN_POINT('Ctrl Pts',(3.99482565231282,0.,12.0046763352305));
#21843=CARTESIAN_POINT('Ctrl Pts',(3.99482565231282,0.8496,12.0046763352305));
#21844=CARTESIAN_POINT('Ctrl Pts',(4.05565687163389,0.,11.9465013108381));
#21845=CARTESIAN_POINT('Ctrl Pts',(4.05565687163389,0.8496,11.9465013108381));
#21846=CARTESIAN_POINT('Ctrl Pts',(4.0908196144603,0.,11.9117811315282));
#21847=CARTESIAN_POINT('Ctrl Pts',(4.0908196144603,0.8496,11.9117811315282));
#21848=CARTESIAN_POINT('Ctrl Pts',(4.1,0.,11.9026515720695));
#21849=CARTESIAN_POINT('Ctrl Pts',(4.1,0.8496,11.9026515720695));
#21850=CARTESIAN_POINT('',(4.10063757647074,0.292307308198873,3.09202603079313));
#21851=CARTESIAN_POINT('',(4.1006262898548,0.292339670981987,3.09201395474132));
#21852=CARTESIAN_POINT('Ctrl Pts',(4.15877746029711,0.0799982138568305,
3.43674861413894));
#21853=CARTESIAN_POINT('Ctrl Pts',(4.14646117554196,0.124733851720112,3.38095797208512));
#21854=CARTESIAN_POINT('Ctrl Pts',(4.12508521221268,0.202624969870674,3.27000814202033));
#21855=CARTESIAN_POINT('Ctrl Pts',(4.10791209946146,0.265571898245336,3.14988703412665));
#21856=CARTESIAN_POINT('Ctrl Pts',(4.1006381376306,0.292296403815986,3.09203050838626));
#21857=CARTESIAN_POINT('Origin',(4.18004567262241,0.307776805703052,3.08202038908219));
#21858=CARTESIAN_POINT('Origin',(4.36136464669403,0.283715212921747,3.04584783530248));
#21859=CARTESIAN_POINT('Origin',(4.1,0.,1.2));
#21860=CARTESIAN_POINT('Ctrl Pts',(4.29339835604888,0.0559939529287135,
3.55467920026169));
#21861=CARTESIAN_POINT('Ctrl Pts',(4.25584474784527,0.150162334098852,3.46593762044134));
#21862=CARTESIAN_POINT('Ctrl Pts',(4.17638455329654,0.33726205850833,3.22405277301241));
#21863=CARTESIAN_POINT('Ctrl Pts',(4.13042338687859,0.443584832494149,2.92533348324746));
#21864=CARTESIAN_POINT('Ctrl Pts',(4.11051138672739,0.490305829863764,2.74803482597387));
#21865=CARTESIAN_POINT('Ctrl Pts',(4.3060475661543,0.0550570568185274,3.54597738315241));
#21866=CARTESIAN_POINT('Ctrl Pts',(4.26914663034547,0.150354528702341,3.45998535295299));
#21867=CARTESIAN_POINT('Ctrl Pts',(4.18859964481653,0.340124295101877,3.22265812391974));
#21868=CARTESIAN_POINT('Ctrl Pts',(4.14050849741124,0.447815386226925,2.92485200908127));
#21869=CARTESIAN_POINT('Ctrl Pts',(4.11965690824515,0.495007873940908,2.74784464353325));
#21870=CARTESIAN_POINT('Ctrl Pts',(4.33523822515995,0.0596089270271733,
3.53376471245904));
#21871=CARTESIAN_POINT('Ctrl Pts',(4.29744618195624,0.156949697666454,3.45282690279432));
#21872=CARTESIAN_POINT('Ctrl Pts',(4.21178168150148,0.35100840785864,3.22251980707619));
#21873=CARTESIAN_POINT('Ctrl Pts',(4.15902952625075,0.460249382405453,2.92536481676328));
#21874=CARTESIAN_POINT('Ctrl Pts',(4.13617464437627,0.507855044332698,2.74857164914344));
#21875=CARTESIAN_POINT('Ctrl Pts',(4.38400568703593,0.0874022066366798,
3.53702215045297));
#21876=CARTESIAN_POINT('Ctrl Pts',(4.3397963041374,0.186814587951356,3.45970264916118));
#21877=CARTESIAN_POINT('Ctrl Pts',(4.24053830160474,0.383996027912259,3.23126786608819));
#21878=CARTESIAN_POINT('Ctrl Pts',(4.18058055549715,0.492294479045333,2.93123150415905));
#21879=CARTESIAN_POINT('Ctrl Pts',(4.15478642497044,0.539079251837051,2.75350788240694));
#21880=CARTESIAN_POINT('Ctrl Pts',(4.40199170668536,0.116954263196119,3.56084440742005));
#21881=CARTESIAN_POINT('Ctrl Pts',(4.35269219239138,0.217003436097948,3.48044613277936));
#21882=CARTESIAN_POINT('Ctrl Pts',(4.24528014220526,0.413945938159646,3.24416115246424));
#21883=CARTESIAN_POINT('Ctrl Pts',(4.18297157398144,0.519676492843704,2.93904329627266));
#21884=CARTESIAN_POINT('Ctrl Pts',(4.15627962724123,0.565091367558406,2.75968239072319));
#21885=CARTESIAN_POINT('Ctrl Pts',(4.4028813462376,0.132178376897717,3.57815186105023));
#21886=CARTESIAN_POINT('Ctrl Pts',(4.35199587562355,0.232956026703696,3.49496809556833));
#21887=CARTESIAN_POINT('Ctrl Pts',(4.24197300931968,0.430310911915843,3.25270142258189));
#21888=CARTESIAN_POINT('Ctrl Pts',(4.17940016830811,0.534808403083364,2.94423234285935));
#21889=CARTESIAN_POINT('Ctrl Pts',(4.15273910526043,0.579540791776975,2.76375542954464));
#21890=CARTESIAN_POINT('',(4.11092960039253,0.489270313943276,2.7535990262568));
#21891=CARTESIAN_POINT('Ctrl Pts',(4.29338839752952,0.0560337429176049,
3.55463113046212));
#21892=CARTESIAN_POINT('Ctrl Pts',(4.28200201425128,0.0845703603400842,
3.52772622977568));
#21893=CARTESIAN_POINT('Ctrl Pts',(4.2709089389845,0.111840202565025,3.49944329913683));
#21894=CARTESIAN_POINT('Ctrl Pts',(4.26022466516199,0.137812970890808,3.46992665998807));
#21895=CARTESIAN_POINT('Ctrl Pts',(4.24925651305979,0.164475828680185,3.43962577168181));
#21896=CARTESIAN_POINT('Ctrl Pts',(4.23871834098693,0.189772252648034,3.40802535345698));
#21897=CARTESIAN_POINT('Ctrl Pts',(4.22869342338732,0.213651455574615,3.37524966812642));
#21898=CARTESIAN_POINT('Ctrl Pts',(4.22022011266837,0.233834754250891,3.34754684034024));
#21899=CARTESIAN_POINT('Ctrl Pts',(4.21211246977426,0.253005453813316,3.31900381508105));
#21900=CARTESIAN_POINT('Ctrl Pts',(4.20440515624013,0.271118966485284,3.28967551860074));
#21901=CARTESIAN_POINT('Ctrl Pts',(4.20081384008402,0.279559177255812,3.27600964338828));
#21902=CARTESIAN_POINT('Ctrl Pts',(4.19730929252788,0.287769629485392,3.26217300268237));
#21903=CARTESIAN_POINT('Ctrl Pts',(4.19388960090582,0.295760962667081,3.24817707975791));
#21904=CARTESIAN_POINT('Ctrl Pts',(4.1836826106382,0.319613247909556,3.2064024799213));
#21905=CARTESIAN_POINT('Ctrl Pts',(4.17426127019943,0.341554919196119,3.16314473495888));
#21906=CARTESIAN_POINT('Ctrl Pts',(4.16557077913211,0.36180048426393,3.11876022001722));
#21907=CARTESIAN_POINT('Ctrl Pts',(4.15562425095267,0.384972141871765,3.06796080889318));
#21908=CARTESIAN_POINT('Ctrl Pts',(4.14663412018599,0.405922678178319,3.01568449521542));
#21909=CARTESIAN_POINT('Ctrl Pts',(4.13847959221096,0.424941648061345,2.96242067986732));
#21910=CARTESIAN_POINT('Ctrl Pts',(4.13793497928194,0.426211859767844,2.95886337249452));
#21911=CARTESIAN_POINT('Ctrl Pts',(4.13739408426757,0.427473443573063,2.9553016503188));
#21912=CARTESIAN_POINT('Ctrl Pts',(4.13685686763256,0.428726480598055,2.95173565560756));
#21913=CARTESIAN_POINT('Ctrl Pts',(4.12711395055437,0.451451457888153,2.88706306635978));
#21914=CARTESIAN_POINT('Ctrl Pts',(4.1185832632104,0.471366282144737,2.82098952702215));
#21915=CARTESIAN_POINT('Ctrl Pts',(4.11092961016103,0.48927029109206,2.75359911226844));
#21916=CARTESIAN_POINT('Ctrl Pts',(4.11092959062404,0.489270336794493,2.75359894024517));
#21917=CARTESIAN_POINT('Ctrl Pts',(4.1107363463406,0.48972238856588,2.75189742393957));
#21918=CARTESIAN_POINT('Ctrl Pts',(4.11054370257317,0.490173111237358,2.75019527901328));
#21919=CARTESIAN_POINT('Ctrl Pts',(4.11035165498701,0.490622516758464,2.74849251651165));
#21920=CARTESIAN_POINT('Ctrl Pts',(4.29852898837605,0.0372770987405308,
3.57383899454876));
#21921=CARTESIAN_POINT('Ctrl Pts',(4.27477346003042,0.123982026893121,3.48643046936511));
#21922=CARTESIAN_POINT('Ctrl Pts',(4.23193632460675,0.280581959460234,3.29066087065414));
#21923=CARTESIAN_POINT('Ctrl Pts',(4.1817587479489,0.465308268502128,2.89185740177477));
#21924=CARTESIAN_POINT('Ctrl Pts',(4.16266015813344,0.536354908261444,2.59271405704707));
#21925=CARTESIAN_POINT('Ctrl Pts',(4.15265762140395,0.573560196368465,2.41375802693634));
#21926=CARTESIAN_POINT('Ctrl Pts',(4.27990542769405,0.0415912017479113,
3.58302567652478));
#21927=CARTESIAN_POINT('Ctrl Pts',(4.25574518298946,0.128851626852539,3.49496679687017));
#21928=CARTESIAN_POINT('Ctrl Pts',(4.21217417030772,0.286596632409413,3.29758018724282));
#21929=CARTESIAN_POINT('Ctrl Pts',(4.16134218460521,0.472536053380556,2.89573250617543));
#21930=CARTESIAN_POINT('Ctrl Pts',(4.14218738993462,0.543679227290343,2.59573641962871));
#21931=CARTESIAN_POINT('Ctrl Pts',(4.13215107098433,0.580950336455741,2.4164357799317));
#21932=CARTESIAN_POINT('Ctrl Pts',(4.2425246107023,0.0384093103467611,3.58977350532038));
#21933=CARTESIAN_POINT('Ctrl Pts',(4.21784750090365,0.125768723447587,3.50101955140993));
#21934=CARTESIAN_POINT('Ctrl Pts',(4.17340163251863,0.283772364998772,3.30214121155968));
#21935=CARTESIAN_POINT('Ctrl Pts',(4.12188632167338,0.469965279517223,2.89820958314819));
#21936=CARTESIAN_POINT('Ctrl Pts',(4.10266098140499,0.541170438724443,2.59763356171415));
#21937=CARTESIAN_POINT('Ctrl Pts',(4.09259095256892,0.578455090364732,2.41812014531828));
#21938=CARTESIAN_POINT('Ctrl Pts',(4.20079672067991,0.0123622460192512,
3.57509535012891));
#21939=CARTESIAN_POINT('Ctrl Pts',(4.17648320323078,0.0980364595359651,
3.48663488226387));
#21940=CARTESIAN_POINT('Ctrl Pts',(4.1329090360641,0.2524767319253,3.28946784706272));
#21941=CARTESIAN_POINT('Ctrl Pts',(4.08235693904747,0.435012022130954,2.8906393693344));
#21942=CARTESIAN_POINT('Ctrl Pts',(4.06323935395148,0.50581699413431,2.59179524992414));
#21943=CARTESIAN_POINT('Ctrl Pts',(4.0532219348772,0.542904670388583,2.41292428466811));
#21944=CARTESIAN_POINT('Ctrl Pts',(4.18838200131568,-0.00802902932684357,
3.55824631789071));
#21945=CARTESIAN_POINT('Ctrl Pts',(4.16482172696645,0.0761931109747066,
3.47052062622828));
#21946=CARTESIAN_POINT('Ctrl Pts',(4.12272687827244,0.227572559537098,3.2758060231306));
#21947=CARTESIAN_POINT('Ctrl Pts',(4.07356897734373,0.406942533188969,2.88269695569247));
#21948=CARTESIAN_POINT('Ctrl Pts',(4.05459109477352,0.477418672060344,2.58565061480296));
#21949=CARTESIAN_POINT('Ctrl Pts',(4.04464671888026,0.514335567712338,2.40746452010013));
#21950=CARTESIAN_POINT('Ctrl Pts',(4.1858850014514,-0.0182571874063626,
3.54880807404773));
#21951=CARTESIAN_POINT('Ctrl Pts',(4.16280303442141,0.0652367320815442,
3.46156265250184));
#21952=CARTESIAN_POINT('Ctrl Pts',(4.12161403444145,0.215078388014765,3.26830977903833));
#21953=CARTESIAN_POINT('Ctrl Pts',(4.07328088856278,0.392860332120455,2.87837605543618));
#21954=CARTESIAN_POINT('Ctrl Pts',(4.05438293677277,0.463168756286503,2.58230694074878));
#21955=CARTESIAN_POINT('Ctrl Pts',(4.04448133058357,0.5000000000037,2.4044944869251));
#21956=CARTESIAN_POINT('Ctrl Pts',(4.13468980447943,0.501507067233083,11.7463816858832));
#21957=CARTESIAN_POINT('Ctrl Pts',(4.12315670636567,0.500503082254402,11.7605952205767));
#21958=CARTESIAN_POINT('Ctrl Pts',(4.11159548058617,0.5,11.7748268489774));
#21959=CARTESIAN_POINT('Ctrl Pts',(4.1,0.5,11.7890187209237));
#21960=CARTESIAN_POINT('Ctrl Pts',(4.15241805382695,0.503050355590439,11.7637744947979));
#21961=CARTESIAN_POINT('Ctrl Pts',(4.14072380658156,0.501498211900196,11.7777465183035));
#21962=CARTESIAN_POINT('Ctrl Pts',(4.1289422172797,0.500510602421279,11.7917766549303));
#21963=CARTESIAN_POINT('Ctrl Pts',(4.11709141945523,0.5,11.8057761908248));
#21964=CARTESIAN_POINT('Ctrl Pts',(4.18493513822404,0.483966152642229,11.7938187431267));
#21965=CARTESIAN_POINT('Ctrl Pts',(4.17228908000075,0.482051425256797,11.80741030448));
#21966=CARTESIAN_POINT('Ctrl Pts',(4.15953538207889,0.480683792904307,11.8210795723414));
#21967=CARTESIAN_POINT('Ctrl Pts',(4.14667030106967,0.479896459182794,11.8347771301359));
#21968=CARTESIAN_POINT('Ctrl Pts',(4.19815579876099,0.440436692354107,11.8030020113162));
#21969=CARTESIAN_POINT('Ctrl Pts',(4.1845616929059,0.439020641370625,11.8169554560875));
#21970=CARTESIAN_POINT('Ctrl Pts',(4.17089559391198,0.438186472135287,11.830986356775));
#21971=CARTESIAN_POINT('Ctrl Pts',(4.15712386170588,0.437951958020513,11.8450264384616));
#21972=CARTESIAN_POINT('Ctrl Pts',(4.19894501008271,0.421808480679699,11.8021914830442));
#21973=CARTESIAN_POINT('Ctrl Pts',(4.18508246714534,0.420603698705282,11.8164284594574));
#21974=CARTESIAN_POINT('Ctrl Pts',(4.17114700318572,0.42,11.8307238382166));
#21975=CARTESIAN_POINT('Ctrl Pts',(4.15712386170588,0.42,11.8450264384616));
#21976=CARTESIAN_POINT('Origin',(4.03743041112843,1.49645215763755,11.737916375275));
#21977=CARTESIAN_POINT('',(4.15712386170589,0.42,11.8450264384616));
#21978=CARTESIAN_POINT('Origin',(4.1,0.42,11.7890187209237));
#21979=CARTESIAN_POINT('Ctrl Pts',(4.15712386170588,0.42,11.8450264384616));
#21980=CARTESIAN_POINT('Ctrl Pts',(4.17114700318572,0.42,11.8307238382166));
#21981=CARTESIAN_POINT('Ctrl Pts',(4.18508246714534,0.420603698705282,11.8164284594574));
#21982=CARTESIAN_POINT('Ctrl Pts',(4.19894501008271,0.421808480679699,11.8021914830442));
#21983=CARTESIAN_POINT('Ctrl Pts',(4.09999999999981,0.42,11.9026515720696));
#21984=CARTESIAN_POINT('Ctrl Pts',(4.11927627294066,0.42,11.8834820198546));
#21985=CARTESIAN_POINT('Ctrl Pts',(4.13827843210563,0.42,11.8642474273109));
#21986=CARTESIAN_POINT('Ctrl Pts',(4.15712386170585,0.42,11.8450264384616));
#21987=CARTESIAN_POINT('Ctrl Pts',(4.09999999999981,0.443935944027351,11.9026515720696));
#21988=CARTESIAN_POINT('Ctrl Pts',(4.11927735039401,0.44393594402735,11.8834809483665));
#21989=CARTESIAN_POINT('Ctrl Pts',(4.13827796583818,0.44393594402735,11.8642479028703));
#21990=CARTESIAN_POINT('Ctrl Pts',(4.15712386170585,0.44393594402735,11.8450264384616));
#21991=CARTESIAN_POINT('Ctrl Pts',(4.08582416465968,0.485360148657719,11.8883968170229));
#21992=CARTESIAN_POINT('Ctrl Pts',(4.10501545837473,0.485360148657719,11.8693117735566));
#21993=CARTESIAN_POINT('Ctrl Pts',(4.12396030833632,0.485360148657719,11.8501355018591));
#21994=CARTESIAN_POINT('Ctrl Pts',(4.14276896321521,0.485360148657719,11.8309520205925));
#21995=CARTESIAN_POINT('Ctrl Pts',(4.05624736761447,0.5,11.8586553600413));
#21996=CARTESIAN_POINT('Ctrl Pts',(4.07526199817245,0.5,11.8397460016581));
#21997=CARTESIAN_POINT('Ctrl Pts',(4.0940863606134,0.499999999999999,11.8206923301711));
#21998=CARTESIAN_POINT('Ctrl Pts',(4.11281856459138,0.499999999999999,11.8015868233495));
#21999=CARTESIAN_POINT('Ctrl Pts',(4.0435887019288,0.500000000000001,11.8459262210355));
#22000=CARTESIAN_POINT('Ctrl Pts',(4.06252783272241,0.5,11.8270919444215));
#22001=CARTESIAN_POINT('Ctrl Pts',(4.08130046851069,0.499999999999999,11.8080909041462));
#22002=CARTESIAN_POINT('Ctrl Pts',(4.09999999999996,0.499999999999999,11.7890187209237));
#22003=CARTESIAN_POINT('Ctrl Pts',(4.09999999999981,0.42,11.9026515720696));
#22004=CARTESIAN_POINT('Ctrl Pts',(4.11927627294066,0.42,11.8834820198546));
#22005=CARTESIAN_POINT('Ctrl Pts',(4.13827843210563,0.42,11.8642474273109));
#22006=CARTESIAN_POINT('Ctrl Pts',(4.15712386170585,0.42,11.8450264384616));
#22007=CARTESIAN_POINT('Origin',(-4.1,0.9,6.5));
#22008=CARTESIAN_POINT('Origin',(4.1,0.9,6.5));
#22009=CARTESIAN_POINT('Ctrl Pts',(-4.1,-1.17961196366423E-16,1.26933116532693));
#22010=CARTESIAN_POINT('Ctrl Pts',(-4.1,0.6,1.26933116532693));
#22011=CARTESIAN_POINT('Ctrl Pts',(-4.1,-1.17961196366423E-16,1.25328382445493));
#22012=CARTESIAN_POINT('Ctrl Pts',(-4.1,0.6,1.25328382445493));
#22013=CARTESIAN_POINT('Ctrl Pts',(-4.09002305366,-1.18393877442287E-16,
1.22124310128144));
#22014=CARTESIAN_POINT('Ctrl Pts',(-4.09002305366,0.6,1.22124310128144));
#22015=CARTESIAN_POINT('Ctrl Pts',(-4.06370099763855,-1.19535414655197E-16,
1.2004273196109));
#22016=CARTESIAN_POINT('Ctrl Pts',(-4.06370099763855,0.6,1.2004273196109));
#22017=CARTESIAN_POINT('Ctrl Pts',(-4.04872369693346,-1.20184951533693E-16,
1.19466558266346));
#22018=CARTESIAN_POINT('Ctrl Pts',(-4.04872369693346,0.6,1.19466558266346));
#22019=CARTESIAN_POINT('',(-4.05991477685645,0.499739255703113,1.19999999917294));
#22020=CARTESIAN_POINT('',(-4.04872369689169,0.425808996579714,1.19466558264739));
#22021=CARTESIAN_POINT('Ctrl Pts',(-4.05991477685645,0.499739255703113,
1.19999999917294));
#22022=CARTESIAN_POINT('Ctrl Pts',(-4.05991218030895,0.474962555580598,
1.19999833336884));
#22023=CARTESIAN_POINT('Ctrl Pts',(-4.05598720035336,0.449889989994391,
1.19748057630533));
#22024=CARTESIAN_POINT('Ctrl Pts',(-4.04884919779574,0.426222308101129,
1.19471395377504));
#22025=CARTESIAN_POINT('Ctrl Pts',(-4.04878657689504,0.426015612511084,
1.19468977245607));
#22026=CARTESIAN_POINT('Ctrl Pts',(-4.04872369693346,0.425808996580428,
1.19466558266346));
#22027=CARTESIAN_POINT('',(-4.04872369674582,0.083386841251265,1.19466558259128));
#22028=CARTESIAN_POINT('',(-4.04872369693346,0.425808996578679,1.19466558266346));
#22029=CARTESIAN_POINT('',(-4.05990543157618,0.0103940914527843,1.2000161521659));
#22030=CARTESIAN_POINT('Ctrl Pts',(-4.04872369693346,0.0833868071488794,
1.19466558266346));
#22031=CARTESIAN_POINT('Ctrl Pts',(-4.04880141653304,0.0831338820732446,
1.19469548123446));
#22032=CARTESIAN_POINT('Ctrl Pts',(-4.04887876782991,0.0828807524790114,
1.19472538210338));
#22033=CARTESIAN_POINT('Ctrl Pts',(-4.04895570042065,0.0826275846881222,
1.19475526183619));
#22034=CARTESIAN_POINT('Ctrl Pts',(-4.05194285075349,0.0727975472034251,
1.19591543664592));
#22035=CARTESIAN_POINT('Ctrl Pts',(-4.05436347175601,0.062687010783333,
1.19706577060194));
#22036=CARTESIAN_POINT('Ctrl Pts',(-4.05616232857013,0.0524346246710381,
1.19798196717376));
#22037=CARTESIAN_POINT('Ctrl Pts',(-4.05766721379084,0.043857697249005,
1.19874843767289));
#22038=CARTESIAN_POINT('Ctrl Pts',(-4.05873866585706,0.0351814943549607,
1.19935076478133));
#22039=CARTESIAN_POINT('Ctrl Pts',(-4.05934068619687,0.0264871938955073,
1.19969251928842));
#22040=CARTESIAN_POINT('Ctrl Pts',(-4.05971209465163,0.0211233606736628,
1.19990336019361));
#22041=CARTESIAN_POINT('Ctrl Pts',(-4.05990465511051,0.0157526393208265,
1.20001570300931));
#22042=CARTESIAN_POINT('Ctrl Pts',(-4.05990543157618,0.0103940914527843,
1.2000161521659));
#22043=CARTESIAN_POINT('Ctrl Pts',(-4.05987749605595,0.0103667322106564,
1.2));
#22044=CARTESIAN_POINT('Ctrl Pts',(-4.05987749605595,-1.19701232604091E-16,
1.2));
#22045=CARTESIAN_POINT('',(-4.1,-1.17961196366423E-16,1.26933116532693));
#22046=CARTESIAN_POINT('Ctrl Pts',(-4.05987749605677,0.499999999998992,
1.20000000000048));
#22047=CARTESIAN_POINT('Ctrl Pts',(-4.05987749605924,0.499960642899619,
1.2000000000019));
#22048=CARTESIAN_POINT('Ctrl Pts',(-4.05987749606638,0.499921285800245,
1.20000000000603));
#22049=CARTESIAN_POINT('Ctrl Pts',(-4.05987749606638,0.499834371718783,
1.20000000000603));
#22050=CARTESIAN_POINT('Ctrl Pts',(-4.0598774960573,0.499786814736695,1.20000000000078));
#22051=CARTESIAN_POINT('Ctrl Pts',(-4.05987749605608,0.499739257754606,
1.20000000000008));
#22052=CARTESIAN_POINT('Ctrl Pts',(-3.99749546403561,0.425808662442754,
1.12277288952037));
#22053=CARTESIAN_POINT('Ctrl Pts',(-3.99741900307445,0.440723737997244,
1.12056649920249));
#22054=CARTESIAN_POINT('Ctrl Pts',(-3.98925783839562,0.470755634285058,
1.11503732261258));
#22055=CARTESIAN_POINT('Ctrl Pts',(-3.9675518325465,0.493430715073795,1.10823883346629));
#22056=CARTESIAN_POINT('Ctrl Pts',(-3.95471619020724,0.501221222100498,
1.10539530861746));
#22057=CARTESIAN_POINT('Ctrl Pts',(-3.99790114239118,0.425808660873484,
1.13447013611379));
#22058=CARTESIAN_POINT('Ctrl Pts',(-3.99750830618296,0.440793786014735,
1.13248513004705));
#22059=CARTESIAN_POINT('Ctrl Pts',(-3.98845020395956,0.470610844054392,
1.12748649040356));
#22060=CARTESIAN_POINT('Ctrl Pts',(-3.96623032097253,0.491977735388082,
1.12119921453367));
#22061=CARTESIAN_POINT('Ctrl Pts',(-3.95352414898529,0.499091855265921,
1.11853791734794));
#22062=CARTESIAN_POINT('Ctrl Pts',(-4.00394093236138,0.42580863679589,1.15764284313999));
#22063=CARTESIAN_POINT('Ctrl Pts',(-4.00311371590923,0.441868527536911,
1.15623651208263));
#22064=CARTESIAN_POINT('Ctrl Pts',(-3.99226601725672,0.473314772733068,
1.15266048766281));
#22065=CARTESIAN_POINT('Ctrl Pts',(-3.9678344720362,0.49415299798259,1.14800581947106));
#22066=CARTESIAN_POINT('Ctrl Pts',(-3.95443818406651,0.500724592612001,
1.14600324261257));
#22067=CARTESIAN_POINT('Ctrl Pts',(-4.030731649599,0.425808530009691,1.18998205823776));
#22068=CARTESIAN_POINT('Ctrl Pts',(-4.02989922071593,0.446635090392047,
1.18960843288307));
#22069=CARTESIAN_POINT('Ctrl Pts',(-4.01635066531951,0.487487150831074,
1.18865363029091));
#22070=CARTESIAN_POINT('Ctrl Pts',(-3.98472526989518,0.514749615707155,
1.18735776371463));
#22071=CARTESIAN_POINT('Ctrl Pts',(-3.96711397890226,0.523367319030488,
1.18678687783788));
#22072=CARTESIAN_POINT('Ctrl Pts',(-4.05989190797289,0.425808413866688,
1.19999999986964));
#22073=CARTESIAN_POINT('Ctrl Pts',(-4.05957479390507,0.451819306042337,
1.20000581905524));
#22074=CARTESIAN_POINT('Ctrl Pts',(-4.04452566782116,0.503506810044701,
1.1999930990205));
#22075=CARTESIAN_POINT('Ctrl Pts',(-4.00584874486514,0.540239318982905,
1.19998873486588));
#22076=CARTESIAN_POINT('Ctrl Pts',(-3.98334410647183,0.552359067730285,
1.20000004480259));
#22077=CARTESIAN_POINT('Ctrl Pts',(-4.0774473938656,0.425808343825508,1.2));
#22078=CARTESIAN_POINT('Ctrl Pts',(-4.07744751278487,0.454945698277075,
1.2));
#22079=CARTESIAN_POINT('Ctrl Pts',(-4.06151247834833,0.513148697855926,
1.2));
#22080=CARTESIAN_POINT('Ctrl Pts',(-4.018597248821,0.555602008566458,1.2));
#22081=CARTESIAN_POINT('Ctrl Pts',(-3.99313806728599,0.569854029665374,
1.2));
#22082=CARTESIAN_POINT('',(-4.05989001907265,0.49975147889953,1.2));
#22083=CARTESIAN_POINT('',(-3.99749495051979,0.425816408369019,1.12277588236388));
#22084=CARTESIAN_POINT('Ctrl Pts',(-3.95658932953199,0.499868627057285,
1.10580990849871));
#22085=CARTESIAN_POINT('Ctrl Pts',(-3.96360335567988,0.495368835792349,
1.10742680652405));
#22086=CARTESIAN_POINT('Ctrl Pts',(-3.9700453297573,0.489837933598796,1.10919755141692));
#22087=CARTESIAN_POINT('Ctrl Pts',(-3.97558141221856,0.483497827408914,
1.11098169097766));
#22088=CARTESIAN_POINT('Ctrl Pts',(-3.97694492583232,0.481936286163253,
1.11142111697916));
#22089=CARTESIAN_POINT('Ctrl Pts',(-3.97825354811615,0.480325670155073,
1.11186112444703));
#22090=CARTESIAN_POINT('Ctrl Pts',(-3.97950242686639,0.478669304998406,
1.11229909409945));
#22091=CARTESIAN_POINT('Ctrl Pts',(-3.9818456702272,0.475561503976319,1.11312084679567));
#22092=CARTESIAN_POINT('Ctrl Pts',(-3.98397855806195,0.472292666317773,
1.11393570752481));
#22093=CARTESIAN_POINT('Ctrl Pts',(-3.98588913947764,0.468903558492556,
1.11472661791731));
#22094=CARTESIAN_POINT('Ctrl Pts',(-3.98989952307469,0.46178969131097,1.11638676913556));
#22095=CARTESIAN_POINT('Ctrl Pts',(-3.99293173507827,0.454148826888769,
1.11794762353363));
#22096=CARTESIAN_POINT('Ctrl Pts',(-3.99489269458943,0.446280500947391,
1.11938837303024));
#22097=CARTESIAN_POINT('Ctrl Pts',(-3.99656653497968,0.439564236950421,
1.12061817134373));
#22098=CARTESIAN_POINT('Ctrl Pts',(-3.997459613396,0.432681349848232,1.12175934133402));
#22099=CARTESIAN_POINT('Ctrl Pts',(-3.99749495051979,0.425816408369019,
1.12277588236388));
#22100=CARTESIAN_POINT('Origin',(-4.07744739386693,0.425808996578679,1.12));
#22101=CARTESIAN_POINT('Origin',(4.1,0.,1.2));
#22102=CARTESIAN_POINT('Origin',(-3.91744442112685,0.0831608766898327,1.20000000000032));
#22103=CARTESIAN_POINT('Origin',(4.1,0.,1.2));
#22104=CARTESIAN_POINT('Origin',(-4.1,0.,1.2));
#22105=CARTESIAN_POINT('Ctrl Pts',(-4.04872369777422,0.425808996578679,
1.1946655829869));
#22106=CARTESIAN_POINT('Ctrl Pts',(-4.04872369777422,0.0149024691460445,
1.1946655829869));
#22107=CARTESIAN_POINT('Ctrl Pts',(-4.03417809695481,0.425808996578679,
1.18906992029053));
#22108=CARTESIAN_POINT('Ctrl Pts',(-4.03417809695481,0.0149024691460445,
1.18906992029053));
#22109=CARTESIAN_POINT('Ctrl Pts',(-4.00850642174527,0.425808996578679,
1.16912611569929));
#22110=CARTESIAN_POINT('Ctrl Pts',(-4.00850642174527,0.0149024691460445,
1.16912611569929));
#22111=CARTESIAN_POINT('Ctrl Pts',(-3.9980360657665,0.425808996578679,1.1383501202594));
#22112=CARTESIAN_POINT('Ctrl Pts',(-3.9980360657665,0.0149024691460445,
1.1383501202594));
#22113=CARTESIAN_POINT('Ctrl Pts',(-3.99749552679662,0.425808996578679,
1.12277469853698));
#22114=CARTESIAN_POINT('Ctrl Pts',(-3.99749552679662,0.0149024691460445,
1.12277469853698));
#22115=CARTESIAN_POINT('',(-3.99749552930111,0.08338687277103,1.12277470064702));
#22116=CARTESIAN_POINT('',(-3.99749552679662,0.425808996578679,1.12277469853698));
#22117=CARTESIAN_POINT('Origin',(-4.07744739386693,0.0833868903848169,1.12));
#22118=CARTESIAN_POINT('Ctrl Pts',(-3.91780246449684,0.00300376307205705,
1.1265306122449));
#22119=CARTESIAN_POINT('Ctrl Pts',(-3.93576025037965,0.00296202866725982,
1.12704015241118));
#22120=CARTESIAN_POINT('Ctrl Pts',(-3.96555870066537,0.0134692513665733,
1.12719733238845));
#22121=CARTESIAN_POINT('Ctrl Pts',(-3.99216195295547,0.0472952052376165,
1.12560552323969));
#22122=CARTESIAN_POINT('Ctrl Pts',(-3.99753261370091,0.0713291405834686,
1.12384334179573));
#22123=CARTESIAN_POINT('Ctrl Pts',(-3.99749552679548,0.0833868069155861,
1.12277469850418));
#22124=CARTESIAN_POINT('Ctrl Pts',(-3.91780246449684,0.00115146656907868,
1.14914551409197));
#22125=CARTESIAN_POINT('Ctrl Pts',(-3.93613149057372,0.000969237935352311,
1.14954546365303));
#22126=CARTESIAN_POINT('Ctrl Pts',(-3.96686365991627,0.0118424389758149,
1.14966515106411));
#22127=CARTESIAN_POINT('Ctrl Pts',(-3.99366630482309,0.0466900216982605,
1.14841701955119));
#22128=CARTESIAN_POINT('Ctrl Pts',(-3.99865916988022,0.0712429843090682,
1.14702096166311));
#22129=CARTESIAN_POINT('Ctrl Pts',(-3.99830738013179,0.0833868069192833,
1.14616793922152));
#22130=CARTESIAN_POINT('Ctrl Pts',(-3.91780246449684,-0.0199489376043931,
1.18690998941925));
#22131=CARTESIAN_POINT('Ctrl Pts',(-3.94093194698948,-0.0201921648247794,
1.18702695697395));
#22132=CARTESIAN_POINT('Ctrl Pts',(-3.97951730409342,-0.00666843160596345,
1.18706431777373));
#22133=CARTESIAN_POINT('Ctrl Pts',(-4.01329298538155,0.0373349474711074,
1.18669970306998));
#22134=CARTESIAN_POINT('Ctrl Pts',(-4.01937761864352,0.0681485596815143,
1.18628923992153));
#22135=CARTESIAN_POINT('Ctrl Pts',(-4.01886907034338,0.0833868070129213,
1.18603556032283));
#22136=CARTESIAN_POINT('Ctrl Pts',(-3.91780246449684,-0.0597112616448693,
1.2));
#22137=CARTESIAN_POINT('Ctrl Pts',(-3.94986432816707,-0.0597837540420209,
1.19999893991423));
#22138=CARTESIAN_POINT('Ctrl Pts',(-4.00315043136341,-0.0410040343800299,
1.19999296250002));
#22139=CARTESIAN_POINT('Ctrl Pts',(-4.05061466200189,0.0193832087506108,
1.19999621445595));
#22140=CARTESIAN_POINT('Ctrl Pts',(-4.0600434134887,0.0620661620497311,
1.19999748313998));
#22141=CARTESIAN_POINT('Ctrl Pts',(-4.0598919008628,0.0833868071997395,
1.2));
#22142=CARTESIAN_POINT('Ctrl Pts',(-3.91780246449684,-0.0767292357659823,
1.2));
#22143=CARTESIAN_POINT('Ctrl Pts',(-3.95368317895231,-0.0767292357659822,
1.2));
#22144=CARTESIAN_POINT('Ctrl Pts',(-4.01326936269294,-0.0556897214928556,
1.2));
#22145=CARTESIAN_POINT('Ctrl Pts',(-4.06658466073547,0.0117033247253155,
1.2));
#22146=CARTESIAN_POINT('Ctrl Pts',(-4.07744739397586,0.0594663309760329,
1.2));
#22147=CARTESIAN_POINT('Ctrl Pts',(-4.07744739386693,0.0833868072796873,
1.2));
#22148=CARTESIAN_POINT('Ctrl Pts',(-3.99749552679548,0.0833868069155861,
1.12277469850418));
#22149=CARTESIAN_POINT('Ctrl Pts',(-3.99753261370091,0.0713291405834686,
1.12384334179573));
#22150=CARTESIAN_POINT('Ctrl Pts',(-3.99216195295547,0.0472952052376165,
1.12560552323969));
#22151=CARTESIAN_POINT('Ctrl Pts',(-3.96555870066537,0.0134692513665733,
1.12719733238845));
#22152=CARTESIAN_POINT('Ctrl Pts',(-3.93576025037965,0.00296202866725982,
1.12704015241118));
#22153=CARTESIAN_POINT('Ctrl Pts',(-3.91780246449684,0.00300376307205705,
1.1265306122449));
#22154=CARTESIAN_POINT('Ctrl Pts',(-3.9199627360209,0.5,1.2));
#22155=CARTESIAN_POINT('Ctrl Pts',(-3.91859147059112,0.5,1.16263028970545));
#22156=CARTESIAN_POINT('Ctrl Pts',(-3.91708574929206,0.505271087920178,
1.12526784524295));
#22157=CARTESIAN_POINT('Ctrl Pts',(-3.91539217619132,0.515604560956495,
1.08936480468426));
#22158=CARTESIAN_POINT('Ctrl Pts',(-3.94388749707654,0.5,1.1992684093282));
#22159=CARTESIAN_POINT('Ctrl Pts',(-3.94255922360763,0.500070437490442,
1.16187406103769));
#22160=CARTESIAN_POINT('Ctrl Pts',(-3.94110090415831,0.505425615700251,
1.12441169682652));
#22161=CARTESIAN_POINT('Ctrl Pts',(-3.93947649219532,0.515856199601771,
1.08849050110252));
#22162=CARTESIAN_POINT('Ctrl Pts',(-3.98530151225888,0.479904100518027,
1.19800201811456));
#22163=CARTESIAN_POINT('Ctrl Pts',(-3.98404149316127,0.480012713029783,
1.15861674257998));
#22164=CARTESIAN_POINT('Ctrl Pts',(-3.98266889977967,0.485680432111213,
1.11922733796895));
#22165=CARTESIAN_POINT('Ctrl Pts',(-3.98115396081513,0.496695221132957,
1.08133736541183));
#22166=CARTESIAN_POINT('Ctrl Pts',(-3.99992535969115,0.437951958020513,
1.19755483829351));
#22167=CARTESIAN_POINT('Ctrl Pts',(-3.99860101206523,0.437984309190483,
1.15422623809305));
#22168=CARTESIAN_POINT('Ctrl Pts',(-3.9971480185017,0.444112318340178,1.11085352703736));
#22169=CARTESIAN_POINT('Ctrl Pts',(-3.99552667887377,0.456097443939778,
1.06908769510471));
#22170=CARTESIAN_POINT('Ctrl Pts',(-3.99992535969115,0.42,1.19755483829351));
#22171=CARTESIAN_POINT('Ctrl Pts',(-3.99854929471383,0.42,1.15255422928056));
#22172=CARTESIAN_POINT('Ctrl Pts',(-3.99703626487076,0.426325305504265,
1.10749080430861));
#22173=CARTESIAN_POINT('Ctrl Pts',(-3.99533043997794,0.438725473147794,
1.06409547620398));
#22174=CARTESIAN_POINT('',(-3.91539217619132,0.515604560956495,1.08936480468426));
#22175=CARTESIAN_POINT('Ctrl Pts',(-3.9199627360209,0.5,1.2));
#22176=CARTESIAN_POINT('Ctrl Pts',(-3.91859147059112,0.5,1.16263028970545));
#22177=CARTESIAN_POINT('Ctrl Pts',(-3.91708574929206,0.505271087920178,
1.12526784524295));
#22178=CARTESIAN_POINT('Ctrl Pts',(-3.91539217619132,0.515604560956495,
1.08936480468426));
#22179=CARTESIAN_POINT('',(-3.99533043998062,0.438725473135619,1.06409547624199));
#22180=CARTESIAN_POINT('Origin',(-3.91539217619132,0.438725473147794,1.06723776562112));
#22181=CARTESIAN_POINT('Origin',(-3.98259956593766,0.90718624733336,1.19842150873233));
#22182=CARTESIAN_POINT('Ctrl Pts',(-3.99642658272504,0.44384037918325,1.04839302148096));
#22183=CARTESIAN_POINT('Ctrl Pts',(-3.99548774892012,0.44179052725272,1.05345171612862));
#22184=CARTESIAN_POINT('Ctrl Pts',(-3.99511937952587,0.440067061234499,
1.05872620436003));
#22185=CARTESIAN_POINT('Ctrl Pts',(-3.99533043997794,0.438725473147794,
1.06409547620398));
#22186=CARTESIAN_POINT('Ctrl Pts',(-3.99657534106213,0.466413555729877,
1.05663619619587));
#22187=CARTESIAN_POINT('Ctrl Pts',(-3.99579563594237,0.464642772895823,
1.06121182233657));
#22188=CARTESIAN_POINT('Ctrl Pts',(-3.99546531235558,0.463114794501233,
1.06596374902201));
#22189=CARTESIAN_POINT('Ctrl Pts',(-3.99559209183904,0.461888100870439,
1.07075176807162));
#22190=CARTESIAN_POINT('Ctrl Pts',(-3.97685954371716,0.50677512210794,1.06772025968478));
#22191=CARTESIAN_POINT('Ctrl Pts',(-3.97592643102433,0.505042447302577,
1.07279579186463));
#22192=CARTESIAN_POINT('Ctrl Pts',(-3.97553510541324,0.503447592943445,
1.07789416781835));
#22193=CARTESIAN_POINT('Ctrl Pts',(-3.97566885922969,0.501970835818075,
1.08307138584241));
#22194=CARTESIAN_POINT('Ctrl Pts',(-3.93534760874179,0.523078681693286,
1.06606105089355));
#22195=CARTESIAN_POINT('Ctrl Pts',(-3.93375572569525,0.520454986989424,
1.07347568016643));
#22196=CARTESIAN_POINT('Ctrl Pts',(-3.93312277810201,0.518010117677892,
1.08106604861408));
#22197=CARTESIAN_POINT('Ctrl Pts',(-3.93345541319432,0.515793289940452,
1.08870907699796));
#22198=CARTESIAN_POINT('Ctrl Pts',(-3.91758436243186,0.524122951685319,
1.06319194267061));
#22199=CARTESIAN_POINT('Ctrl Pts',(-3.91571147604617,0.521017369008945,
1.07172446094826));
#22200=CARTESIAN_POINT('Ctrl Pts',(-3.91497483111678,0.518151025630959,
1.08051726386549));
#22201=CARTESIAN_POINT('Ctrl Pts',(-3.91539217619132,0.515604560956495,
1.08936480468426));
#22202=CARTESIAN_POINT('',(-3.91758436243186,0.524122951685478,1.06319194267017));
#22203=CARTESIAN_POINT('Origin',(-4.02330412568762,0.546067694126366,1.09055042993106));
#22204=CARTESIAN_POINT('',(-3.99642658272504,0.443840379183073,1.04839302148084));
#22205=CARTESIAN_POINT('Origin',(-3.91758436243186,0.448947542022383,1.03583033120473));
#22206=CARTESIAN_POINT('Origin',(-4.05033769991219,0.474821566285832,1.0709707385159));
#22207=CARTESIAN_POINT('Ctrl Pts',(-2.87962408435655,0.450506079619966,
1.031548284348));
#22208=CARTESIAN_POINT('Ctrl Pts',(-2.88706985293045,0.495141499993335,
0.908913474764299));
#22209=CARTESIAN_POINT('Ctrl Pts',(-2.89830085190713,0.584802360144796,
0.662572286089282));
#22210=CARTESIAN_POINT('Ctrl Pts',(-2.92033299964242,0.698627090634836,
0.349841409292389));
#22211=CARTESIAN_POINT('Ctrl Pts',(-2.97414103030473,0.773765776974324,
0.143399565247164));
#22212=CARTESIAN_POINT('Ctrl Pts',(-3.02113993649286,0.805536061367637,
0.0561114262668838));
#22213=CARTESIAN_POINT('Ctrl Pts',(-3.04982829439264,0.821130183736138,
0.0132669271832156));
#22214=CARTESIAN_POINT('Ctrl Pts',(-3.09662700629875,0.839948596127357,
-0.0384362359316435));
#22215=CARTESIAN_POINT('Ctrl Pts',(-3.20078875895428,0.862136521381471,
-0.0993970595518691));
#22216=CARTESIAN_POINT('Ctrl Pts',(-3.33746877961289,0.868528535167059,
-0.116958973092616));
#22217=CARTESIAN_POINT('Ctrl Pts',(-3.48441332396274,0.862274358796636,
-0.0997757647375922));
#22218=CARTESIAN_POINT('Ctrl Pts',(-3.61382529190729,0.84783025941325,-0.0600909278373817));
#22219=CARTESIAN_POINT('Ctrl Pts',(-3.72587585229285,0.825571951670826,
0.0010632700802009));
#22220=CARTESIAN_POINT('Ctrl Pts',(-3.84060061269669,0.786540385741618,
0.108301616116654));
#22221=CARTESIAN_POINT('Ctrl Pts',(-3.90217403729928,0.738739795172645,
0.239632659341502));
#22222=CARTESIAN_POINT('Ctrl Pts',(-3.93815958139645,0.692207019220546,
0.367480410534435));
#22223=CARTESIAN_POINT('Ctrl Pts',(-3.96327795090667,0.645584422821145,
0.495574941378137));
#22224=CARTESIAN_POINT('Ctrl Pts',(-3.988190288963,0.56591300759988,0.714470355674555));
#22225=CARTESIAN_POINT('Ctrl Pts',(-3.99552195740115,0.49833669404846,0.900134751247067));
#22226=CARTESIAN_POINT('Ctrl Pts',(-3.99961373290197,0.453243799876031,
1.02402645976367));
#22227=CARTESIAN_POINT('Ctrl Pts',(-2.87962408435655,0.472998509594012,
1.03973485935487));
#22228=CARTESIAN_POINT('Ctrl Pts',(-2.88706972471758,0.517633161364987,
0.917102161488891));
#22229=CARTESIAN_POINT('Ctrl Pts',(-2.89829720228894,0.607291613669455,
0.670767588319117));
#22230=CARTESIAN_POINT('Ctrl Pts',(-2.92029355131071,0.72110022589572,0.358080996087986));
#22231=CARTESIAN_POINT('Ctrl Pts',(-2.9740705062357,0.796239021043994,0.151638853093076));
#22232=CARTESIAN_POINT('Ctrl Pts',(-3.02108238010733,0.828022541036071,
0.0643143496040615));
#22233=CARTESIAN_POINT('Ctrl Pts',(-3.04978340300042,0.843624632566539,
0.0214479554278384));
#22234=CARTESIAN_POINT('Ctrl Pts',(-3.096592410354,0.862452712083289,-0.0302817678961312));
#22235=CARTESIAN_POINT('Ctrl Pts',(-3.20082556389089,0.884655834508208,
-0.0912843453999811));
#22236=CARTESIAN_POINT('Ctrl Pts',(-3.33748082734155,0.891040050440225,
-0.108824834514122));
#22237=CARTESIAN_POINT('Ctrl Pts',(-3.48443609473601,0.884781674811433,
-0.0916300887915507));
#22238=CARTESIAN_POINT('Ctrl Pts',(-3.61385184322647,0.870335933837343,
-0.051940741657948));
#22239=CARTESIAN_POINT('Ctrl Pts',(-3.72590622690082,0.84807391828105,0.00922364339451449));
#22240=CARTESIAN_POINT('Ctrl Pts',(-3.84068731705383,0.809022827244695,
0.116515634221966));
#22241=CARTESIAN_POINT('Ctrl Pts',(-3.90219876188619,0.761230212281178,
0.247824764650918));
#22242=CARTESIAN_POINT('Ctrl Pts',(-3.93818741165077,0.714691426981262,
0.375689026391285));
#22243=CARTESIAN_POINT('Ctrl Pts',(-3.96329567170119,0.668068278176157,
0.503785074957183));
#22244=CARTESIAN_POINT('Ctrl Pts',(-3.98820643523393,0.588393873042911,
0.722688703969256));
#22245=CARTESIAN_POINT('Ctrl Pts',(-3.99552190872555,0.520829660445818,
0.908319852442999));
#22246=CARTESIAN_POINT('Ctrl Pts',(-3.99961373290197,0.475736229850077,
1.03221303477054));
#22247=CARTESIAN_POINT('Ctrl Pts',(-2.89968712497522,0.511541907490879,
1.05498163579157));
#22248=CARTESIAN_POINT('Ctrl Pts',(-2.90714300575565,0.556237947877504,
0.932180274090282));
#22249=CARTESIAN_POINT('Ctrl Pts',(-2.9183967840909,0.645941625439093,0.685721445547777));
#22250=CARTESIAN_POINT('Ctrl Pts',(-2.94035557430995,0.759332481137342,
0.374182629944202));
#22251=CARTESIAN_POINT('Ctrl Pts',(-2.99348007913718,0.833071760243458,
0.171585625673285));
#22252=CARTESIAN_POINT('Ctrl Pts',(-3.03867906787114,0.863582657829508,
0.0877576235083202));
#22253=CARTESIAN_POINT('Ctrl Pts',(-3.06601334262966,0.878445385572726,
0.0469226146423277));
#22254=CARTESIAN_POINT('Ctrl Pts',(-3.11011593586453,0.896118505150049,
-0.00163388232768946));
#22255=CARTESIAN_POINT('Ctrl Pts',(-3.20700850686946,0.916796373054912,
-0.058445857478767));
#22256=CARTESIAN_POINT('Ctrl Pts',(-3.33712049077176,0.923017161010362,
-0.0755373319175819));
#22257=CARTESIAN_POINT('Ctrl Pts',(-3.48002463105222,0.916949465597777,
-0.0588664757833766));
#22258=CARTESIAN_POINT('Ctrl Pts',(-3.60584634368539,0.9028960189969,-0.0202549485819569));
#22259=CARTESIAN_POINT('Ctrl Pts',(-3.71361989979722,0.881446144267468,
0.0386780978872879));
#22260=CARTESIAN_POINT('Ctrl Pts',(-3.82318598076471,0.844187728138539,
0.141044754886167));
#22261=CARTESIAN_POINT('Ctrl Pts',(-3.88312165251306,0.797918873417564,
0.26816738845607));
#22262=CARTESIAN_POINT('Ctrl Pts',(-3.91850643383034,0.752156053042667,
0.393899704086659));
#22263=CARTESIAN_POINT('Ctrl Pts',(-3.94333901415249,0.70609879889664,0.52044096985495));
#22264=CARTESIAN_POINT('Ctrl Pts',(-3.96810955084563,0.626950470316382,
0.737899215416785));
#22265=CARTESIAN_POINT('Ctrl Pts',(-3.97543979982371,0.559508505904016,
0.923194489763422));
#22266=CARTESIAN_POINT('Ctrl Pts',(-3.97952773625812,0.514457919677186,
1.04696995815483));
#22267=CARTESIAN_POINT('Ctrl Pts',(-2.9415713861866,0.524472685894761,1.06223105582735));
#22268=CARTESIAN_POINT('Ctrl Pts',(-2.94904828921471,0.569294749116044,
0.93908344923351));
#22269=CARTESIAN_POINT('Ctrl Pts',(-2.96034719658121,0.659086154935045,
0.692383589284719));
#22270=CARTESIAN_POINT('Ctrl Pts',(-2.98212818142746,0.77156013548705,0.383363867441909));
#22271=CARTESIAN_POINT('Ctrl Pts',(-3.03380432716909,0.84237804114237,0.188793270760848));
#22272=CARTESIAN_POINT('Ctrl Pts',(-3.07525468269643,0.870268919584971,
0.112163712031047));
#22273=CARTESIAN_POINT('Ctrl Pts',(-3.0997708540493,0.883610253909479,0.0755086972290682));
#22274=CARTESIAN_POINT('Ctrl Pts',(-3.13825203413196,0.898899082374074,
0.0335029862526778));
#22275=CARTESIAN_POINT('Ctrl Pts',(-3.22001841149168,0.916434974427251,
-0.0146764811934207));
#22276=CARTESIAN_POINT('Ctrl Pts',(-3.33640169127941,0.922292933767806,
-0.0307710922056808));
#22277=CARTESIAN_POINT('Ctrl Pts',(-3.47087833872087,0.916611649236276,
-0.0151618912418065));
#22278=CARTESIAN_POINT('Ctrl Pts',(-3.58920752111338,0.903372611293106,
0.0212120665623573));
#22279=CARTESIAN_POINT('Ctrl Pts',(-3.68805489678656,0.883607893498353,
0.0755151824053357));
#22280=CARTESIAN_POINT('Ctrl Pts',(-3.78689035517007,0.85003771211992,0.167748497709577));
#22281=CARTESIAN_POINT('Ctrl Pts',(-3.84336430236995,0.8069720537749,0.286070421566467));
#22282=CARTESIAN_POINT('Ctrl Pts',(-3.87749705111799,0.762812478046415,
0.407397858733175));
#22283=CARTESIAN_POINT('Ctrl Pts',(-3.90172604413317,0.717935070365446,
0.530697522980297));
#22284=CARTESIAN_POINT('Ctrl Pts',(-3.92619946695966,0.639876694845063,
0.745161147121859));
#22285=CARTESIAN_POINT('Ctrl Pts',(-3.93351559588986,0.572723538474725,
0.929662927894466));
#22286=CARTESIAN_POINT('Ctrl Pts',(-3.93759555129614,0.527760906158602,
1.05319674490226));
#22287=CARTESIAN_POINT('Ctrl Pts',(-2.9594941977123,0.524122950641471,1.06319194553855));
#22288=CARTESIAN_POINT('Ctrl Pts',(-2.96698008492688,0.568998871692987,
0.939896365772286));
#22289=CARTESIAN_POINT('Ctrl Pts',(-2.9782979876664,0.658827601540248,0.693093958898646));
#22290=CARTESIAN_POINT('Ctrl Pts',(-2.99999967569416,0.770907793456571,
0.38515616244041));
#22291=CARTESIAN_POINT('Ctrl Pts',(-3.05105326213358,0.840475615777891,
0.194020141491951));
#22292=CARTESIAN_POINT('Ctrl Pts',(-3.09090069290084,0.867246541900823,
0.12046762647131));
#22293=CARTESIAN_POINT('Ctrl Pts',(-3.11421209795167,0.879937567446779,
0.0855993203540729));
#22294=CARTESIAN_POINT('Ctrl Pts',(-3.15028872702707,0.894206994493787,
0.0463943917538627));
#22295=CARTESIAN_POINT('Ctrl Pts',(-3.22558881811219,0.910399758249608,
0.00190513897618206));
#22296=CARTESIAN_POINT('Ctrl Pts',(-3.3360951886178,0.916101759009581,-0.0137609793575587));
#22297=CARTESIAN_POINT('Ctrl Pts',(-3.46696656599506,0.910585447910795,
0.00139496082504257));
#22298=CARTESIAN_POINT('Ctrl Pts',(-3.58208993795251,0.897694758584722,
0.0368118386696318));
#22299=CARTESIAN_POINT('Ctrl Pts',(-3.67711802975361,0.878650808373231,
0.089134661852922));
#22300=CARTESIAN_POINT('Ctrl Pts',(-3.77136677090444,0.846657118193748,
0.177036603186079));
#22301=CARTESIAN_POINT('Ctrl Pts',(-3.82635384144273,0.804962864100056,
0.2915906248295));
#22302=CARTESIAN_POINT('Ctrl Pts',(-3.85995110804723,0.761488798159762,
0.411034639332341));
#22303=CARTESIAN_POINT('Ctrl Pts',(-3.88392091137359,0.717116212326026,
0.532947316953341));
#22304=CARTESIAN_POINT('Ctrl Pts',(-3.90826705411741,0.639523973437174,
0.746130241225391));
#22305=CARTESIAN_POINT('Ctrl Pts',(-3.91557568799506,0.572495487342456,
0.930289493230857));
#22306=CARTESIAN_POINT('Ctrl Pts',(-3.91965223258409,0.527570443506261,
1.05372003673881));
#22307=CARTESIAN_POINT('',(-2.88729704002952,0.500000000328437,0.895564854801195));
#22308=CARTESIAN_POINT('Ctrl Pts',(-2.88715652162958,0.500000000004701,
0.898556263621882));
#22309=CARTESIAN_POINT('Ctrl Pts',(-2.88720339858619,0.499999999361646,
0.897559129110793));
#22310=CARTESIAN_POINT('Ctrl Pts',(-2.88725023764408,0.499999999368085,
0.896561992815236));
#22311=CARTESIAN_POINT('Ctrl Pts',(-2.88729704002392,0.500000000000096,
0.895564854800933));
#22312=CARTESIAN_POINT('',(-3.99961373290197,0.453243799876042,1.02402645976365));
#22313=CARTESIAN_POINT('Ctrl Pts',(-2.88729704002952,0.500000000328437,
0.895564854801195));
#22314=CARTESIAN_POINT('Ctrl Pts',(-2.88906965512591,0.512137783677987,
0.862216569126075));
#22315=CARTESIAN_POINT('Ctrl Pts',(-2.89078934467508,0.52428817848214,0.828833633764207));
#22316=CARTESIAN_POINT('Ctrl Pts',(-2.89253615105346,0.536464830009127,
0.795378558649242));
#22317=CARTESIAN_POINT('Ctrl Pts',(-2.89381761055983,0.545397637931103,
0.770835870591288));
#22318=CARTESIAN_POINT('Ctrl Pts',(-2.89511395407221,0.554344395792644,
0.746254855389374));
#22319=CARTESIAN_POINT('Ctrl Pts',(-2.89646663063639,0.563304917550206,
0.721636024193941));
#22320=CARTESIAN_POINT('Ctrl Pts',(-2.89734121067155,0.569098389279699,
0.705718591436909));
#22321=CARTESIAN_POINT('Ctrl Pts',(-2.89823953190499,0.574897507579613,
0.689785644855149));
#22322=CARTESIAN_POINT('Ctrl Pts',(-2.89917526582012,0.580700853337509,
0.673841083428042));
#22323=CARTESIAN_POINT('Ctrl Pts',(-2.89971479707597,0.584046982375097,
0.664647669454688));
#22324=CARTESIAN_POINT('Ctrl Pts',(-2.90026689066681,0.587394941514684,
0.655449227317415));
#22325=CARTESIAN_POINT('Ctrl Pts',(-2.90083359406858,0.590739208495519,
0.646260929302945));
#22326=CARTESIAN_POINT('Ctrl Pts',(-2.90240528294206,0.600014161120397,
0.620778206399581));
#22327=CARTESIAN_POINT('Ctrl Pts',(-2.90408968664164,0.609274396150569,
0.595335919755338));
#22328=CARTESIAN_POINT('Ctrl Pts',(-2.90597098506406,0.618563414427602,
0.56981455179029));
#22329=CARTESIAN_POINT('Ctrl Pts',(-2.90768551128761,0.627028985459456,
0.546555586537481));
#22330=CARTESIAN_POINT('Ctrl Pts',(-2.90956331501266,0.635518588868317,
0.523230592871512));
#22331=CARTESIAN_POINT('Ctrl Pts',(-2.91168894974053,0.644054012119428,
0.499779710223596));
#22332=CARTESIAN_POINT('Ctrl Pts',(-2.91366705538124,0.651997036693419,
0.477956429564381));
#22333=CARTESIAN_POINT('Ctrl Pts',(-2.91585960531524,0.659979843146529,
0.456023849090585));
#22334=CARTESIAN_POINT('Ctrl Pts',(-2.9183567293491,0.668008257167524,0.43396596285387));
#22335=CARTESIAN_POINT('Ctrl Pts',(-2.92077093488793,0.675770082905733,
0.412640521904397));
#22336=CARTESIAN_POINT('Ctrl Pts',(-2.92346955517842,0.683574699361931,
0.391197514423489));
#22337=CARTESIAN_POINT('Ctrl Pts',(-2.92655871267213,0.691414026493946,
0.369659140144562));
#22338=CARTESIAN_POINT('Ctrl Pts',(-2.92955133399416,0.699008374653085,
0.348793840061851));
#22339=CARTESIAN_POINT('Ctrl Pts',(-2.93291025093034,0.70663544629957,0.327838632936568));
#22340=CARTESIAN_POINT('Ctrl Pts',(-2.9367590113504,0.714272904796163,0.306854888175159));
#22341=CARTESIAN_POINT('Ctrl Pts',(-2.93885689266313,0.718435928655275,
0.295417074125599));
#22342=CARTESIAN_POINT('Ctrl Pts',(-2.94110120212796,0.722602382083406,
0.283969837412598));
#22343=CARTESIAN_POINT('Ctrl Pts',(-2.94351389087306,0.726763244431991,
0.272537962064403));
#22344=CARTESIAN_POINT('Ctrl Pts',(-2.94661866850662,0.732117665876711,
0.25782681005079));
#22345=CARTESIAN_POINT('Ctrl Pts',(-2.95000336005515,0.737468874357662,
0.243124485582583));
#22346=CARTESIAN_POINT('Ctrl Pts',(-2.95376109050901,0.742841037534281,
0.228364588561198));
#22347=CARTESIAN_POINT('Ctrl Pts',(-2.95729395081782,0.747891719665993,
0.214487953451476));
#22348=CARTESIAN_POINT('Ctrl Pts',(-2.96115642045917,0.752961014265982,
0.200560181005442));
#22349=CARTESIAN_POINT('Ctrl Pts',(-2.96544977445503,0.758055775150981,
0.186562440516388));
#22350=CARTESIAN_POINT('Ctrl Pts',(-2.96952289573906,0.762889194202305,
0.173282730814113));
#22351=CARTESIAN_POINT('Ctrl Pts',(-2.97398373546562,0.767745620448862,
0.159939809362452));
#22352=CARTESIAN_POINT('Ctrl Pts',(-2.97894249446087,0.772617350031455,
0.14655484234059));
#22353=CARTESIAN_POINT('Ctrl Pts',(-2.98370439589809,0.777295677032889,
0.133701244543323));
#22354=CARTESIAN_POINT('Ctrl Pts',(-2.98892541390208,0.781988195935133,
0.120808654819044));
#22355=CARTESIAN_POINT('Ctrl Pts',(-2.99472675076426,0.78667401504634,0.107934472619355));
#22356=CARTESIAN_POINT('Ctrl Pts',(-2.99762127725687,0.789011963674251,
0.101511011556323));
#22357=CARTESIAN_POINT('Ctrl Pts',(-3.00066060816065,0.791347981754224,
0.0950928546301593));
#22358=CARTESIAN_POINT('Ctrl Pts',(-3.00386228892887,0.793678090217947,
0.0886909342412002));
#22359=CARTESIAN_POINT('Ctrl Pts',(-3.00948082270016,0.797767127833499,
0.0774563957251705));
#22360=CARTESIAN_POINT('Ctrl Pts',(-3.01561191556197,0.801849220402643,
0.0662409385673262));
#22361=CARTESIAN_POINT('Ctrl Pts',(-3.0223851741983,0.805900395663406,0.055110426016126));
#22362=CARTESIAN_POINT('Ctrl Pts',(-3.02782556918369,0.809154367607626,
0.0461702115758429));
#22363=CARTESIAN_POINT('Ctrl Pts',(-3.03368223245992,0.812389485062581,
0.0372817994190711));
#22364=CARTESIAN_POINT('Ctrl Pts',(-3.0400481045814,0.81559153492332,0.0284842397307234));
#22365=CARTESIAN_POINT('Ctrl Pts',(-3.04611577676524,0.818643589457321,
0.0200987888156099));
#22366=CARTESIAN_POINT('Ctrl Pts',(-3.05265301996243,0.821667341345101,
0.0117910987819022));
#22367=CARTESIAN_POINT('Ctrl Pts',(-3.05969044973315,0.824619391171969,
0.00368040854147765));
#22368=CARTESIAN_POINT('Ctrl Pts',(-3.06690597848203,0.82764614967441,-0.0046355420981232));
#22369=CARTESIAN_POINT('Ctrl Pts',(-3.07464711940229,0.83059711117744,-0.0127432421933774));
#22370=CARTESIAN_POINT('Ctrl Pts',(-3.08293432214086,0.833428549750499,
-0.0205225557374285));
#22371=CARTESIAN_POINT('Ctrl Pts',(-3.08900359713866,0.835502202330433,
-0.0262198693765905));
#22372=CARTESIAN_POINT('Ctrl Pts',(-3.09536426361141,0.837511450702421,
-0.0317402339087038));
#22373=CARTESIAN_POINT('Ctrl Pts',(-3.102023294888,0.839442269732748,-0.0370451155955819));
#22374=CARTESIAN_POINT('Ctrl Pts',(-3.1094340557817,0.841591056480911,-0.0429488586653822));
#22375=CARTESIAN_POINT('Ctrl Pts',(-3.11722060609208,0.8436428828278,-0.0485862052221031));
#22376=CARTESIAN_POINT('Ctrl Pts',(-3.12529583871742,0.845562886609632,
-0.0538613722579536));
#22377=CARTESIAN_POINT('Ctrl Pts',(-3.13341782061337,0.847494005709194,
-0.0591670783782781));
#22378=CARTESIAN_POINT('Ctrl Pts',(-3.14183173807261,0.849291747731165,
-0.0641063339896468));
#22379=CARTESIAN_POINT('Ctrl Pts',(-3.15042212018654,0.850936379853183,
-0.0686249236082001));
#22380=CARTESIAN_POINT('Ctrl Pts',(-3.15734806920517,0.852262355587489,
-0.0722680119969508));
#22381=CARTESIAN_POINT('Ctrl Pts',(-3.1643881120949,0.853489141241828,-0.0756385778807585));
#22382=CARTESIAN_POINT('Ctrl Pts',(-3.17147060890108,0.854613538175338,
-0.0787278330660827));
#22383=CARTESIAN_POINT('Ctrl Pts',(-3.18024623377992,0.856006731278484,
-0.0825555996579158));
#22384=CARTESIAN_POINT('Ctrl Pts',(-3.18907687523737,0.857242188179029,
-0.0859499895948705));
#22385=CARTESIAN_POINT('Ctrl Pts',(-3.19793312265248,0.858337868433289,
-0.0889603463523945));
#22386=CARTESIAN_POINT('Ctrl Pts',(-3.2131925497421,0.860225739465991,-0.0941472293855846));
#22387=CARTESIAN_POINT('Ctrl Pts',(-3.22852785907475,0.86169972756608,-0.0981969784071248));
#22388=CARTESIAN_POINT('Ctrl Pts',(-3.24381982804354,0.862842315550003,
-0.101336213092694));
#22389=CARTESIAN_POINT('Ctrl Pts',(-3.25916182043291,0.863988641192523,
-0.104485716910859));
#22390=CARTESIAN_POINT('Ctrl Pts',(-3.27446023005863,0.864801422853929,
-0.106718816172519));
#22391=CARTESIAN_POINT('Ctrl Pts',(-3.28962546932607,0.865349158675545,
-0.108223707974235));
#22392=CARTESIAN_POINT('Ctrl Pts',(-3.30345932201092,0.865848807677636,
-0.109596482325133));
#22393=CARTESIAN_POINT('Ctrl Pts',(-3.31718287702708,0.866127684895366,
-0.110362691183646));
#22394=CARTESIAN_POINT('Ctrl Pts',(-3.33074870214876,0.866227388645556,
-0.110636624985929));
#22395=CARTESIAN_POINT('Ctrl Pts',(-3.33884111261622,0.866286864841397,
-0.110800034490998));
#22396=CARTESIAN_POINT('Ctrl Pts',(-3.34687301046511,0.86628237775275,-0.11078770631626));
#22397=CARTESIAN_POINT('Ctrl Pts',(-3.35484001959732,0.866221349813515,
-0.110620033431256));
#22398=CARTESIAN_POINT('Ctrl Pts',(-3.36947366066627,0.866109254930338,
-0.110312055270891));
#22399=CARTESIAN_POINT('Ctrl Pts',(-3.38389482814325,0.865807432300713,
-0.109482804411314));
#22400=CARTESIAN_POINT('Ctrl Pts',(-3.39813942762288,0.865348115847427,
-0.108220842827527));
#22401=CARTESIAN_POINT('Ctrl Pts',(-3.41318766118658,0.864862886250162,
-0.106887685465791));
#22402=CARTESIAN_POINT('Ctrl Pts',(-3.42803949559875,0.864201828823164,
-0.105071445112153));
#22403=CARTESIAN_POINT('Ctrl Pts',(-3.44275393648476,0.863384196034785,
-0.102825017488676));
#22404=CARTESIAN_POINT('Ctrl Pts',(-3.45532171030314,0.862685846431803,
-0.100906317723598));
#22405=CARTESIAN_POINT('Ctrl Pts',(-3.4677897761167,0.861872922343871,-0.0986728271482742));
#22406=CARTESIAN_POINT('Ctrl Pts',(-3.48019827523262,0.860947876601344,
-0.0961312848587167));
#22407=CARTESIAN_POINT('Ctrl Pts',(-3.49513963286312,0.8598340078623,-0.0930709556499571));
#22408=CARTESIAN_POINT('Ctrl Pts',(-3.50998931624428,0.858557840967348,
-0.089564715922621));
#22409=CARTESIAN_POINT('Ctrl Pts',(-3.52473645223634,0.857117620036816,
-0.0856077414369611));
#22410=CARTESIAN_POINT('Ctrl Pts',(-3.54127412363113,0.855502533521181,
-0.0811703277047876));
#22411=CARTESIAN_POINT('Ctrl Pts',(-3.55768510248944,0.853681303099851,
-0.0761665382465599));
#22412=CARTESIAN_POINT('Ctrl Pts',(-3.57395757994887,0.851634209192849,
-0.070542193961567));
#22413=CARTESIAN_POINT('Ctrl Pts',(-3.58761668013831,0.849915880754991,
-0.0658211253793454));
#22414=CARTESIAN_POINT('Ctrl Pts',(-3.60117829038003,0.848038110914512,
-0.060661995143698));
#22415=CARTESIAN_POINT('Ctrl Pts',(-3.6146298930802,0.84597971447189,-0.0550065973973076));
#22416=CARTESIAN_POINT('Ctrl Pts',(-3.62657049822057,0.844152534492555,
-0.0499864616628069));
#22417=CARTESIAN_POINT('Ctrl Pts',(-3.63843162632087,0.842181318652093,
-0.0445705906522641));
#22418=CARTESIAN_POINT('Ctrl Pts',(-3.65014896992634,0.8400553704926,-0.0387295960891255));
#22419=CARTESIAN_POINT('Ctrl Pts',(-3.66894272975055,0.836645505556185,
-0.0293610691729366));
#22420=CARTESIAN_POINT('Ctrl Pts',(-3.68735920610381,0.832838066824895,
-0.0189002172327613));
#22421=CARTESIAN_POINT('Ctrl Pts',(-3.70514280927609,0.828591806062877,
-0.00723371167200015));
#22422=CARTESIAN_POINT('Ctrl Pts',(-3.71362054925493,0.826567542797777,
-0.00167209406010711));
#22423=CARTESIAN_POINT('Ctrl Pts',(-3.72195672266957,0.824443138391217,
0.00416465907670791));
#22424=CARTESIAN_POINT('Ctrl Pts',(-3.73012282927105,0.822215961845034,
0.0102837763464823));
#22425=CARTESIAN_POINT('Ctrl Pts',(-3.74073718401333,0.819321064302234,
0.0182374419769606));
#22426=CARTESIAN_POINT('Ctrl Pts',(-3.75105335567548,0.816254009126217,
0.026664106817291));
#22427=CARTESIAN_POINT('Ctrl Pts',(-3.76096038332406,0.813036383310419,
0.0355044610904482));
#22428=CARTESIAN_POINT('Ctrl Pts',(-3.77048021789542,0.809944510897677,
0.0439993107282911));
#22429=CARTESIAN_POINT('Ctrl Pts',(-3.77962242626167,0.806713575795501,
0.0528762319652448));
#22430=CARTESIAN_POINT('Ctrl Pts',(-3.78831696314315,0.803374869806503,
0.062049251280213));
#22431=CARTESIAN_POINT('Ctrl Pts',(-3.79496379746781,0.800822482500531,
0.0690618777690747));
#22432=CARTESIAN_POINT('Ctrl Pts',(-3.80134959436443,0.798207357924017,
0.0762468734921084));
#22433=CARTESIAN_POINT('Ctrl Pts',(-3.80745376791091,0.795548593922769,
0.0835517675491962));
#22434=CARTESIAN_POINT('Ctrl Pts',(-3.82454823836735,0.788102841877238,
0.10400880316515));
#22435=CARTESIAN_POINT('Ctrl Pts',(-3.83946221950595,0.780306519377066,
0.125429023189158));
#22436=CARTESIAN_POINT('Ctrl Pts',(-3.85260231893967,0.772297204784702,
0.147434434176986));
#22437=CARTESIAN_POINT('Ctrl Pts',(-3.86512430791641,0.764664648460241,
0.168404710331158));
#22438=CARTESIAN_POINT('Ctrl Pts',(-3.87603724729861,0.756840228025687,
0.189902128795414));
#22439=CARTESIAN_POINT('Ctrl Pts',(-3.88566793707772,0.748948363478614,
0.211584848435892));
#22440=CARTESIAN_POINT('Ctrl Pts',(-3.89335476066421,0.742649399236893,
0.228891110455972));
#22441=CARTESIAN_POINT('Ctrl Pts',(-3.90022423734518,0.736307637874966,
0.246314956597437));
#22442=CARTESIAN_POINT('Ctrl Pts',(-3.90642254620822,0.729981049634948,
0.263697114929073));
#22443=CARTESIAN_POINT('Ctrl Pts',(-3.91059554935688,0.725721682567389,
0.275399629768361));
#22444=CARTESIAN_POINT('Ctrl Pts',(-3.91446234610801,0.721471283238569,
0.287077505947959));
#22445=CARTESIAN_POINT('Ctrl Pts',(-3.91807359617238,0.717231425397062,
0.298726419629196));
#22446=CARTESIAN_POINT('Ctrl Pts',(-3.92287656539946,0.711592406670298,
0.314219496248863));
#22447=CARTESIAN_POINT('Ctrl Pts',(-3.9272292236022,0.705971453373679,0.329662938507133));
#22448=CARTESIAN_POINT('Ctrl Pts',(-3.93123176207092,0.700356158170212,
0.34509083528223));
#22449=CARTESIAN_POINT('Ctrl Pts',(-3.93386883168704,0.696656524929363,
0.355255494071726));
#22450=CARTESIAN_POINT('Ctrl Pts',(-3.93635393272922,0.692958190829683,
0.365416583500196));
#22451=CARTESIAN_POINT('Ctrl Pts',(-3.93870841662801,0.689257829337623,
0.375583243143451));
#22452=CARTESIAN_POINT('Ctrl Pts',(-3.94382390749327,0.681218205273688,
0.397671928720016));
#22453=CARTESIAN_POINT('Ctrl Pts',(-3.94831885241916,0.673177794435633,
0.41976277594071));
#22454=CARTESIAN_POINT('Ctrl Pts',(-3.9523304703066,0.665170889075466,0.44176156761748));
#22455=CARTESIAN_POINT('Ctrl Pts',(-3.95613817456041,0.657570980894964,
0.462642143733336));
#22456=CARTESIAN_POINT('Ctrl Pts',(-3.95950945349948,0.650003104747759,
0.483434712561013));
#22457=CARTESIAN_POINT('Ctrl Pts',(-3.96254420999663,0.642468554647117,
0.504135718828276));
#22458=CARTESIAN_POINT('Ctrl Pts',(-3.96597393742826,0.633953389364699,
0.527530943164642));
#22459=CARTESIAN_POINT('Ctrl Pts',(-3.96897347355073,0.625481816767219,
0.55080639758349));
#22460=CARTESIAN_POINT('Ctrl Pts',(-3.97165158136693,0.617042978738954,
0.573991914512582));
#22461=CARTESIAN_POINT('Ctrl Pts',(-3.97412494043032,0.609249313227979,
0.595404834518768));
#22462=CARTESIAN_POINT('Ctrl Pts',(-3.97632347848357,0.601483217612124,
0.616742006860656));
#22463=CARTESIAN_POINT('Ctrl Pts',(-3.97831229220852,0.593724774977134,
0.638058152810425));
#22464=CARTESIAN_POINT('Ctrl Pts',(-3.97974379269629,0.588140433780633,
0.653401004150341));
#22465=CARTESIAN_POINT('Ctrl Pts',(-3.98106661594193,0.582557871569018,
0.668738967769455));
#22466=CARTESIAN_POINT('Ctrl Pts',(-3.98229809143707,0.576976592903405,
0.68407340487491));
#22467=CARTESIAN_POINT('Ctrl Pts',(-3.98480909968719,0.56559623102785,0.715340692153218));
#22468=CARTESIAN_POINT('Ctrl Pts',(-3.98694117105561,0.554226106519258,
0.746579852496963));
#22469=CARTESIAN_POINT('Ctrl Pts',(-3.9888095252893,0.542876129547436,0.777763657938374));
#22470=CARTESIAN_POINT('Ctrl Pts',(-3.99076772011234,0.530980384218651,
0.810446949616796));
#22471=CARTESIAN_POINT('Ctrl Pts',(-3.99243593368405,0.519106627018567,
0.843069829408114));
#22472=CARTESIAN_POINT('Ctrl Pts',(-3.99391540185511,0.507248820519574,
0.87564888500836));
#22473=CARTESIAN_POINT('Ctrl Pts',(-3.99551021095321,0.494466566694838,
0.91076783876156));
#22474=CARTESIAN_POINT('Ctrl Pts',(-3.99688550405414,0.481702741944058,
0.945836159050202));
#22475=CARTESIAN_POINT('Ctrl Pts',(-3.99813625458243,0.468931928776515,
0.980923679856098));
#22476=CARTESIAN_POINT('Ctrl Pts',(-3.99864819727412,0.463704727731907,
0.995285296693106));
#22477=CARTESIAN_POINT('Ctrl Pts',(-3.99913894233745,0.458476169216874,
1.00965064314946));
#22478=CARTESIAN_POINT('Ctrl Pts',(-3.99961373290197,0.453243799876032,
1.02402645976366));
#22479=CARTESIAN_POINT('',(-3.91965223258409,0.527570443506261,1.05372003673881));
#22480=CARTESIAN_POINT('Origin',(-3.91965223258409,0.452395033843389,1.02635842527276));
#22481=CARTESIAN_POINT('',(-2.95949419761707,0.524122950903392,1.06319194481893));
#22482=CARTESIAN_POINT('Ctrl Pts',(-3.91965223258409,0.527570443506261,
1.05372003673881));
#22483=CARTESIAN_POINT('Ctrl Pts',(-3.91557568799506,0.572495487342456,
0.930289493230857));
#22484=CARTESIAN_POINT('Ctrl Pts',(-3.90826705411741,0.639523973437174,
0.746130241225391));
#22485=CARTESIAN_POINT('Ctrl Pts',(-3.88392091137359,0.717116212326026,
0.532947316953341));
#22486=CARTESIAN_POINT('Ctrl Pts',(-3.85995110804723,0.761488798159762,
0.411034639332341));
#22487=CARTESIAN_POINT('Ctrl Pts',(-3.82635384144273,0.804962864100056,
0.2915906248295));
#22488=CARTESIAN_POINT('Ctrl Pts',(-3.77136677090444,0.846657118193748,
0.177036603186079));
#22489=CARTESIAN_POINT('Ctrl Pts',(-3.67711802975361,0.878650808373231,
0.089134661852922));
#22490=CARTESIAN_POINT('Ctrl Pts',(-3.58208993795251,0.897694758584722,
0.0368118386696318));
#22491=CARTESIAN_POINT('Ctrl Pts',(-3.46696656599506,0.910585447910795,
0.00139496082504257));
#22492=CARTESIAN_POINT('Ctrl Pts',(-3.3360951886178,0.916101759009581,-0.0137609793575587));
#22493=CARTESIAN_POINT('Ctrl Pts',(-3.22558881811219,0.910399758249608,
0.00190513897618206));
#22494=CARTESIAN_POINT('Ctrl Pts',(-3.15028872702707,0.894206994493787,
0.0463943917538627));
#22495=CARTESIAN_POINT('Ctrl Pts',(-3.11421209795167,0.879937567446779,
0.0855993203540729));
#22496=CARTESIAN_POINT('Ctrl Pts',(-3.09090069290084,0.867246541900823,
0.12046762647131));
#22497=CARTESIAN_POINT('Ctrl Pts',(-3.05105326213358,0.840475615777891,
0.194020141491951));
#22498=CARTESIAN_POINT('Ctrl Pts',(-2.99999967569416,0.770907793456571,
0.38515616244041));
#22499=CARTESIAN_POINT('Ctrl Pts',(-2.9782979876664,0.658827601540248,0.693093958898646));
#22500=CARTESIAN_POINT('Ctrl Pts',(-2.96698008492688,0.568998871692987,
0.939896365772286));
#22501=CARTESIAN_POINT('Ctrl Pts',(-2.9594941977123,0.524122950641471,1.06319194553855));
#22502=CARTESIAN_POINT('Origin',(-2.9594941977123,0.448947540978598,1.0358303340725));
#22503=CARTESIAN_POINT('Ctrl Pts',(-2.89005284851791,0.473859726879199,
1.19608230823957));
#22504=CARTESIAN_POINT('Ctrl Pts',(-2.89347901133131,0.474015979945485,
1.14661220793332));
#22505=CARTESIAN_POINT('Ctrl Pts',(-2.8967631553832,0.48293057760256,1.09714693603063));
#22506=CARTESIAN_POINT('Ctrl Pts',(-2.8997444856637,0.500000000116261,1.0507842073536));
#22507=CARTESIAN_POINT('Ctrl Pts',(-2.90496083257667,0.490269001123116,
1.19707182630597));
#22508=CARTESIAN_POINT('Ctrl Pts',(-2.90839510354824,0.490488270635738,
1.14949416876069));
#22509=CARTESIAN_POINT('Ctrl Pts',(-2.91169011394851,0.49911244823268,1.10190390404276));
#22510=CARTESIAN_POINT('Ctrl Pts',(-2.91467642669419,0.515552148620265,
1.05735131869985));
#22511=CARTESIAN_POINT('Ctrl Pts',(-2.92693299276352,0.499999999999999,
1.19853022935878));
#22512=CARTESIAN_POINT('Ctrl Pts',(-2.9304999693179,0.500173738497183,1.15205198095784));
#22513=CARTESIAN_POINT('Ctrl Pts',(-2.93391047394094,0.508550849038461,
1.10553353033146));
#22514=CARTESIAN_POINT('Ctrl Pts',(-2.9369928411141,0.524562029109686,1.06198558733789));
#22515=CARTESIAN_POINT('Ctrl Pts',(-2.94907641594456,0.499999999999999,
1.2));
#22516=CARTESIAN_POINT('Ctrl Pts',(-2.95278203038302,0.499999999999999,
1.15347630759795));
#22517=CARTESIAN_POINT('Ctrl Pts',(-2.95631131108945,0.508222479010737,
1.10687813316721));
#22518=CARTESIAN_POINT('Ctrl Pts',(-2.9594941977123,0.5241229508155,1.06319194506041));
#22519=CARTESIAN_POINT('Ctrl Pts',(-2.95949419767749,0.524122950641611,
1.06319194553817));
#22520=CARTESIAN_POINT('Ctrl Pts',(-2.95631131106372,0.508222478950789,
1.10687813350695));
#22521=CARTESIAN_POINT('Ctrl Pts',(-2.95278203036951,0.499999999999999,
1.15347630776754));
#22522=CARTESIAN_POINT('Ctrl Pts',(-2.94907641594456,0.499999999999999,
1.2));
#22523=CARTESIAN_POINT('Origin',(-3.91965223258409,0.452395033843409,1.0263584252727));
#22524=CARTESIAN_POINT('',(-3.99746275444911,0.445738635713984,1.04371397372222));
#22525=CARTESIAN_POINT('Origin',(-3.91965223258409,0.452395033843409,1.0263584252727));
#22526=CARTESIAN_POINT('Origin',(-3.91965223258409,0.452395033843409,1.0263584252727));
#22527=CARTESIAN_POINT('Ctrl Pts',(-3.99746275438256,0.445738635719676,
1.04371397370738));
#22528=CARTESIAN_POINT('Ctrl Pts',(-3.99706351813064,0.445109606322813,
1.0452626260641));
#22529=CARTESIAN_POINT('Ctrl Pts',(-3.99671788877829,0.44447641750283,1.04682338437936));
#22530=CARTESIAN_POINT('Ctrl Pts',(-3.99642658272506,0.443840379183309,
1.04839302148081));
#22531=CARTESIAN_POINT('Ctrl Pts',(-3.99755582933675,0.468280384206874,
1.0519421574563));
#22532=CARTESIAN_POINT('Ctrl Pts',(-3.9971768724252,0.467663343351554,1.05349202747387));
#22533=CARTESIAN_POINT('Ctrl Pts',(-3.99684651829552,0.46703688980806,1.05506776196706));
#22534=CARTESIAN_POINT('Ctrl Pts',(-3.99657534106215,0.466413555729912,
1.05663619619577));
#22535=CARTESIAN_POINT('Ctrl Pts',(-3.97806581626837,0.508977365274313,
1.06180057527797));
#22536=CARTESIAN_POINT('Ctrl Pts',(-3.97759566678914,0.508247059602534,
1.06376320056323));
#22537=CARTESIAN_POINT('Ctrl Pts',(-3.97719426482472,0.507513520656082,
1.06573512393595));
#22538=CARTESIAN_POINT('Ctrl Pts',(-3.97685956385479,0.50677514383455,1.06772027127607));
#22539=CARTESIAN_POINT('Ctrl Pts',(-3.93715733927913,0.526140389499051,
1.05764907783222));
#22540=CARTESIAN_POINT('Ctrl Pts',(-3.93645817327013,0.525126591517723,
1.06043493280982));
#22541=CARTESIAN_POINT('Ctrl Pts',(-3.93585500062643,0.524105540900254,
1.0632393122251));
#22542=CARTESIAN_POINT('Ctrl Pts',(-3.93534760874183,0.523078681693311,
1.06606105089346));
#22543=CARTESIAN_POINT('Ctrl Pts',(-3.91965223258409,0.527570443506282,
1.05372003673876));
#22544=CARTESIAN_POINT('Ctrl Pts',(-3.91885525761101,0.526429247151133,
1.05685544795569));
#22545=CARTESIAN_POINT('Ctrl Pts',(-3.91816549099621,0.525279290574345,
1.06001492768377));
#22546=CARTESIAN_POINT('Ctrl Pts',(-3.91758436243191,0.524122951685363,
1.06319194267048));
#22547=CARTESIAN_POINT('Origin',(-4.05559523088995,0.440984362651786,1.05744795078647));
#22548=CARTESIAN_POINT('Origin',(-4.03591301597994,0.517624494217011,1.08104630782635));
#22549=CARTESIAN_POINT('Ctrl Pts',(-3.99500090812059,0.125168749047044,
0.930078956913999));
#22550=CARTESIAN_POINT('Ctrl Pts',(-3.99593963459395,0.232006196698264,
0.968035837491526));
#22551=CARTESIAN_POINT('Ctrl Pts',(-3.99674494883676,0.33885382942011,1.00593844604213));
#22552=CARTESIAN_POINT('Ctrl Pts',(-3.99746275438256,0.445738635719677,
1.04371397370738));
#22553=CARTESIAN_POINT('Ctrl Pts',(-3.99824520675537,0.128463087592629,
0.921420039511872));
#22554=CARTESIAN_POINT('Ctrl Pts',(-3.99857533133843,0.235036780014703,
0.960065081373451));
#22555=CARTESIAN_POINT('Ctrl Pts',(-3.99885884426554,0.341611566532603,
0.998688309789087));
#22556=CARTESIAN_POINT('Ctrl Pts',(-3.99910791850814,0.448191320810768,
1.0372788540661));
#22557=CARTESIAN_POINT('Ctrl Pts',(-3.99976439851731,0.131971946808211,
0.91219976288192));
#22558=CARTESIAN_POINT('Ctrl Pts',(-3.99978611058741,0.238221660879987,
0.95169039150062));
#22559=CARTESIAN_POINT('Ctrl Pts',(-3.99981055015748,0.344480567483035,
0.991147371513851));
#22560=CARTESIAN_POINT('Ctrl Pts',(-3.99983334587227,0.450722471820515,
1.03063914975585));
#22561=CARTESIAN_POINT('Ctrl Pts',(-3.99945760881125,0.135462337836371,
0.903030354983464));
#22562=CARTESIAN_POINT('Ctrl Pts',(-3.99950970007112,0.241391193737631,
0.943357929054413));
#22563=CARTESIAN_POINT('Ctrl Pts',(-3.99956010118928,0.347337150066848,
0.983640596922404));
#22564=CARTESIAN_POINT('Ctrl Pts',(-3.99961373290197,0.453243799876052,
1.02402645976362));
#22565=CARTESIAN_POINT('Ctrl Pts',(-3.99961373290197,0.453243799876052,
1.02402645976362));
#22566=CARTESIAN_POINT('Ctrl Pts',(-3.99956010118928,0.347337150066848,
0.983640596922404));
#22567=CARTESIAN_POINT('Ctrl Pts',(-3.99950970007112,0.241391193737631,
0.943357929054413));
#22568=CARTESIAN_POINT('Ctrl Pts',(-3.99945760881125,0.135462337836371,
0.903030354983464));
#22569=CARTESIAN_POINT('',(-3.99500090813004,0.125168749022039,0.930078956989209));
#22570=CARTESIAN_POINT('Origin',(-3.91949669889834,0.134607090093723,0.905380128844431));
#22571=CARTESIAN_POINT('Ctrl Pts',(-3.99500090812059,0.125168749047044,
0.930078956913999));
#22572=CARTESIAN_POINT('Ctrl Pts',(-3.99593963459395,0.232006196698264,
0.968035837491526));
#22573=CARTESIAN_POINT('Ctrl Pts',(-3.99674494883676,0.33885382942011,1.00593844604213));
#22574=CARTESIAN_POINT('Ctrl Pts',(-3.99746275438256,0.445738635719677,
1.04371397370738));
#22575=CARTESIAN_POINT('Ctrl Pts',(-2.87936339380758,0.054276641292682,
0.892181871006899));
#22576=CARTESIAN_POINT('Ctrl Pts',(-2.87936339380758,0.618092213764237,
1.0973939570023));
#22577=CARTESIAN_POINT('Ctrl Pts',(-2.88050601962387,0.061089278956966,
0.873464302857353));
#22578=CARTESIAN_POINT('Ctrl Pts',(-2.88050601962387,0.624904851428521,
1.07867638885275));
#22579=CARTESIAN_POINT('Ctrl Pts',(-2.88410012960011,0.0831761921549222,
0.812781007580514));
#22580=CARTESIAN_POINT('Ctrl Pts',(-2.88410012960011,0.646991764626477,
1.01799309357591));
#22581=CARTESIAN_POINT('Ctrl Pts',(-2.88965455295869,0.120639229722751,
0.709852157798725));
#22582=CARTESIAN_POINT('Ctrl Pts',(-2.88965455295869,0.684454802194306,
0.915064243794126));
#22583=CARTESIAN_POINT('Ctrl Pts',(-2.89676647174981,0.173526397310949,
0.564545859071238));
#22584=CARTESIAN_POINT('Ctrl Pts',(-2.89676647174981,0.737341969782504,
0.769757945066639));
#22585=CARTESIAN_POINT('Ctrl Pts',(-2.90717911786707,0.241012720183549,
0.379128710856747));
#22586=CARTESIAN_POINT('Ctrl Pts',(-2.90717911786707,0.804828292655104,
0.584340796852148));
#22587=CARTESIAN_POINT('Ctrl Pts',(-2.92780415844476,0.312514210565547,
0.182679980574853));
#22588=CARTESIAN_POINT('Ctrl Pts',(-2.92780415844476,0.876329783037102,
0.387892066570254));
#22589=CARTESIAN_POINT('Ctrl Pts',(-2.96639254265869,0.374982215648805,
0.0110505471702249));
#22590=CARTESIAN_POINT('Ctrl Pts',(-2.96639254265869,0.93879778812036,0.216262633165626));
#22591=CARTESIAN_POINT('Ctrl Pts',(-3.03063129752067,0.423994474883956,
-0.123609528354807));
#22592=CARTESIAN_POINT('Ctrl Pts',(-3.03063129752067,0.987810047355511,
0.0816025576405938));
#22593=CARTESIAN_POINT('Ctrl Pts',(-3.12452733970658,0.456428987719491,
-0.212722619981451));
#22594=CARTESIAN_POINT('Ctrl Pts',(-3.12452733970658,1.02024456019105,-0.00751053398605017));
#22595=CARTESIAN_POINT('Ctrl Pts',(-3.24511001026157,0.472026186037003,
-0.255575570165571));
#22596=CARTESIAN_POINT('Ctrl Pts',(-3.24511001026157,1.03584175850856,-0.0503634841701701));
#22597=CARTESIAN_POINT('Ctrl Pts',(-3.38164698943802,0.473698270059231,
-0.260169583260074));
#22598=CARTESIAN_POINT('Ctrl Pts',(-3.38164698943802,1.03751384253079,-0.0549574972646732));
#22599=CARTESIAN_POINT('Ctrl Pts',(-3.52045328348989,0.465105650196581,
-0.236561554213485));
#22600=CARTESIAN_POINT('Ctrl Pts',(-3.52045328348989,1.02892122266814,-0.0313494682180842));
#22601=CARTESIAN_POINT('Ctrl Pts',(-3.64881642260079,0.448607387242662,
-0.191232949287367));
#22602=CARTESIAN_POINT('Ctrl Pts',(-3.64881642260079,1.01242295971422,0.0139791367080338));
#22603=CARTESIAN_POINT('Ctrl Pts',(-3.75872318140663,0.42348833261052,-0.122218913887511));
#22604=CARTESIAN_POINT('Ctrl Pts',(-3.75872318140663,0.987303905082075,
0.0829931721078898));
#22605=CARTESIAN_POINT('Ctrl Pts',(-3.84598208672296,0.387862727674243,
-0.0243383687706796));
#22606=CARTESIAN_POINT('Ctrl Pts',(-3.84598208672296,0.951678300145798,
0.180873717224721));
#22607=CARTESIAN_POINT('Ctrl Pts',(-3.9098657241983,0.340085651878983,0.10692806814437));
#22608=CARTESIAN_POINT('Ctrl Pts',(-3.9098657241983,0.903901224350538,0.312140154139771));
#22609=CARTESIAN_POINT('Ctrl Pts',(-3.9525920016999,0.280544576017308,0.270515829604357));
#22610=CARTESIAN_POINT('Ctrl Pts',(-3.9525920016999,0.844360148488863,0.475727915599758));
#22611=CARTESIAN_POINT('Ctrl Pts',(-3.97841403016126,0.21121967143493,0.460984439550287));
#22612=CARTESIAN_POINT('Ctrl Pts',(-3.97841403016126,0.775035243906485,
0.666196525545688));
#22613=CARTESIAN_POINT('Ctrl Pts',(-3.98977740850458,0.150154761706452,
0.628758900150314));
#22614=CARTESIAN_POINT('Ctrl Pts',(-3.98977740850458,0.713970334178007,
0.833970986145715));
#22615=CARTESIAN_POINT('Ctrl Pts',(-3.99545186687387,0.102617065619347,
0.759367646722532));
#22616=CARTESIAN_POINT('Ctrl Pts',(-3.99545186687387,0.666432638090902,
0.964579732717933));
#22617=CARTESIAN_POINT('Ctrl Pts',(-3.99855414331415,0.0704990924696529,
0.847611052709967));
#22618=CARTESIAN_POINT('Ctrl Pts',(-3.99855414331415,0.634314664941208,
1.05282313870537));
#22619=CARTESIAN_POINT('Ctrl Pts',(-3.99999413894399,0.054342424295042,
0.892001133693331));
#22620=CARTESIAN_POINT('Ctrl Pts',(-3.99999413894399,0.618157996766597,
1.09721321968873));
#22621=CARTESIAN_POINT('Ctrl Pts',(-4.,0.0542766412926824,0.892181871006898));
#22622=CARTESIAN_POINT('Ctrl Pts',(-4.,0.618092213764237,1.0973939570023));
#22623=CARTESIAN_POINT('',(-2.87936339380758,0.0542766412926824,0.892181871006898));
#22624=CARTESIAN_POINT('Ctrl Pts',(-2.87936339380758,0.510402750471661,
1.0581981978197));
#22625=CARTESIAN_POINT('Ctrl Pts',(-2.87936339380758,0.38345364991127,1.01199250394885));
#22626=CARTESIAN_POINT('Ctrl Pts',(-2.87936339380758,0.25645519700216,0.965768847292079));
#22627=CARTESIAN_POINT('Ctrl Pts',(-2.87936339380758,0.129452050955553,
0.919543482472951));
#22628=CARTESIAN_POINT('Ctrl Pts',(-2.88380565711847,0.507160352260398,
1.06851837583814));
#22629=CARTESIAN_POINT('Ctrl Pts',(-2.885256581924,0.379732217321614,1.02359703230995));
#22630=CARTESIAN_POINT('Ctrl Pts',(-2.88661730605277,0.252436541519274,
0.978175521115242));
#22631=CARTESIAN_POINT('Ctrl Pts',(-2.88800949912464,0.125204871749137,
0.932598552100246));
#22632=CARTESIAN_POINT('Ctrl Pts',(-2.88583635958945,0.503581269771104,
1.07976272406583));
#22633=CARTESIAN_POINT('Ctrl Pts',(-2.88803975294752,0.375510613992429,
1.03657431850542));
#22634=CARTESIAN_POINT('Ctrl Pts',(-2.8901570753878,0.247726768638573,0.992479117588928));
#22635=CARTESIAN_POINT('Ctrl Pts',(-2.89233651283672,0.120040512706022,
0.948170442679049));
#22636=CARTESIAN_POINT('Ctrl Pts',(-2.8852657140673,0.5,1.09088035845137));
#22637=CARTESIAN_POINT('Ctrl Pts',(-2.88739518236194,0.371284826357953,
1.04939286925411));
#22638=CARTESIAN_POINT('Ctrl Pts',(-2.88948025018409,0.243010859025609,
1.00659623192935));
#22639=CARTESIAN_POINT('Ctrl Pts',(-2.89158569656657,0.114864540034388,
0.963528635709792));
#22640=CARTESIAN_POINT('Ctrl Pts',(-2.803641505311,0.08,1.2));
#22641=CARTESIAN_POINT('Ctrl Pts',(-2.803641505311,0.584,1.2));
#22642=CARTESIAN_POINT('Ctrl Pts',(-2.82677300877682,0.08,1.2));
#22643=CARTESIAN_POINT('Ctrl Pts',(-2.82677300877682,0.584,1.2));
#22644=CARTESIAN_POINT('Ctrl Pts',(-2.86687236848073,0.08,1.18130984727688));
#22645=CARTESIAN_POINT('Ctrl Pts',(-2.86687236848073,0.584,1.18130984727688));
#22646=CARTESIAN_POINT('Ctrl Pts',(-2.88261462067416,0.08,1.14154581001999));
#22647=CARTESIAN_POINT('Ctrl Pts',(-2.88261462067416,0.584,1.14154581001999));
#22648=CARTESIAN_POINT('Ctrl Pts',(-2.88353005387198,0.08,1.12422135153951));
#22649=CARTESIAN_POINT('Ctrl Pts',(-2.88353005387198,0.584,1.12422135153951));
#22650=CARTESIAN_POINT('',(-2.803641505311,0.5,1.2));
#22651=CARTESIAN_POINT('Ctrl Pts',(-3.9106833422892,0.0384897740707112,
0.939615427909197));
#22652=CARTESIAN_POINT('Ctrl Pts',(-3.91354391573668,0.0199991968201913,
1.00079349366622));
#22653=CARTESIAN_POINT('Ctrl Pts',(-3.9158360335454,0.00804296821746633,
1.06397598649794));
#22654=CARTESIAN_POINT('Ctrl Pts',(-3.91781846660453,0.00290707172437443,
1.12772087043234));
#22655=CARTESIAN_POINT('Ctrl Pts',(-3.93437185463721,0.0388201352419867,
0.938499550671921));
#22656=CARTESIAN_POINT('Ctrl Pts',(-3.93732958055613,0.0201980578537388,
0.999813489629965));
#22657=CARTESIAN_POINT('Ctrl Pts',(-3.93967836210679,0.00816932330334512,
1.06306801873905));
#22658=CARTESIAN_POINT('Ctrl Pts',(-3.94170600662187,0.00296563685502545,
1.12691026059145));
#22659=CARTESIAN_POINT('Ctrl Pts',(-3.97540039704606,0.0582587635086386,
0.942269104078657));
#22660=CARTESIAN_POINT('Ctrl Pts',(-3.97851429576965,0.0399886969010512,
1.00247500534244));
#22661=CARTESIAN_POINT('Ctrl Pts',(-3.98096563012735,0.0281607199544487,
1.06457282534426));
#22662=CARTESIAN_POINT('Ctrl Pts',(-3.98306565367973,0.0230377862102752,
1.12711565157154));
#22663=CARTESIAN_POINT('Ctrl Pts',(-3.99034065233881,0.0980581224574643,
0.953531437079163));
#22664=CARTESIAN_POINT('Ctrl Pts',(-3.99333584061565,0.0807856567863764,
1.01108170025839));
#22665=CARTESIAN_POINT('Ctrl Pts',(-3.9957069693143,0.0696117321811971,
1.07033813817931));
#22666=CARTESIAN_POINT('Ctrl Pts',(-3.99774875287515,0.0647997910680151,
1.12997927823579));
#22667=CARTESIAN_POINT('Ctrl Pts',(-3.990599354584,0.115088570413461,0.958665497906023));
#22668=CARTESIAN_POINT('Ctrl Pts',(-3.9934922166161,0.0982419908213599,
1.01503404648247));
#22669=CARTESIAN_POINT('Ctrl Pts',(-3.99580030401545,0.087348807066054,
1.07303953608064));
#22670=CARTESIAN_POINT('Ctrl Pts',(-3.99779298688,0.0826695349261019,1.13141756172706));
#22671=CARTESIAN_POINT('',(-3.99059905039462,0.115068728348614,0.9586595164214));
#22672=CARTESIAN_POINT('Ctrl Pts',(-3.99749553673965,0.0833869626360487,
1.12277470481743));
#22673=CARTESIAN_POINT('Ctrl Pts',(-3.99557092677476,0.088417954777819,
1.0673144474751));
#22674=CARTESIAN_POINT('Ctrl Pts',(-3.99334924695252,0.0990531491906679,
1.01224727331911));
#22675=CARTESIAN_POINT('Ctrl Pts',(-3.99059905039179,0.115068728358824,
0.958659516390688));
#22676=CARTESIAN_POINT('Origin',(-3.91070419800688,0.115068728358824,0.96275982886584));
#22677=CARTESIAN_POINT('Ctrl Pts',(-3.99059905039179,0.115068728358825,
0.958659516390683));
#22678=CARTESIAN_POINT('Ctrl Pts',(-3.99022032406425,0.117088541529883,
0.951280009531972));
#22679=CARTESIAN_POINT('Ctrl Pts',(-3.99095351851113,0.11955866968438,0.943986539572236));
#22680=CARTESIAN_POINT('Ctrl Pts',(-3.99276651177431,0.122341921457849,
0.937078276746861));
#22681=CARTESIAN_POINT('Ctrl Pts',(-3.99024788717857,0.0923702555515019,
0.951817078587972));
#22682=CARTESIAN_POINT('Ctrl Pts',(-3.98978566864749,0.0945716870691454,
0.944022370054385));
#22683=CARTESIAN_POINT('Ctrl Pts',(-3.99058029988189,0.0971825638221607,
0.93620230647329));
#22684=CARTESIAN_POINT('Ctrl Pts',(-3.99256871721073,0.0999892111837481,
0.928891350782428));
#22685=CARTESIAN_POINT('Ctrl Pts',(-3.96997099994117,0.0530616659229667,
0.940976960505986));
#22686=CARTESIAN_POINT('Ctrl Pts',(-3.96936836234513,0.0561827488203104,
0.930609204971929));
#22687=CARTESIAN_POINT('Ctrl Pts',(-3.97037966405284,0.0595786334866178,
0.920227936342186));
#22688=CARTESIAN_POINT('Ctrl Pts',(-3.97292637392248,0.0630513948986112,
0.910362103819981));
#22689=CARTESIAN_POINT('Ctrl Pts',(-3.92846526015161,0.0387425083350586,
0.938779222925522));
#22690=CARTESIAN_POINT('Ctrl Pts',(-3.92775891147314,0.0431208469974308,
0.924351545690715));
#22691=CARTESIAN_POINT('Ctrl Pts',(-3.9290879339547,0.047896842751599,0.909937955493114));
#22692=CARTESIAN_POINT('Ctrl Pts',(-3.9323846422143,0.0528332298852771,
0.896147611255728));
#22693=CARTESIAN_POINT('Ctrl Pts',(-3.91070419800688,0.0384900677109053,
0.939614446316161));
#22694=CARTESIAN_POINT('Ctrl Pts',(-3.90995323778991,0.043344115284559,
0.923554376403128));
#22695=CARTESIAN_POINT('Ctrl Pts',(-3.91141850629553,0.0486938803101099,
0.90752038074473));
#22696=CARTESIAN_POINT('Ctrl Pts',(-3.91503635643999,0.0542766412926799,
0.892181871006906));
#22697=CARTESIAN_POINT('',(-3.99276651177429,0.122341921455471,0.93707827674599));
#22698=CARTESIAN_POINT('Origin',(-3.91503635643999,0.129452050955553,0.919543482472958));
#22699=CARTESIAN_POINT('Ctrl Pts',(-3.99059905039179,0.115068728358825,
0.958659516390683));
#22700=CARTESIAN_POINT('Ctrl Pts',(-3.99022032406425,0.117088541529883,
0.951280009531972));
#22701=CARTESIAN_POINT('Ctrl Pts',(-3.99095351851113,0.11955866968438,0.943986539572236));
#22702=CARTESIAN_POINT('Ctrl Pts',(-3.99276651177431,0.122341921457849,
0.937078276746861));
#22703=CARTESIAN_POINT('Ctrl Pts',(-3.91949669889834,0.0594316804308502,
0.878018517378377));
#22704=CARTESIAN_POINT('Ctrl Pts',(-3.91776450002014,0.0577396751765171,
0.882667263608256));
#22705=CARTESIAN_POINT('Ctrl Pts',(-3.91627531395221,0.0560185533163472,
0.887396007055203));
#22706=CARTESIAN_POINT('Ctrl Pts',(-3.91503635643999,0.0542766412926799,
0.892181871006905));
#22707=CARTESIAN_POINT('Ctrl Pts',(-3.94201201831921,0.0567353225932654,
0.885426699651911));
#22708=CARTESIAN_POINT('Ctrl Pts',(-3.9405226858886,0.0552989731010419,
0.889375045120937));
#22709=CARTESIAN_POINT('Ctrl Pts',(-3.93923778894123,0.053832019954493,
0.893401502356153));
#22710=CARTESIAN_POINT('Ctrl Pts',(-3.93816740413907,0.052352092749476,
0.897469524672002));
#22711=CARTESIAN_POINT('Ctrl Pts',(-3.98099331223824,0.070815773798773,
0.905076632451692));
#22712=CARTESIAN_POINT('Ctrl Pts',(-3.97992327128341,0.069788483816893,
0.907811358142667));
#22713=CARTESIAN_POINT('Ctrl Pts',(-3.97899701572105,0.068744459577118,
0.91059438223949));
#22714=CARTESIAN_POINT('Ctrl Pts',(-3.97821832116159,0.0676852936406248,
0.913418676649671));
#22715=CARTESIAN_POINT('Ctrl Pts',(-3.99491190730368,0.108366920859318,
0.923930428412372));
#22716=CARTESIAN_POINT('Ctrl Pts',(-3.99402530924208,0.107450746899103,
0.926226086767676));
#22717=CARTESIAN_POINT('Ctrl Pts',(-3.99325856149151,0.106518326821552,
0.928569719091837));
#22718=CARTESIAN_POINT('Ctrl Pts',(-3.99261816585162,0.105577388752273,
0.930938082273536));
#22719=CARTESIAN_POINT('Ctrl Pts',(-3.99500090812059,0.125168749047044,
0.930078956913999));
#22720=CARTESIAN_POINT('Ctrl Pts',(-3.99413338741396,0.124238863836765,
0.932375620181965));
#22721=CARTESIAN_POINT('Ctrl Pts',(-3.99338738371022,0.123295065052931,
0.934712494920036));
#22722=CARTESIAN_POINT('Ctrl Pts',(-3.99276651177431,0.122341921457849,
0.937078276746861));
#22723=CARTESIAN_POINT('Origin',(-3.91949669889834,0.134607090093723,0.905380128844431));
#22724=CARTESIAN_POINT('Origin',(-4.0510872574969,0.118364537007352,0.949600376125361));
#22725=CARTESIAN_POINT('Origin',(-3.91949669889834,0.134607090093723,0.905380128844431));
#22726=CARTESIAN_POINT('Ctrl Pts',(-3.99499168547955,0.124132806141263,
0.929711262728432));
#22727=CARTESIAN_POINT('Ctrl Pts',(-3.99594631188109,0.231310970463683,
0.9677529322264));
#22728=CARTESIAN_POINT('Ctrl Pts',(-3.99676075730698,0.338517926331372,
1.00575284837914));
#22729=CARTESIAN_POINT('Ctrl Pts',(-3.99748245955517,0.445763956511613,
1.04363554723628));
#22730=CARTESIAN_POINT('Ctrl Pts',(-3.9915949893774,0.121141354506694,0.938941135546907));
#22731=CARTESIAN_POINT('Ctrl Pts',(-3.99320655831758,0.22857262587258,0.976182588452333));
#22732=CARTESIAN_POINT('Ctrl Pts',(-3.99457441210398,0.336045551741593,
1.01337043101945));
#22733=CARTESIAN_POINT('Ctrl Pts',(-3.99578832520602,0.443592156028746,
1.05036245459742));
#22734=CARTESIAN_POINT('Ctrl Pts',(-3.99009222817804,0.117914157270493,
0.948787406604446));
#22735=CARTESIAN_POINT('Ctrl Pts',(-3.9920041082913,0.225667811748472,0.985047957459691));
#22736=CARTESIAN_POINT('Ctrl Pts',(-3.99362608533509,0.333454367731145,
1.02129852328768));
#22737=CARTESIAN_POINT('Ctrl Pts',(-3.99506362287769,0.441337300197856,
1.05730597317919));
#22738=CARTESIAN_POINT('Ctrl Pts',(-3.99059262862431,0.114685780139278,
0.958534409222154));
#22739=CARTESIAN_POINT('Ctrl Pts',(-3.9924053082979,0.2227624802018,0.993842518267836));
#22740=CARTESIAN_POINT('Ctrl Pts',(-3.99395808870925,0.330862808266828,
1.02917430286131));
#22741=CARTESIAN_POINT('Ctrl Pts',(-3.99533497979657,0.439082237595944,
1.06421098217699));
#22742=CARTESIAN_POINT('Ctrl Pts',(-3.99059905040313,0.115068728317981,
0.958659516513544));
#22743=CARTESIAN_POINT('Ctrl Pts',(-3.9924069847619,0.22289907004185,0.993887178660277));
#22744=CARTESIAN_POINT('Ctrl Pts',(-3.99395630241674,0.330753044397502,
1.02913803372068));
#22745=CARTESIAN_POINT('Ctrl Pts',(-3.99533043998868,0.438725473099098,
1.06409547635602));
#22746=CARTESIAN_POINT('Ctrl Pts',(-2.87936339380758,-3.,1.2));
#22747=CARTESIAN_POINT('Ctrl Pts',(-2.87936339380758,4.2,1.2));
#22748=CARTESIAN_POINT('Ctrl Pts',(-2.88050601962387,-3.,1.18008118002045));
#22749=CARTESIAN_POINT('Ctrl Pts',(-2.88050601962387,4.2,1.18008118002045));
#22750=CARTESIAN_POINT('Ctrl Pts',(-2.88410012960011,-3.,1.11550336602625));
#22751=CARTESIAN_POINT('Ctrl Pts',(-2.88410012960011,4.2,1.11550336602625));
#22752=CARTESIAN_POINT('Ctrl Pts',(-2.88965455295869,-3.,1.00596877194195));
#22753=CARTESIAN_POINT('Ctrl Pts',(-2.88965455295869,4.2,1.00596877194195));
#22754=CARTESIAN_POINT('Ctrl Pts',(-2.89676647174981,-3.,0.851337038635417));
#22755=CARTESIAN_POINT('Ctrl Pts',(-2.89676647174981,4.2,0.851337038635417));
#22756=CARTESIAN_POINT('Ctrl Pts',(-2.90717911786707,-3.,0.654020230869684));
#22757=CARTESIAN_POINT('Ctrl Pts',(-2.90717911786707,4.2,0.654020230869684));
#22758=CARTESIAN_POINT('Ctrl Pts',(-2.92780415844476,-3.,0.444963858672577));
#22759=CARTESIAN_POINT('Ctrl Pts',(-2.92780415844476,4.2,0.444963858672577));
#22760=CARTESIAN_POINT('Ctrl Pts',(-2.96639254265869,-3.,0.262319630540737));
#22761=CARTESIAN_POINT('Ctrl Pts',(-2.96639254265869,4.2,0.262319630540737));
#22762=CARTESIAN_POINT('Ctrl Pts',(-3.03063129752067,-3.,0.11901737132707));
#22763=CARTESIAN_POINT('Ctrl Pts',(-3.03063129752067,4.2,0.11901737132707));
#22764=CARTESIAN_POINT('Ctrl Pts',(-3.12452733970658,-3.,0.0241851999813871));
#22765=CARTESIAN_POINT('Ctrl Pts',(-3.12452733970658,4.2,0.0241851999813871));
#22766=CARTESIAN_POINT('Ctrl Pts',(-3.24511001026157,-3.,-0.0214179570895714));
#22767=CARTESIAN_POINT('Ctrl Pts',(-3.24511001026157,4.2,-0.0214179570895714));
#22768=CARTESIAN_POINT('Ctrl Pts',(-3.38164698943802,-3.,-0.0263068037112043));
#22769=CARTESIAN_POINT('Ctrl Pts',(-3.38164698943802,4.2,-0.0263068037112043));
#22770=CARTESIAN_POINT('Ctrl Pts',(-3.52045328348989,-3.,-0.00118366394785932));
#22771=CARTESIAN_POINT('Ctrl Pts',(-3.52045328348989,4.2,-0.00118366394785932));
#22772=CARTESIAN_POINT('Ctrl Pts',(-3.64881642260079,-3.,0.0470540298718583));
#22773=CARTESIAN_POINT('Ctrl Pts',(-3.64881642260079,4.2,0.0470540298718583));
#22774=CARTESIAN_POINT('Ctrl Pts',(-3.75872318140663,-3.,0.120497232333251));
#22775=CARTESIAN_POINT('Ctrl Pts',(-3.75872318140663,4.2,0.120497232333251));
#22776=CARTESIAN_POINT('Ctrl Pts',(-3.84598208672296,-3.,0.224659532804408));
#22777=CARTESIAN_POINT('Ctrl Pts',(-3.84598208672296,4.2,0.224659532804408));
#22778=CARTESIAN_POINT('Ctrl Pts',(-3.9098657241983,-3.,0.364350357241515));
#22779=CARTESIAN_POINT('Ctrl Pts',(-3.9098657241983,4.2,0.364350357241515));
#22780=CARTESIAN_POINT('Ctrl Pts',(-3.9525920016999,-3.,0.538436816836325));
#22781=CARTESIAN_POINT('Ctrl Pts',(-3.9525920016999,4.2,0.538436816836325));
#22782=CARTESIAN_POINT('Ctrl Pts',(-3.97841403016126,-3.,0.741129277895169));
#22783=CARTESIAN_POINT('Ctrl Pts',(-3.97841403016126,4.2,0.741129277895169));
#22784=CARTESIAN_POINT('Ctrl Pts',(-3.98977740850458,-3.,0.919671129654853));
#22785=CARTESIAN_POINT('Ctrl Pts',(-3.98977740850458,4.2,0.919671129654853));
#22786=CARTESIAN_POINT('Ctrl Pts',(-3.99545186687387,-3.,1.05866205464795));
#22787=CARTESIAN_POINT('Ctrl Pts',(-3.99545186687387,4.2,1.05866205464795));
#22788=CARTESIAN_POINT('Ctrl Pts',(-3.99855414331415,-3.,1.15256872586734));
#22789=CARTESIAN_POINT('Ctrl Pts',(-3.99855414331415,4.2,1.15256872586734));
#22790=CARTESIAN_POINT('Ctrl Pts',(-3.99999413894399,-3.,1.19980766336825));
#22791=CARTESIAN_POINT('Ctrl Pts',(-3.99999413894399,4.2,1.19980766336825));
#22792=CARTESIAN_POINT('Ctrl Pts',(-4.,-3.,1.2));
#22793=CARTESIAN_POINT('Ctrl Pts',(-4.,4.2,1.2));
#22794=CARTESIAN_POINT('Origin',(-3.2,0.9,1.2));
#22795=CARTESIAN_POINT('',(-4.5,0.524122951685637,1.06319194266973));
#22796=CARTESIAN_POINT('Origin',(4.1,0.,1.2));
#22797=CARTESIAN_POINT('Origin',(3.2,0.9,1.2));
#22798=CARTESIAN_POINT('',(-4.5,0.524122951685637,1.06319194266973));
#22799=CARTESIAN_POINT('Ctrl Pts',(4.08617023400024,-0.552060840994624,
11.9163435012344));
#22800=CARTESIAN_POINT('Ctrl Pts',(4.08617023400024,1.61522066995007,11.9163435012344));
#22801=CARTESIAN_POINT('Ctrl Pts',(4.10576511646638,-0.552060840994624,
11.8970344456328));
#22802=CARTESIAN_POINT('Ctrl Pts',(4.10576511646638,1.61522066995007,11.8970344456328));
#22803=CARTESIAN_POINT('Ctrl Pts',(4.15149421914094,-0.552060840994624,
11.8511956487512));
#22804=CARTESIAN_POINT('Ctrl Pts',(4.15149421914094,1.61522066995007,11.8511956487512));
#22805=CARTESIAN_POINT('Ctrl Pts',(4.22408937937455,-0.552060840994624,
11.7763607682953));
#22806=CARTESIAN_POINT('Ctrl Pts',(4.22408937937455,1.61522066995007,11.7763607682953));
#22807=CARTESIAN_POINT('Ctrl Pts',(4.3260071847331,-0.552060840994624,11.6707401393954));
#22808=CARTESIAN_POINT('Ctrl Pts',(4.3260071847331,1.61522066995007,11.6707401393954));
#22809=CARTESIAN_POINT('Ctrl Pts',(4.46255574628753,-0.552060840994624,
11.5373242211525));
#22810=CARTESIAN_POINT('Ctrl Pts',(4.46255574628753,1.61522066995007,11.5373242211525));
#22811=CARTESIAN_POINT('Ctrl Pts',(4.61532593596939,-0.552060840994624,
11.4029224160728));
#22812=CARTESIAN_POINT('Ctrl Pts',(4.61532593596939,1.61522066995007,11.4029224160728));
#22813=CARTESIAN_POINT('Ctrl Pts',(4.77596612414944,-0.552060840994624,
11.2768795166233));
#22814=CARTESIAN_POINT('Ctrl Pts',(4.77596612414944,1.61522066995007,11.2768795166233));
#22815=CARTESIAN_POINT('Ctrl Pts',(4.94211773226968,-0.552060840994624,
11.1598106424589));
#22816=CARTESIAN_POINT('Ctrl Pts',(4.94211773226968,1.61522066995007,11.1598106424589));
#22817=CARTESIAN_POINT('Ctrl Pts',(5.11112998264613,-0.552060840994624,
11.051370419133));
#22818=CARTESIAN_POINT('Ctrl Pts',(5.11112998264613,1.61522066995007,11.051370419133));
#22819=CARTESIAN_POINT('Ctrl Pts',(5.28082876351925,-0.552060840994624,
10.9511663773825));
#22820=CARTESIAN_POINT('Ctrl Pts',(5.28082876351925,1.61522066995007,10.9511663773825));
#22821=CARTESIAN_POINT('Ctrl Pts',(5.45051506148977,-0.552060840994624,
10.8599381259735));
#22822=CARTESIAN_POINT('Ctrl Pts',(5.45051506148977,1.61522066995007,10.8599381259735));
#22823=CARTESIAN_POINT('Ctrl Pts',(5.62101499943423,-0.552060840994624,
10.7795199127532));
#22824=CARTESIAN_POINT('Ctrl Pts',(5.62101499943423,1.61522066995007,10.7795199127532));
#22825=CARTESIAN_POINT('Ctrl Pts',(5.7936769541502,-0.552060840994624,10.7114411549111));
#22826=CARTESIAN_POINT('Ctrl Pts',(5.7936769541502,1.61522066995007,10.7114411549111));
#22827=CARTESIAN_POINT('Ctrl Pts',(5.96961932707136,-0.552060840994624,
10.6558377434042));
#22828=CARTESIAN_POINT('Ctrl Pts',(5.96961932707136,1.61522066995007,10.6558377434042));
#22829=CARTESIAN_POINT('Ctrl Pts',(6.14893768388704,-0.552060840994624,
10.6103475969888));
#22830=CARTESIAN_POINT('Ctrl Pts',(6.14893768388704,1.61522066995007,10.6103475969888));
#22831=CARTESIAN_POINT('Ctrl Pts',(6.32976796473819,-0.552060840994624,
10.5687216653907));
#22832=CARTESIAN_POINT('Ctrl Pts',(6.32976796473819,1.61522066995007,10.5687216653907));
#22833=CARTESIAN_POINT('Ctrl Pts',(6.50892555577775,-0.552060840994624,
10.5222908830264));
#22834=CARTESIAN_POINT('Ctrl Pts',(6.50892555577775,1.61522066995007,10.5222908830264));
#22835=CARTESIAN_POINT('Ctrl Pts',(6.68288828293941,-0.552060840994624,
10.462050267878));
#22836=CARTESIAN_POINT('Ctrl Pts',(6.68288828293941,1.61522066995007,10.462050267878));
#22837=CARTESIAN_POINT('Ctrl Pts',(6.84859008776107,-0.552060840994624,
10.3804015453596));
#22838=CARTESIAN_POINT('Ctrl Pts',(6.84859008776107,1.61522066995007,10.3804015453596));
#22839=CARTESIAN_POINT('Ctrl Pts',(7.00445448641038,-0.552060840994624,
10.2733319413005));
#22840=CARTESIAN_POINT('Ctrl Pts',(7.00445448641038,1.61522066995007,10.2733319413005));
#22841=CARTESIAN_POINT('Ctrl Pts',(7.15081550722288,-0.552060840994624,
10.1414720974144));
#22842=CARTESIAN_POINT('Ctrl Pts',(7.15081550722288,1.61522066995007,10.1414720974144));
#22843=CARTESIAN_POINT('Ctrl Pts',(7.28883796912684,-0.552060840994624,
9.98835756998534));
#22844=CARTESIAN_POINT('Ctrl Pts',(7.28883796912684,1.61522066995007,9.98835756998534));
#22845=CARTESIAN_POINT('Ctrl Pts',(7.41967047354988,-0.552060840994624,
9.81917361987377));
#22846=CARTESIAN_POINT('Ctrl Pts',(7.41967047354988,1.61522066995007,9.81917361987377));
#22847=CARTESIAN_POINT('Ctrl Pts',(7.54360573526532,-0.552060840994624,
9.63939026966049));
#22848=CARTESIAN_POINT('Ctrl Pts',(7.54360573526532,1.61522066995007,9.63939026966049));
#22849=CARTESIAN_POINT('Ctrl Pts',(7.6590003866074,-0.552060840994624,9.45324999450471));
#22850=CARTESIAN_POINT('Ctrl Pts',(7.6590003866074,1.61522066995007,9.45324999450471));
#22851=CARTESIAN_POINT('Ctrl Pts',(7.76209282457502,-0.552060840994624,
9.26297089919836));
#22852=CARTESIAN_POINT('Ctrl Pts',(7.76209282457502,1.61522066995007,9.26297089919836));
#22853=CARTESIAN_POINT('Ctrl Pts',(7.84862074946283,-0.552060840994624,
9.06945407017055));
#22854=CARTESIAN_POINT('Ctrl Pts',(7.84862074946283,1.61522066995007,9.06945407017055));
#22855=CARTESIAN_POINT('Ctrl Pts',(7.91508259073031,-0.552060840994624,
8.87266947141857));
#22856=CARTESIAN_POINT('Ctrl Pts',(7.91508259073031,1.61522066995007,8.87266947141857));
#22857=CARTESIAN_POINT('Ctrl Pts',(7.96007609558387,-0.552060840994624,
8.67216210283894));
#22858=CARTESIAN_POINT('Ctrl Pts',(7.96007609558387,1.61522066995007,8.67216210283894));
#22859=CARTESIAN_POINT('Ctrl Pts',(7.98575825096082,-0.552060840994624,
8.46752658699496));
#22860=CARTESIAN_POINT('Ctrl Pts',(7.98575825096082,1.61522066995007,8.46752658699496));
#22861=CARTESIAN_POINT('Ctrl Pts',(7.9987984391963,-0.552060840994624,8.25883677791438));
#22862=CARTESIAN_POINT('Ctrl Pts',(7.9987984391963,1.61522066995007,8.25883677791438));
#22863=CARTESIAN_POINT('Ctrl Pts',(8.00781893805568,-0.552060840994624,
8.04662057355209));
#22864=CARTESIAN_POINT('Ctrl Pts',(8.00781893805568,1.61522066995007,8.04662057355209));
#22865=CARTESIAN_POINT('Ctrl Pts',(8.02124364536257,-0.552060840994624,
7.8318867323277));
#22866=CARTESIAN_POINT('Ctrl Pts',(8.02124364536257,1.61522066995007,7.8318867323277));
#22867=CARTESIAN_POINT('Ctrl Pts',(8.04494633492827,-0.552060840994624,
7.61613341658679));
#22868=CARTESIAN_POINT('Ctrl Pts',(8.04494633492827,1.61522066995007,7.61613341658679));
#22869=CARTESIAN_POINT('Ctrl Pts',(8.08008348678094,-0.552060840994624,
7.40136016279815));
#22870=CARTESIAN_POINT('Ctrl Pts',(8.08008348678094,1.61522066995007,7.40136016279815));
#22871=CARTESIAN_POINT('Ctrl Pts',(8.12057943633426,-0.552060840994624,
7.19009032473197));
#22872=CARTESIAN_POINT('Ctrl Pts',(8.12057943633426,1.61522066995007,7.19009032473197));
#22873=CARTESIAN_POINT('Ctrl Pts',(8.15569042861283,-0.552060840994624,
6.98516923427904));
#22874=CARTESIAN_POINT('Ctrl Pts',(8.15569042861283,1.61522066995007,6.98516923427904));
#22875=CARTESIAN_POINT('Ctrl Pts',(8.17293082304204,-0.552060840994624,
6.78954489191915));
#22876=CARTESIAN_POINT('Ctrl Pts',(8.17293082304204,1.61522066995007,6.78954489191915));
#22877=CARTESIAN_POINT('Ctrl Pts',(8.16089752265956,-0.552060840994624,
6.60605451948904));
#22878=CARTESIAN_POINT('Ctrl Pts',(8.16089752265956,1.61522066995007,6.60605451948904));
#22879=CARTESIAN_POINT('Ctrl Pts',(8.11207116917844,-0.552060840994624,
6.43720976255638));
#22880=CARTESIAN_POINT('Ctrl Pts',(8.11207116917844,1.61522066995007,6.43720976255638));
#22881=CARTESIAN_POINT('Ctrl Pts',(8.02580908828092,-0.552060840994624,
6.28498018271691));
#22882=CARTESIAN_POINT('Ctrl Pts',(8.02580908828092,1.61522066995007,6.28498018271691));
#22883=CARTESIAN_POINT('Ctrl Pts',(7.90644860448881,-0.552060840994624,
6.15052660592943));
#22884=CARTESIAN_POINT('Ctrl Pts',(7.90644860448881,1.61522066995007,6.15052660592943));
#22885=CARTESIAN_POINT('Ctrl Pts',(7.76106756457749,-0.552060840994624,
6.03389995867286));
#22886=CARTESIAN_POINT('Ctrl Pts',(7.76106756457749,1.61522066995007,6.03389995867286));
#22887=CARTESIAN_POINT('Ctrl Pts',(7.59751903688427,-0.552060840994624,
5.93381436957244));
#22888=CARTESIAN_POINT('Ctrl Pts',(7.59751903688427,1.61522066995007,5.93381436957244));
#22889=CARTESIAN_POINT('Ctrl Pts',(7.42198551710643,-0.552060840994624,
5.84723737025948));
#22890=CARTESIAN_POINT('Ctrl Pts',(7.42198551710643,1.61522066995007,5.84723737025948));
#22891=CARTESIAN_POINT('Ctrl Pts',(7.23853768475023,-0.552060840994624,
5.76979878895671));
#22892=CARTESIAN_POINT('Ctrl Pts',(7.23853768475023,1.61522066995007,5.76979878895671));
#22893=CARTESIAN_POINT('Ctrl Pts',(7.04976847947264,-0.552060840994624,
5.69662713609756));
#22894=CARTESIAN_POINT('Ctrl Pts',(7.04976847947264,1.61522066995007,5.69662713609756));
#22895=CARTESIAN_POINT('Ctrl Pts',(6.85709976037512,-0.552060840994624,
5.62308582598972));
#22896=CARTESIAN_POINT('Ctrl Pts',(6.85709976037512,1.61522066995007,5.62308582598972));
#22897=CARTESIAN_POINT('Ctrl Pts',(6.66121503090593,-0.552060840994624,
5.54547963906641));
#22898=CARTESIAN_POINT('Ctrl Pts',(6.66121503090593,1.61522066995007,5.54547963906641));
#22899=CARTESIAN_POINT('Ctrl Pts',(6.46246210121974,-0.552060840994624,
5.46195513100458));
#22900=CARTESIAN_POINT('Ctrl Pts',(6.46246210121974,1.61522066995007,5.46195513100458));
#22901=CARTESIAN_POINT('Ctrl Pts',(6.26112587698791,-0.552060840994624,
5.37226655127806));
#22902=CARTESIAN_POINT('Ctrl Pts',(6.26112587698791,1.61522066995007,5.37226655127806));
#22903=CARTESIAN_POINT('Ctrl Pts',(6.05762450882876,-0.552060840994624,
5.27709955371581));
#22904=CARTESIAN_POINT('Ctrl Pts',(6.05762450882876,1.61522066995007,5.27709955371581));
#22905=CARTESIAN_POINT('Ctrl Pts',(5.85274048349253,-0.552060840994624,
5.17752467829117));
#22906=CARTESIAN_POINT('Ctrl Pts',(5.85274048349253,1.61522066995007,5.17752467829117));
#22907=CARTESIAN_POINT('Ctrl Pts',(5.6478173738032,-0.552060840994624,5.07442896098936));
#22908=CARTESIAN_POINT('Ctrl Pts',(5.6478173738032,1.61522066995007,5.07442896098936));
#22909=CARTESIAN_POINT('Ctrl Pts',(5.44501860313336,-0.552060840994624,
4.96787993373722));
#22910=CARTESIAN_POINT('Ctrl Pts',(5.44501860313336,1.61522066995007,4.96787993373722));
#22911=CARTESIAN_POINT('Ctrl Pts',(5.24741086000008,-0.552060840994624,
4.85676111532844));
#22912=CARTESIAN_POINT('Ctrl Pts',(5.24741086000008,1.61522066995007,4.85676111532844));
#22913=CARTESIAN_POINT('Ctrl Pts',(5.05850630701875,-0.552060840994624,
4.73929437247794));
#22914=CARTESIAN_POINT('Ctrl Pts',(5.05850630701875,1.61522066995007,4.73929437247794));
#22915=CARTESIAN_POINT('Ctrl Pts',(4.88190185104846,-0.552060840994624,
4.61340315498245));
#22916=CARTESIAN_POINT('Ctrl Pts',(4.88190185104846,1.61522066995007,4.61340315498245));
#22917=CARTESIAN_POINT('Ctrl Pts',(4.7208720035032,-0.552060840994624,4.47714872481864));
#22918=CARTESIAN_POINT('Ctrl Pts',(4.7208720035032,1.61522066995007,4.47714872481864));
#22919=CARTESIAN_POINT('Ctrl Pts',(4.57800047823784,-0.552060840994624,
4.32911151507775));
#22920=CARTESIAN_POINT('Ctrl Pts',(4.57800047823784,1.61522066995007,4.32911151507775));
#22921=CARTESIAN_POINT('Ctrl Pts',(4.4547451964031,-0.552060840994624,4.16885849319143));
#22922=CARTESIAN_POINT('Ctrl Pts',(4.4547451964031,1.61522066995007,4.16885849319143));
#22923=CARTESIAN_POINT('Ctrl Pts',(4.35148411330737,-0.552060840994624,
3.99681013615577));
#22924=CARTESIAN_POINT('Ctrl Pts',(4.35148411330737,1.61522066995007,3.99681013615577));
#22925=CARTESIAN_POINT('Ctrl Pts',(4.26765207024408,-0.552060840994624,
3.81399668859083));
#22926=CARTESIAN_POINT('Ctrl Pts',(4.26765207024408,1.61522066995007,3.81399668859083));
#22927=CARTESIAN_POINT('Ctrl Pts',(4.20184334854117,-0.552060840994624,
3.62185203209172));
#22928=CARTESIAN_POINT('Ctrl Pts',(4.20184334854117,1.61522066995007,3.62185203209172));
#22929=CARTESIAN_POINT('Ctrl Pts',(4.15193466045737,-0.552060840994624,
3.42199345348454));
#22930=CARTESIAN_POINT('Ctrl Pts',(4.15193466045737,1.61522066995007,3.42199345348454));
#22931=CARTESIAN_POINT('Ctrl Pts',(4.11518318246501,-0.552060840994624,
3.21600287470933));
#22932=CARTESIAN_POINT('Ctrl Pts',(4.11518318246501,1.61522066995007,3.21600287470933));
#22933=CARTESIAN_POINT('Ctrl Pts',(4.08854433447712,-0.552060840994624,
3.00529120729351));
#22934=CARTESIAN_POINT('Ctrl Pts',(4.08854433447712,1.61522066995007,3.00529120729351));
#22935=CARTESIAN_POINT('Ctrl Pts',(4.06899962712481,-0.552060840994624,
2.7909834104826));
#22936=CARTESIAN_POINT('Ctrl Pts',(4.06899962712481,1.61522066995007,2.7909834104826));
#22937=CARTESIAN_POINT('Ctrl Pts',(4.05390260344518,-0.552060840994624,
2.57377631141663));
#22938=CARTESIAN_POINT('Ctrl Pts',(4.05390260344518,1.61522066995007,2.57377631141663));
#22939=CARTESIAN_POINT('Ctrl Pts',(4.04126813644791,-0.552060840994624,
2.35385258470204));
#22940=CARTESIAN_POINT('Ctrl Pts',(4.04126813644791,1.61522066995007,2.35385258470204));
#22941=CARTESIAN_POINT('Ctrl Pts',(4.03021014446877,-0.552060840994624,
2.13065748555701));
#22942=CARTESIAN_POINT('Ctrl Pts',(4.03021014446877,1.61522066995007,2.13065748555701));
#22943=CARTESIAN_POINT('Ctrl Pts',(4.02066709528519,-0.552060840994624,
1.9033255681334));
#22944=CARTESIAN_POINT('Ctrl Pts',(4.02066709528519,1.61522066995007,1.9033255681334));
#22945=CARTESIAN_POINT('Ctrl Pts',(4.012782399266,-0.552060840994624,1.67142113207676));
#22946=CARTESIAN_POINT('Ctrl Pts',(4.012782399266,1.61522066995007,1.67142113207676));
#22947=CARTESIAN_POINT('Ctrl Pts',(4.00639322616619,-0.552060840994624,
1.4355810193293));
#22948=CARTESIAN_POINT('Ctrl Pts',(4.00639322616619,1.61522066995007,1.4355810193293));
#22949=CARTESIAN_POINT('Ctrl Pts',(4.00047520099043,-0.552060840994624,
1.19819542279832));
#22950=CARTESIAN_POINT('Ctrl Pts',(4.00047520099043,1.61522066995007,1.19819542279832));
#22951=CARTESIAN_POINT('Ctrl Pts',(3.99260375067002,-0.552060840994624,
0.964078729991153));
#22952=CARTESIAN_POINT('Ctrl Pts',(3.99260375067002,1.61522066995007,0.964078729991153));
#22953=CARTESIAN_POINT('Ctrl Pts',(3.97841403016118,-0.552060840994624,
0.741129277895168));
#22954=CARTESIAN_POINT('Ctrl Pts',(3.97841403016118,1.61522066995007,0.741129277895168));
#22955=CARTESIAN_POINT('Ctrl Pts',(3.95259200169988,-0.552060840994624,
0.538436816836329));
#22956=CARTESIAN_POINT('Ctrl Pts',(3.95259200169988,1.61522066995007,0.538436816836329));
#22957=CARTESIAN_POINT('Ctrl Pts',(3.90986572419832,-0.552060840994624,
0.364350357241537));
#22958=CARTESIAN_POINT('Ctrl Pts',(3.90986572419832,1.61522066995007,0.364350357241537));
#22959=CARTESIAN_POINT('Ctrl Pts',(3.84598208672298,-0.552060840994624,
0.224659532804428));
#22960=CARTESIAN_POINT('Ctrl Pts',(3.84598208672298,1.61522066995007,0.224659532804428));
#22961=CARTESIAN_POINT('Ctrl Pts',(3.75872318140661,-0.552060840994624,
0.120497232333236));
#22962=CARTESIAN_POINT('Ctrl Pts',(3.75872318140661,1.61522066995007,0.120497232333236));
#22963=CARTESIAN_POINT('Ctrl Pts',(3.64881642260075,-0.552060840994624,
0.0470540298718229));
#22964=CARTESIAN_POINT('Ctrl Pts',(3.64881642260075,1.61522066995007,0.0470540298718229));
#22965=CARTESIAN_POINT('Ctrl Pts',(3.52045328348988,-0.552060840994624,
-0.00118366394786523));
#22966=CARTESIAN_POINT('Ctrl Pts',(3.52045328348988,1.61522066995007,-0.00118366394786523));
#22967=CARTESIAN_POINT('Ctrl Pts',(3.3816469894381,-0.552060840994624,-0.0263068037111615));
#22968=CARTESIAN_POINT('Ctrl Pts',(3.3816469894381,1.61522066995007,-0.0263068037111615));
#22969=CARTESIAN_POINT('Ctrl Pts',(3.2451100102617,-0.552060840994624,-0.0214179570895094));
#22970=CARTESIAN_POINT('Ctrl Pts',(3.2451100102617,1.61522066995007,-0.0214179570895094));
#22971=CARTESIAN_POINT('Ctrl Pts',(3.12452733970665,-0.552060840994624,
0.0241851999814078));
#22972=CARTESIAN_POINT('Ctrl Pts',(3.12452733970665,1.61522066995007,0.0241851999814078));
#22973=CARTESIAN_POINT('Ctrl Pts',(3.03063129752059,-0.552060840994624,
0.119017371327004));
#22974=CARTESIAN_POINT('Ctrl Pts',(3.03063129752059,1.61522066995007,0.119017371327004));
#22975=CARTESIAN_POINT('Ctrl Pts',(2.96639254265844,-0.552060840994624,
0.262319630540593));
#22976=CARTESIAN_POINT('Ctrl Pts',(2.96639254265844,1.61522066995007,0.262319630540593));
#22977=CARTESIAN_POINT('Ctrl Pts',(2.92780415844446,-0.552060840994624,
0.444963858672424));
#22978=CARTESIAN_POINT('Ctrl Pts',(2.92780415844446,1.61522066995007,0.444963858672424));
#22979=CARTESIAN_POINT('Ctrl Pts',(2.90717911786689,-0.552060840994624,
0.65402023086958));
#22980=CARTESIAN_POINT('Ctrl Pts',(2.90717911786689,1.61522066995007,0.65402023086958));
#22981=CARTESIAN_POINT('Ctrl Pts',(2.89547076625581,-0.552060840994624,
0.875890304828918));
#22982=CARTESIAN_POINT('Ctrl Pts',(2.89547076625581,1.61522066995007,0.875890304828918));
#22983=CARTESIAN_POINT('Ctrl Pts',(2.88537704766906,-0.552060840994624,
1.10060381648398));
#22984=CARTESIAN_POINT('Ctrl Pts',(2.88537704766906,1.61522066995007,1.10060381648398));
#22985=CARTESIAN_POINT('Ctrl Pts',(2.8728456296504,-0.552060840994624,1.32371934078733));
#22986=CARTESIAN_POINT('Ctrl Pts',(2.8728456296504,1.61522066995007,1.32371934078733));
#22987=CARTESIAN_POINT('Ctrl Pts',(2.85578261679345,-0.552060840994624,
1.54401727992264));
#22988=CARTESIAN_POINT('Ctrl Pts',(2.85578261679345,1.61522066995007,1.54401727992264));
#22989=CARTESIAN_POINT('Ctrl Pts',(2.83335686249019,-0.552060840994624,
1.76209503442146));
#22990=CARTESIAN_POINT('Ctrl Pts',(2.83335686249019,1.61522066995007,1.76209503442146));
#22991=CARTESIAN_POINT('Ctrl Pts',(2.80505146480345,-0.552060840994624,
1.97856787413951));
#22992=CARTESIAN_POINT('Ctrl Pts',(2.80505146480345,1.61522066995007,1.97856787413951));
#22993=CARTESIAN_POINT('Ctrl Pts',(2.76985908233915,-0.552060840994624,
2.19251877196071));
#22994=CARTESIAN_POINT('Ctrl Pts',(2.76985908233915,1.61522066995007,2.19251877196071));
#22995=CARTESIAN_POINT('Ctrl Pts',(2.72531955636536,-0.552060840994624,
2.39962532458029));
#22996=CARTESIAN_POINT('Ctrl Pts',(2.72531955636536,1.61522066995007,2.39962532458029));
#22997=CARTESIAN_POINT('Ctrl Pts',(2.66797634363184,-0.552060840994624,
2.59347738935741));
#22998=CARTESIAN_POINT('Ctrl Pts',(2.66797634363184,1.61522066995007,2.59347738935741));
#22999=CARTESIAN_POINT('Ctrl Pts',(2.59397540849171,-0.552060840994624,
2.7672283971178));
#23000=CARTESIAN_POINT('Ctrl Pts',(2.59397540849171,1.61522066995007,2.7672283971178));
#23001=CARTESIAN_POINT('Ctrl Pts',(2.49960870420485,-0.552060840994624,
2.91510580081997));
#23002=CARTESIAN_POINT('Ctrl Pts',(2.49960870420485,1.61522066995007,2.91510580081997));
#23003=CARTESIAN_POINT('Ctrl Pts',(2.38189256086504,-0.552060840994624,
3.03403241435618));
#23004=CARTESIAN_POINT('Ctrl Pts',(2.38189256086504,1.61522066995007,3.03403241435618));
#23005=CARTESIAN_POINT('Ctrl Pts',(2.23909845280558,-0.552060840994624,
3.12505646843308));
#23006=CARTESIAN_POINT('Ctrl Pts',(2.23909845280558,1.61522066995007,3.12505646843308));
#23007=CARTESIAN_POINT('Ctrl Pts',(2.07061055216582,-0.552060840994624,
3.19196918412265));
#23008=CARTESIAN_POINT('Ctrl Pts',(2.07061055216582,1.61522066995007,3.19196918412265));
#23009=CARTESIAN_POINT('Ctrl Pts',(1.87681490437036,-0.552060840994624,
3.24001322621211));
#23010=CARTESIAN_POINT('Ctrl Pts',(1.87681490437036,1.61522066995007,3.24001322621211));
#23011=CARTESIAN_POINT('Ctrl Pts',(1.65897747541321,-0.552060840994624,
3.27464765209773));
#23012=CARTESIAN_POINT('Ctrl Pts',(1.65897747541321,1.61522066995007,3.27464765209773));
#23013=CARTESIAN_POINT('Ctrl Pts',(1.4191255439272,-0.552060840994624,3.30006519349576));
#23014=CARTESIAN_POINT('Ctrl Pts',(1.4191255439272,1.61522066995007,3.30006519349576));
#23015=CARTESIAN_POINT('Ctrl Pts',(1.15993538533448,-0.552060840994624,
3.31897283641381));
#23016=CARTESIAN_POINT('Ctrl Pts',(1.15993538533448,1.61522066995007,3.31897283641381));
#23017=CARTESIAN_POINT('Ctrl Pts',(0.884625090385968,-0.552060840994624,
3.33300441174764));
#23018=CARTESIAN_POINT('Ctrl Pts',(0.884625090385968,1.61522066995007,3.33300441174764));
#23019=CARTESIAN_POINT('Ctrl Pts',(0.596845720618978,-0.552060840994624,
3.34293392264922));
#23020=CARTESIAN_POINT('Ctrl Pts',(0.596845720618978,1.61522066995007,3.34293392264922));
#23021=CARTESIAN_POINT('Ctrl Pts',(0.30057321210183,-0.552060840994624,
3.34897162637417));
#23022=CARTESIAN_POINT('Ctrl Pts',(0.30057321210183,1.61522066995007,3.34897162637417));
#23023=CARTESIAN_POINT('Ctrl Pts',(1.66741620510891E-14,-0.552060840994624,
3.35102435732185));
#23024=CARTESIAN_POINT('Ctrl Pts',(1.66741620510891E-14,1.61522066995007,
3.35102435732185));
#23025=CARTESIAN_POINT('Ctrl Pts',(-0.300573212101791,-0.552060840994624,
3.34897162637426));
#23026=CARTESIAN_POINT('Ctrl Pts',(-0.300573212101791,1.61522066995007,
3.34897162637426));
#23027=CARTESIAN_POINT('Ctrl Pts',(-0.596845720618908,-0.552060840994624,
3.34293392264938));
#23028=CARTESIAN_POINT('Ctrl Pts',(-0.596845720618908,1.61522066995007,
3.34293392264938));
#23029=CARTESIAN_POINT('Ctrl Pts',(-0.884625090385886,-0.552060840994624,
3.33300441174785));
#23030=CARTESIAN_POINT('Ctrl Pts',(-0.884625090385886,1.61522066995007,
3.33300441174785));
#23031=CARTESIAN_POINT('Ctrl Pts',(-1.15993538533442,-0.552060840994624,
3.31897283641402));
#23032=CARTESIAN_POINT('Ctrl Pts',(-1.15993538533442,1.61522066995007,3.31897283641402));
#23033=CARTESIAN_POINT('Ctrl Pts',(-1.41912554392716,-0.552060840994624,
3.30006519349591));
#23034=CARTESIAN_POINT('Ctrl Pts',(-1.41912554392716,1.61522066995007,3.30006519349591));
#23035=CARTESIAN_POINT('Ctrl Pts',(-1.65897747541319,-0.552060840994624,
3.27464765209779));
#23036=CARTESIAN_POINT('Ctrl Pts',(-1.65897747541319,1.61522066995007,3.27464765209779));
#23037=CARTESIAN_POINT('Ctrl Pts',(-1.87681490437034,-0.552060840994624,
3.24001322621208));
#23038=CARTESIAN_POINT('Ctrl Pts',(-1.87681490437034,1.61522066995007,3.24001322621208));
#23039=CARTESIAN_POINT('Ctrl Pts',(-2.07061055216576,-0.552060840994624,
3.19196918412254));
#23040=CARTESIAN_POINT('Ctrl Pts',(-2.07061055216576,1.61522066995007,3.19196918412254));
#23041=CARTESIAN_POINT('Ctrl Pts',(-2.23909845280547,-0.552060840994624,
3.12505646843295));
#23042=CARTESIAN_POINT('Ctrl Pts',(-2.23909845280547,1.61522066995007,3.12505646843295));
#23043=CARTESIAN_POINT('Ctrl Pts',(-2.38189256086493,-0.552060840994624,
3.03403241435609));
#23044=CARTESIAN_POINT('Ctrl Pts',(-2.38189256086493,1.61522066995007,3.03403241435609));
#23045=CARTESIAN_POINT('Ctrl Pts',(-2.49960870420481,-0.552060840994624,
2.91510580081997));
#23046=CARTESIAN_POINT('Ctrl Pts',(-2.49960870420481,1.61522066995007,2.91510580081997));
#23047=CARTESIAN_POINT('Ctrl Pts',(-2.59397540849182,-0.552060840994624,
2.76722839711793));
#23048=CARTESIAN_POINT('Ctrl Pts',(-2.59397540849182,1.61522066995007,2.76722839711793));
#23049=CARTESIAN_POINT('Ctrl Pts',(-2.66797634363209,-0.552060840994624,
2.59347738935767));
#23050=CARTESIAN_POINT('Ctrl Pts',(-2.66797634363209,1.61522066995007,2.59347738935767));
#23051=CARTESIAN_POINT('Ctrl Pts',(-2.72531955636566,-0.552060840994624,
2.39962532458057));
#23052=CARTESIAN_POINT('Ctrl Pts',(-2.72531955636566,1.61522066995007,2.39962532458057));
#23053=CARTESIAN_POINT('Ctrl Pts',(-2.76985908233936,-0.552060840994624,
2.19251877196088));
#23054=CARTESIAN_POINT('Ctrl Pts',(-2.76985908233936,1.61522066995007,2.19251877196088));
#23055=CARTESIAN_POINT('Ctrl Pts',(-2.80505146480344,-0.552060840994624,
1.97856787413951));
#23056=CARTESIAN_POINT('Ctrl Pts',(-2.80505146480344,1.61522066995007,1.97856787413951));
#23057=CARTESIAN_POINT('Ctrl Pts',(-2.8333568624899,-0.552060840994624,
1.76209503442131));
#23058=CARTESIAN_POINT('Ctrl Pts',(-2.8333568624899,1.61522066995007,1.76209503442131));
#23059=CARTESIAN_POINT('Ctrl Pts',(-2.85578261679294,-0.552060840994624,
1.54401727992238));
#23060=CARTESIAN_POINT('Ctrl Pts',(-2.85578261679294,1.61522066995007,1.54401727992238));
#23061=CARTESIAN_POINT('Ctrl Pts',(-2.87284562964987,-0.552060840994624,
1.32371934078708));
#23062=CARTESIAN_POINT('Ctrl Pts',(-2.87284562964987,1.61522066995007,1.32371934078708));
#23063=CARTESIAN_POINT('Ctrl Pts',(-2.88537704766869,-0.552060840994624,
1.10060381648384));
#23064=CARTESIAN_POINT('Ctrl Pts',(-2.88537704766869,1.61522066995007,1.10060381648384));
#23065=CARTESIAN_POINT('Ctrl Pts',(-2.89547076625573,-0.552060840994624,
0.875890304828914));
#23066=CARTESIAN_POINT('Ctrl Pts',(-2.89547076625573,1.61522066995007,0.875890304828914));
#23067=CARTESIAN_POINT('Ctrl Pts',(-2.90717911786707,-0.552060840994624,
0.654020230869684));
#23068=CARTESIAN_POINT('Ctrl Pts',(-2.90717911786707,1.61522066995007,0.654020230869684));
#23069=CARTESIAN_POINT('Ctrl Pts',(-2.92780415844476,-0.552060840994624,
0.444963858672577));
#23070=CARTESIAN_POINT('Ctrl Pts',(-2.92780415844476,1.61522066995007,0.444963858672577));
#23071=CARTESIAN_POINT('Ctrl Pts',(-2.96639254265869,-0.552060840994624,
0.262319630540737));
#23072=CARTESIAN_POINT('Ctrl Pts',(-2.96639254265869,1.61522066995007,0.262319630540737));
#23073=CARTESIAN_POINT('Ctrl Pts',(-3.03063129752067,-0.552060840994624,
0.11901737132707));
#23074=CARTESIAN_POINT('Ctrl Pts',(-3.03063129752067,1.61522066995007,0.11901737132707));
#23075=CARTESIAN_POINT('Ctrl Pts',(-3.12452733970658,-0.552060840994624,
0.0241851999813871));
#23076=CARTESIAN_POINT('Ctrl Pts',(-3.12452733970658,1.61522066995007,0.0241851999813871));
#23077=CARTESIAN_POINT('Ctrl Pts',(-3.24511001026157,-0.552060840994624,
-0.0214179570895714));
#23078=CARTESIAN_POINT('Ctrl Pts',(-3.24511001026157,1.61522066995007,-0.0214179570895714));
#23079=CARTESIAN_POINT('Ctrl Pts',(-3.38164698943802,-0.552060840994624,
-0.0263068037112043));
#23080=CARTESIAN_POINT('Ctrl Pts',(-3.38164698943802,1.61522066995007,-0.0263068037112043));
#23081=CARTESIAN_POINT('Ctrl Pts',(-3.52045328348989,-0.552060840994624,
-0.00118366394785932));
#23082=CARTESIAN_POINT('Ctrl Pts',(-3.52045328348989,1.61522066995007,-0.00118366394785932));
#23083=CARTESIAN_POINT('Ctrl Pts',(-3.64881642260079,-0.552060840994624,
0.0470540298718583));
#23084=CARTESIAN_POINT('Ctrl Pts',(-3.64881642260079,1.61522066995007,0.0470540298718583));
#23085=CARTESIAN_POINT('Ctrl Pts',(-3.75872318140663,-0.552060840994624,
0.120497232333251));
#23086=CARTESIAN_POINT('Ctrl Pts',(-3.75872318140663,1.61522066995007,0.120497232333251));
#23087=CARTESIAN_POINT('Ctrl Pts',(-3.84598208672296,-0.552060840994624,
0.224659532804408));
#23088=CARTESIAN_POINT('Ctrl Pts',(-3.84598208672296,1.61522066995007,0.224659532804408));
#23089=CARTESIAN_POINT('Ctrl Pts',(-3.9098657241983,-0.552060840994624,
0.364350357241515));
#23090=CARTESIAN_POINT('Ctrl Pts',(-3.9098657241983,1.61522066995007,0.364350357241515));
#23091=CARTESIAN_POINT('Ctrl Pts',(-3.9525920016999,-0.552060840994624,
0.538436816836325));
#23092=CARTESIAN_POINT('Ctrl Pts',(-3.9525920016999,1.61522066995007,0.538436816836325));
#23093=CARTESIAN_POINT('Ctrl Pts',(-3.97841403016126,-0.552060840994624,
0.741129277895169));
#23094=CARTESIAN_POINT('Ctrl Pts',(-3.97841403016126,1.61522066995007,0.741129277895169));
#23095=CARTESIAN_POINT('Ctrl Pts',(-3.99260375067011,-0.552060840994624,
0.964078729991154));
#23096=CARTESIAN_POINT('Ctrl Pts',(-3.99260375067011,1.61522066995007,0.964078729991154));
#23097=CARTESIAN_POINT('Ctrl Pts',(-4.00047520099045,-0.552060840994624,
1.1981954227983));
#23098=CARTESIAN_POINT('Ctrl Pts',(-4.00047520099045,1.61522066995007,1.1981954227983));
#23099=CARTESIAN_POINT('Ctrl Pts',(-4.00639322616607,-0.552060840994624,
1.43558101932923));
#23100=CARTESIAN_POINT('Ctrl Pts',(-4.00639322616607,1.61522066995007,1.43558101932923));
#23101=CARTESIAN_POINT('Ctrl Pts',(-4.01278239926574,-0.552060840994624,
1.67142113207667));
#23102=CARTESIAN_POINT('Ctrl Pts',(-4.01278239926574,1.61522066995007,1.67142113207667));
#23103=CARTESIAN_POINT('Ctrl Pts',(-4.02066709528487,-0.552060840994624,
1.90332556813333));
#23104=CARTESIAN_POINT('Ctrl Pts',(-4.02066709528487,1.61522066995007,1.90332556813333));
#23105=CARTESIAN_POINT('Ctrl Pts',(-4.0302101444685,-0.552060840994624,
2.130657485557));
#23106=CARTESIAN_POINT('Ctrl Pts',(-4.0302101444685,1.61522066995007,2.130657485557));
#23107=CARTESIAN_POINT('Ctrl Pts',(-4.04126813644779,-0.552060840994624,
2.35385258470204));
#23108=CARTESIAN_POINT('Ctrl Pts',(-4.04126813644779,1.61522066995007,2.35385258470204));
#23109=CARTESIAN_POINT('Ctrl Pts',(-4.05390260344525,-0.552060840994624,
2.57377631141659));
#23110=CARTESIAN_POINT('Ctrl Pts',(-4.05390260344525,1.61522066995007,2.57377631141659));
#23111=CARTESIAN_POINT('Ctrl Pts',(-4.06899962712502,-0.552060840994624,
2.7909834104825));
#23112=CARTESIAN_POINT('Ctrl Pts',(-4.06899962712502,1.61522066995007,2.7909834104825));
#23113=CARTESIAN_POINT('Ctrl Pts',(-4.08854433447739,-0.552060840994624,
3.00529120729338));
#23114=CARTESIAN_POINT('Ctrl Pts',(-4.08854433447739,1.61522066995007,3.00529120729338));
#23115=CARTESIAN_POINT('Ctrl Pts',(-4.11518318246524,-0.552060840994624,
3.21600287470921));
#23116=CARTESIAN_POINT('Ctrl Pts',(-4.11518318246524,1.61522066995007,3.21600287470921));
#23117=CARTESIAN_POINT('Ctrl Pts',(-4.15193466045748,-0.552060840994624,
3.42199345348447));
#23118=CARTESIAN_POINT('Ctrl Pts',(-4.15193466045748,1.61522066995007,3.42199345348447));
#23119=CARTESIAN_POINT('Ctrl Pts',(-4.20184334854115,-0.552060840994624,
3.62185203209171));
#23120=CARTESIAN_POINT('Ctrl Pts',(-4.20184334854115,1.61522066995007,3.62185203209171));
#23121=CARTESIAN_POINT('Ctrl Pts',(-4.26765207024395,-0.552060840994624,
3.81399668859083));
#23122=CARTESIAN_POINT('Ctrl Pts',(-4.26765207024395,1.61522066995007,3.81399668859083));
#23123=CARTESIAN_POINT('Ctrl Pts',(-4.35148411330718,-0.552060840994624,
3.99681013615577));
#23124=CARTESIAN_POINT('Ctrl Pts',(-4.35148411330718,1.61522066995007,3.99681013615577));
#23125=CARTESIAN_POINT('Ctrl Pts',(-4.45474519640294,-0.552060840994624,
4.16885849319142));
#23126=CARTESIAN_POINT('Ctrl Pts',(-4.45474519640294,1.61522066995007,4.16885849319142));
#23127=CARTESIAN_POINT('Ctrl Pts',(-4.57800047823775,-0.552060840994624,
4.32911151507774));
#23128=CARTESIAN_POINT('Ctrl Pts',(-4.57800047823775,1.61522066995007,4.32911151507774));
#23129=CARTESIAN_POINT('Ctrl Pts',(-4.7208720035032,-0.552060840994624,
4.47714872481861));
#23130=CARTESIAN_POINT('Ctrl Pts',(-4.7208720035032,1.61522066995007,4.47714872481861));
#23131=CARTESIAN_POINT('Ctrl Pts',(-4.88190185104852,-0.552060840994624,
4.61340315498244));
#23132=CARTESIAN_POINT('Ctrl Pts',(-4.88190185104852,1.61522066995007,4.61340315498244));
#23133=CARTESIAN_POINT('Ctrl Pts',(-5.05850630701885,-0.552060840994624,
4.73929437247796));
#23134=CARTESIAN_POINT('Ctrl Pts',(-5.05850630701885,1.61522066995007,4.73929437247796));
#23135=CARTESIAN_POINT('Ctrl Pts',(-5.24741086000019,-0.552060840994624,
4.8567611153285));
#23136=CARTESIAN_POINT('Ctrl Pts',(-5.24741086000019,1.61522066995007,4.8567611153285));
#23137=CARTESIAN_POINT('Ctrl Pts',(-5.44501860313342,-0.552060840994624,
4.96787993373728));
#23138=CARTESIAN_POINT('Ctrl Pts',(-5.44501860313342,1.61522066995007,4.96787993373728));
#23139=CARTESIAN_POINT('Ctrl Pts',(-5.64781737380319,-0.552060840994624,
5.07442896098937));
#23140=CARTESIAN_POINT('Ctrl Pts',(-5.64781737380319,1.61522066995007,5.07442896098937));
#23141=CARTESIAN_POINT('Ctrl Pts',(-5.85274048349242,-0.552060840994624,
5.17752467829109));
#23142=CARTESIAN_POINT('Ctrl Pts',(-5.85274048349242,1.61522066995007,5.17752467829109));
#23143=CARTESIAN_POINT('Ctrl Pts',(-6.05762450882858,-0.552060840994624,
5.27709955371564));
#23144=CARTESIAN_POINT('Ctrl Pts',(-6.05762450882858,1.61522066995007,5.27709955371564));
#23145=CARTESIAN_POINT('Ctrl Pts',(-6.26112587698772,-0.552060840994624,
5.37226655127787));
#23146=CARTESIAN_POINT('Ctrl Pts',(-6.26112587698772,1.61522066995007,5.37226655127787));
#23147=CARTESIAN_POINT('Ctrl Pts',(-6.46246210121964,-0.552060840994624,
5.46195513100446));
#23148=CARTESIAN_POINT('Ctrl Pts',(-6.46246210121964,1.61522066995007,5.46195513100446));
#23149=CARTESIAN_POINT('Ctrl Pts',(-6.66121503090592,-0.552060840994624,
5.54547963906637));
#23150=CARTESIAN_POINT('Ctrl Pts',(-6.66121503090592,1.61522066995007,5.54547963906637));
#23151=CARTESIAN_POINT('Ctrl Pts',(-6.8570997603751,-0.552060840994624,
5.62308582598972));
#23152=CARTESIAN_POINT('Ctrl Pts',(-6.8570997603751,1.61522066995007,5.62308582598972));
#23153=CARTESIAN_POINT('Ctrl Pts',(-7.04976847947249,-0.552060840994624,
5.69662713609756));
#23154=CARTESIAN_POINT('Ctrl Pts',(-7.04976847947249,1.61522066995007,5.69662713609756));
#23155=CARTESIAN_POINT('Ctrl Pts',(-7.23853768475,-0.552060840994624,5.76979878895672));
#23156=CARTESIAN_POINT('Ctrl Pts',(-7.23853768475,1.61522066995007,5.76979878895672));
#23157=CARTESIAN_POINT('Ctrl Pts',(-7.42198551710617,-0.552060840994624,
5.84723737025949));
#23158=CARTESIAN_POINT('Ctrl Pts',(-7.42198551710617,1.61522066995007,5.84723737025949));
#23159=CARTESIAN_POINT('Ctrl Pts',(-7.59751903688412,-0.552060840994624,
5.93381436957244));
#23160=CARTESIAN_POINT('Ctrl Pts',(-7.59751903688412,1.61522066995007,5.93381436957244));
#23161=CARTESIAN_POINT('Ctrl Pts',(-7.76106756457753,-0.552060840994624,
6.03389995867283));
#23162=CARTESIAN_POINT('Ctrl Pts',(-7.76106756457753,1.61522066995007,6.03389995867283));
#23163=CARTESIAN_POINT('Ctrl Pts',(-7.90644860448901,-0.552060840994624,
6.15052660592937));
#23164=CARTESIAN_POINT('Ctrl Pts',(-7.90644860448901,1.61522066995007,6.15052660592937));
#23165=CARTESIAN_POINT('Ctrl Pts',(-8.02580908828117,-0.552060840994624,
6.28498018271686));
#23166=CARTESIAN_POINT('Ctrl Pts',(-8.02580908828117,1.61522066995007,6.28498018271686));
#23167=CARTESIAN_POINT('Ctrl Pts',(-8.11207116917861,-0.552060840994624,
6.43720976255636));
#23168=CARTESIAN_POINT('Ctrl Pts',(-8.11207116917861,1.61522066995007,6.43720976255636));
#23169=CARTESIAN_POINT('Ctrl Pts',(-8.16089752265956,-0.552060840994624,
6.60605451948903));
#23170=CARTESIAN_POINT('Ctrl Pts',(-8.16089752265956,1.61522066995007,6.60605451948903));
#23171=CARTESIAN_POINT('Ctrl Pts',(-8.17293082304181,-0.552060840994624,
6.78954489191904));
#23172=CARTESIAN_POINT('Ctrl Pts',(-8.17293082304181,1.61522066995007,6.78954489191904));
#23173=CARTESIAN_POINT('Ctrl Pts',(-8.15569042861244,-0.552060840994624,
6.9851692342788));
#23174=CARTESIAN_POINT('Ctrl Pts',(-8.15569042861244,1.61522066995007,6.9851692342788));
#23175=CARTESIAN_POINT('Ctrl Pts',(-8.12057943633387,-0.552060840994624,
7.19009032473164));
#23176=CARTESIAN_POINT('Ctrl Pts',(-8.12057943633387,1.61522066995007,7.19009032473164));
#23177=CARTESIAN_POINT('Ctrl Pts',(-8.08008348678073,-0.552060840994624,
7.40136016279791));
#23178=CARTESIAN_POINT('Ctrl Pts',(-8.08008348678073,1.61522066995007,7.40136016279791));
#23179=CARTESIAN_POINT('Ctrl Pts',(-8.04494633492831,-0.552060840994624,
7.61613341658677));
#23180=CARTESIAN_POINT('Ctrl Pts',(-8.04494633492831,1.61522066995007,7.61613341658677));
#23181=CARTESIAN_POINT('Ctrl Pts',(-8.02124364536279,-0.552060840994624,
7.83188673232793));
#23182=CARTESIAN_POINT('Ctrl Pts',(-8.02124364536279,1.61522066995007,7.83188673232793));
#23183=CARTESIAN_POINT('Ctrl Pts',(-8.007818938056,-0.552060840994624,8.04662057355248));
#23184=CARTESIAN_POINT('Ctrl Pts',(-8.007818938056,1.61522066995007,8.04662057355248));
#23185=CARTESIAN_POINT('Ctrl Pts',(-7.99879843919661,-0.552060840994624,
8.25883677791483));
#23186=CARTESIAN_POINT('Ctrl Pts',(-7.99879843919661,1.61522066995007,8.25883677791483));
#23187=CARTESIAN_POINT('Ctrl Pts',(-7.98575825096101,-0.552060840994624,
8.46752658699528));
#23188=CARTESIAN_POINT('Ctrl Pts',(-7.98575825096101,1.61522066995007,8.46752658699528));
#23189=CARTESIAN_POINT('Ctrl Pts',(-7.96007609558389,-0.552060840994624,
8.67216210283896));
#23190=CARTESIAN_POINT('Ctrl Pts',(-7.96007609558389,1.61522066995007,8.67216210283896));
#23191=CARTESIAN_POINT('Ctrl Pts',(-7.91508259073019,-0.552060840994624,
8.87266947141823));
#23192=CARTESIAN_POINT('Ctrl Pts',(-7.91508259073019,1.61522066995007,8.87266947141823));
#23193=CARTESIAN_POINT('Ctrl Pts',(-7.84862074946261,-0.552060840994624,
9.06945407016992));
#23194=CARTESIAN_POINT('Ctrl Pts',(-7.84862074946261,1.61522066995007,9.06945407016992));
#23195=CARTESIAN_POINT('Ctrl Pts',(-7.76209282457479,-0.552060840994624,
9.26297089919765));
#23196=CARTESIAN_POINT('Ctrl Pts',(-7.76209282457479,1.61522066995007,9.26297089919765));
#23197=CARTESIAN_POINT('Ctrl Pts',(-7.65900038660722,-0.552060840994624,
9.4532499945042));
#23198=CARTESIAN_POINT('Ctrl Pts',(-7.65900038660722,1.61522066995007,9.4532499945042));
#23199=CARTESIAN_POINT('Ctrl Pts',(-7.5436057352653,-0.552060840994624,
9.63939026966035));
#23200=CARTESIAN_POINT('Ctrl Pts',(-7.5436057352653,1.61522066995007,9.63939026966035));
#23201=CARTESIAN_POINT('Ctrl Pts',(-7.41967047355001,-0.552060840994624,
9.81917361987397));
#23202=CARTESIAN_POINT('Ctrl Pts',(-7.41967047355001,1.61522066995007,9.81917361987397));
#23203=CARTESIAN_POINT('Ctrl Pts',(-7.28883796912703,-0.552060840994624,
9.98835756998572));
#23204=CARTESIAN_POINT('Ctrl Pts',(-7.28883796912703,1.61522066995007,9.98835756998572));
#23205=CARTESIAN_POINT('Ctrl Pts',(-7.15081550722306,-0.552060840994624,
10.1414720974148));
#23206=CARTESIAN_POINT('Ctrl Pts',(-7.15081550722306,1.61522066995007,10.1414720974148));
#23207=CARTESIAN_POINT('Ctrl Pts',(-7.0044544864105,-0.552060840994624,
10.2733319413008));
#23208=CARTESIAN_POINT('Ctrl Pts',(-7.0044544864105,1.61522066995007,10.2733319413008));
#23209=CARTESIAN_POINT('Ctrl Pts',(-6.84859008776113,-0.552060840994624,
10.3804015453596));
#23210=CARTESIAN_POINT('Ctrl Pts',(-6.84859008776113,1.61522066995007,10.3804015453596));
#23211=CARTESIAN_POINT('Ctrl Pts',(-6.68288828293938,-0.552060840994624,
10.4620502678778));
#23212=CARTESIAN_POINT('Ctrl Pts',(-6.68288828293938,1.61522066995007,10.4620502678778));
#23213=CARTESIAN_POINT('Ctrl Pts',(-6.50892555577766,-0.552060840994624,
10.522290883026));
#23214=CARTESIAN_POINT('Ctrl Pts',(-6.50892555577766,1.61522066995007,10.522290883026));
#23215=CARTESIAN_POINT('Ctrl Pts',(-6.32976796473811,-0.552060840994624,
10.5687216653902));
#23216=CARTESIAN_POINT('Ctrl Pts',(-6.32976796473811,1.61522066995007,10.5687216653902));
#23217=CARTESIAN_POINT('Ctrl Pts',(-6.14893768388701,-0.552060840994624,
10.6103475969885));
#23218=CARTESIAN_POINT('Ctrl Pts',(-6.14893768388701,1.61522066995007,10.6103475969885));
#23219=CARTESIAN_POINT('Ctrl Pts',(-5.96961932707142,-0.552060840994624,
10.6558377434043));
#23220=CARTESIAN_POINT('Ctrl Pts',(-5.96961932707142,1.61522066995007,10.6558377434043));
#23221=CARTESIAN_POINT('Ctrl Pts',(-5.79367695415031,-0.552060840994624,
10.7114411549114));
#23222=CARTESIAN_POINT('Ctrl Pts',(-5.79367695415031,1.61522066995007,10.7114411549114));
#23223=CARTESIAN_POINT('Ctrl Pts',(-5.62101499943431,-0.552060840994624,
10.7795199127535));
#23224=CARTESIAN_POINT('Ctrl Pts',(-5.62101499943431,1.61522066995007,10.7795199127535));
#23225=CARTESIAN_POINT('Ctrl Pts',(-5.45051506148982,-0.552060840994624,
10.8599381259737));
#23226=CARTESIAN_POINT('Ctrl Pts',(-5.45051506148982,1.61522066995007,10.8599381259737));
#23227=CARTESIAN_POINT('Ctrl Pts',(-5.28082876351929,-0.552060840994624,
10.9511663773826));
#23228=CARTESIAN_POINT('Ctrl Pts',(-5.28082876351929,1.61522066995007,10.9511663773826));
#23229=CARTESIAN_POINT('Ctrl Pts',(-5.11112998264616,-0.552060840994624,
11.0513704191329));
#23230=CARTESIAN_POINT('Ctrl Pts',(-5.11112998264616,1.61522066995007,11.0513704191329));
#23231=CARTESIAN_POINT('Ctrl Pts',(-4.94211773226973,-0.552060840994624,
11.1598106424589));
#23232=CARTESIAN_POINT('Ctrl Pts',(-4.94211773226973,1.61522066995007,11.1598106424589));
#23233=CARTESIAN_POINT('Ctrl Pts',(-4.77596612414951,-0.552060840994624,
11.2768795166235));
#23234=CARTESIAN_POINT('Ctrl Pts',(-4.77596612414951,1.61522066995007,11.2768795166235));
#23235=CARTESIAN_POINT('Ctrl Pts',(-4.61532593596946,-0.552060840994624,
11.4029224160731));
#23236=CARTESIAN_POINT('Ctrl Pts',(-4.61532593596946,1.61522066995007,11.4029224160731));
#23237=CARTESIAN_POINT('Ctrl Pts',(-4.46255574628757,-0.552060840994624,
11.5373242211527));
#23238=CARTESIAN_POINT('Ctrl Pts',(-4.46255574628757,1.61522066995007,11.5373242211527));
#23239=CARTESIAN_POINT('Ctrl Pts',(-4.31893584999241,-0.552060840994624,
11.6776492463597));
#23240=CARTESIAN_POINT('Ctrl Pts',(-4.31893584999241,1.61522066995007,11.6776492463597));
#23241=CARTESIAN_POINT('Ctrl Pts',(-4.18369962429796,-0.552060840994624,
11.8183570873721));
#23242=CARTESIAN_POINT('Ctrl Pts',(-4.18369962429796,1.61522066995007,11.8183570873721));
#23243=CARTESIAN_POINT('Ctrl Pts',(-4.05395481372655,-0.552060840994624,
11.9514202619522));
#23244=CARTESIAN_POINT('Ctrl Pts',(-4.05395481372655,1.61522066995007,11.9514202619522));
#23245=CARTESIAN_POINT('Ctrl Pts',(-3.92533033057354,-0.552060840994624,
12.0684942936867));
#23246=CARTESIAN_POINT('Ctrl Pts',(-3.92533033057354,1.61522066995007,12.0684942936867));
#23247=CARTESIAN_POINT('Ctrl Pts',(-3.79241297762166,-0.552060840994624,
12.1626050652586));
#23248=CARTESIAN_POINT('Ctrl Pts',(-3.79241297762166,1.61522066995007,12.1626050652586));
#23249=CARTESIAN_POINT('Ctrl Pts',(-3.64927048315908,-0.552060840994624,
12.2301117722809));
#23250=CARTESIAN_POINT('Ctrl Pts',(-3.64927048315908,1.61522066995007,12.2301117722809));
#23251=CARTESIAN_POINT('Ctrl Pts',(-3.48993681214334,-0.552060840994624,
12.2723364229645));
#23252=CARTESIAN_POINT('Ctrl Pts',(-3.48993681214334,1.61522066995007,12.2723364229645));
#23253=CARTESIAN_POINT('Ctrl Pts',(-3.30884480305534,-0.552060840994624,
12.2938762651139));
#23254=CARTESIAN_POINT('Ctrl Pts',(-3.30884480305534,1.61522066995007,12.2938762651139));
#23255=CARTESIAN_POINT('Ctrl Pts',(-3.10127560868576,-0.552060840994624,
12.3010487961981));
#23256=CARTESIAN_POINT('Ctrl Pts',(-3.10127560868576,1.61522066995007,12.3010487961981));
#23257=CARTESIAN_POINT('Ctrl Pts',(-2.86376302967345,-0.552060840994624,
12.300400839059));
#23258=CARTESIAN_POINT('Ctrl Pts',(-2.86376302967345,1.61522066995007,12.300400839059));
#23259=CARTESIAN_POINT('Ctrl Pts',(-2.59461297443094,-0.552060840994624,
12.2969132923574));
#23260=CARTESIAN_POINT('Ctrl Pts',(-2.59461297443094,1.61522066995007,12.2969132923574));
#23261=CARTESIAN_POINT('Ctrl Pts',(-2.29394197380209,-0.552060840994624,
12.2935845551224));
#23262=CARTESIAN_POINT('Ctrl Pts',(-2.29394197380209,1.61522066995007,12.2935845551224));
#23263=CARTESIAN_POINT('Ctrl Pts',(-1.96338745719135,-0.552060840994624,
12.2919684497906));
#23264=CARTESIAN_POINT('Ctrl Pts',(-1.96338745719135,1.61522066995007,12.2919684497906));
#23265=CARTESIAN_POINT('Ctrl Pts',(-1.60591558979456,-0.552060840994624,
12.2924280531798));
#23266=CARTESIAN_POINT('Ctrl Pts',(-1.60591558979456,1.61522066995007,12.2924280531798));
#23267=CARTESIAN_POINT('Ctrl Pts',(-1.22558901314075,-0.552060840994624,
12.2945066442122));
#23268=CARTESIAN_POINT('Ctrl Pts',(-1.22558901314075,1.61522066995007,12.2945066442122));
#23269=CARTESIAN_POINT('Ctrl Pts',(-0.827351903312651,-0.552060840994624,
12.2972483292773));
#23270=CARTESIAN_POINT('Ctrl Pts',(-0.827351903312651,1.61522066995007,
12.2972483292773));
#23271=CARTESIAN_POINT('Ctrl Pts',(-0.498916532526571,-0.552060840994624,
12.299081889758));
#23272=CARTESIAN_POINT('Ctrl Pts',(-0.498916532526571,1.61522066995007,
12.299081889758));
#23273=CARTESIAN_POINT('Ctrl Pts',(-0.249771440080693,-0.552060840994624,
12.2998330708668));
#23274=CARTESIAN_POINT('Ctrl Pts',(-0.249771440080693,1.61522066995007,
12.2998330708668));
#23275=CARTESIAN_POINT('Ctrl Pts',(-0.0832571466935557,-0.552060840994624,
12.2999999999989));
#23276=CARTESIAN_POINT('Ctrl Pts',(-0.0832571466935557,1.61522066995007,
12.2999999999989));
#23277=CARTESIAN_POINT('Ctrl Pts',(0.,-0.552060840994624,12.3));
#23278=CARTESIAN_POINT('Ctrl Pts',(0.,1.61522066995007,12.3));
#23279=CARTESIAN_POINT('Ctrl Pts',(0.0832571466935396,-0.552060840994624,
12.3000000000011));
#23280=CARTESIAN_POINT('Ctrl Pts',(0.0832571466935396,1.61522066995007,
12.3000000000011));
#23281=CARTESIAN_POINT('Ctrl Pts',(0.24977144008061,-0.552060840994624,
12.2998330708736));
#23282=CARTESIAN_POINT('Ctrl Pts',(0.24977144008061,1.61522066995007,12.2998330708736));
#23283=CARTESIAN_POINT('Ctrl Pts',(0.498916532526534,-0.552060840994624,
12.2990818897713));
#23284=CARTESIAN_POINT('Ctrl Pts',(0.498916532526534,1.61522066995007,12.2990818897713));
#23285=CARTESIAN_POINT('Ctrl Pts',(0.827351903312438,-0.552060840994624,
12.2972483292974));
#23286=CARTESIAN_POINT('Ctrl Pts',(0.827351903312438,1.61522066995007,12.2972483292974));
#23287=CARTESIAN_POINT('Ctrl Pts',(1.22558901314046,-0.552060840994624,
12.2945066442369));
#23288=CARTESIAN_POINT('Ctrl Pts',(1.22558901314046,1.61522066995007,12.2945066442369));
#23289=CARTESIAN_POINT('Ctrl Pts',(1.60591558979418,-0.552060840994624,
12.2924280532047));
#23290=CARTESIAN_POINT('Ctrl Pts',(1.60591558979418,1.61522066995007,12.2924280532047));
#23291=CARTESIAN_POINT('Ctrl Pts',(1.96338745719096,-0.552060840994624,
12.291968449812));
#23292=CARTESIAN_POINT('Ctrl Pts',(1.96338745719096,1.61522066995007,12.291968449812));
#23293=CARTESIAN_POINT('Ctrl Pts',(2.29394197380175,-0.552060840994624,
12.2935845551378));
#23294=CARTESIAN_POINT('Ctrl Pts',(2.29394197380175,1.61522066995007,12.2935845551378));
#23295=CARTESIAN_POINT('Ctrl Pts',(2.59461297443069,-0.552060840994624,
12.2969132923658));
#23296=CARTESIAN_POINT('Ctrl Pts',(2.59461297443069,1.61522066995007,12.2969132923658));
#23297=CARTESIAN_POINT('Ctrl Pts',(2.86376302967335,-0.552060840994624,
12.3004008390612));
#23298=CARTESIAN_POINT('Ctrl Pts',(2.86376302967335,1.61522066995007,12.3004008390612));
#23299=CARTESIAN_POINT('Ctrl Pts',(3.10127560868576,-0.552060840994624,
12.3010487961961));
#23300=CARTESIAN_POINT('Ctrl Pts',(3.10127560868576,1.61522066995007,12.3010487961961));
#23301=CARTESIAN_POINT('Ctrl Pts',(3.30884480305537,-0.552060840994624,
12.2938762651102));
#23302=CARTESIAN_POINT('Ctrl Pts',(3.30884480305537,1.61522066995007,12.2938762651102));
#23303=CARTESIAN_POINT('Ctrl Pts',(3.48993681214337,-0.552060840994624,
12.2723364229612));
#23304=CARTESIAN_POINT('Ctrl Pts',(3.48993681214337,1.61522066995007,12.2723364229612));
#23305=CARTESIAN_POINT('Ctrl Pts',(3.64927048315907,-0.552060840994624,
12.2301117722792));
#23306=CARTESIAN_POINT('Ctrl Pts',(3.64927048315907,1.61522066995007,12.2301117722792));
#23307=CARTESIAN_POINT('Ctrl Pts',(3.79241297762162,-0.552060840994624,
12.1626050652587));
#23308=CARTESIAN_POINT('Ctrl Pts',(3.79241297762162,1.61522066995007,12.1626050652587));
#23309=CARTESIAN_POINT('Ctrl Pts',(3.90529123941674,-0.552060840994624,
12.0826827671148));
#23310=CARTESIAN_POINT('Ctrl Pts',(3.90529123941674,1.61522066995007,12.0826827671148));
#23311=CARTESIAN_POINT('Ctrl Pts',(3.98932418204563,-0.552060840994624,
12.0094836266392));
#23312=CARTESIAN_POINT('Ctrl Pts',(3.98932418204563,1.61522066995007,12.0094836266392));
#23313=CARTESIAN_POINT('Ctrl Pts',(4.04740991713241,-0.552060840994624,
11.9543581845679));
#23314=CARTESIAN_POINT('Ctrl Pts',(4.04740991713241,1.61522066995007,11.9543581845679));
#23315=CARTESIAN_POINT('Ctrl Pts',(4.07977092452996,-0.552060840994624,
11.9226494651812));
#23316=CARTESIAN_POINT('Ctrl Pts',(4.07977092452996,1.61522066995007,11.9226494651812));
#23317=CARTESIAN_POINT('Ctrl Pts',(4.08617023400024,-0.552060840994624,
11.9163435012344));
#23318=CARTESIAN_POINT('Ctrl Pts',(4.08617023400024,1.61522066995007,11.9163435012344));
#23319=CARTESIAN_POINT('Origin',(3.,0.,10.7));
#23320=CARTESIAN_POINT('',(2.7,0.,10.7));
#23321=CARTESIAN_POINT('Origin',(-3.,0.,11.7));
#23322=CARTESIAN_POINT('',(-3.36,0.,11.7));
#23323=CARTESIAN_POINT('Origin',(3.,0.,11.7));
#23324=CARTESIAN_POINT('',(2.64,0.,11.7));
#23325=CARTESIAN_POINT('Origin',(-3.,0.,10.7));
#23326=CARTESIAN_POINT('',(-3.3,0.,10.7));
#23327=CARTESIAN_POINT('Origin',(3.43968169690401,0.733833766068903,0.487016215536267));
#23328=CARTESIAN_POINT('Origin',(-4.33293714059227,0.0306667563398384,11.9026515720683));
#23329=CARTESIAN_POINT('Origin',(-3.43968169690379,0.733833766068911,0.487016215536247));
#85751=UNCERTAINTY_MEASURE_WITH_UNIT(LENGTH_MEASURE(0.001),#85790,
'DISTANCE_ACCURACY_VALUE',
'Maximum model space distance between geometric entities at asserted c
onnectivities');
#85769=UNCERTAINTY_MEASURE_WITH_UNIT(LENGTH_MEASURE(0.001),#85790,
'DISTANCE_ACCURACY_VALUE',
'Maximum model space distance between geometric entities at asserted c
onnectivities');
#85771=(
GEOMETRIC_REPRESENTATION_CONTEXT(3)
GLOBAL_UNCERTAINTY_ASSIGNED_CONTEXT((#85751))
GLOBAL_UNIT_ASSIGNED_CONTEXT((#85790,#85792,#85793))
REPRESENTATION_CONTEXT('','3D')
);
#85789=(
GEOMETRIC_REPRESENTATION_CONTEXT(3)
GLOBAL_UNCERTAINTY_ASSIGNED_CONTEXT((#85769))
GLOBAL_UNIT_ASSIGNED_CONTEXT((#85790,#85792,#85793))
REPRESENTATION_CONTEXT('','3D')
);
#85790=(
LENGTH_UNIT()
NAMED_UNIT(*)
SI_UNIT(.CENTI.,.METRE.)
);
#85792=(
NAMED_UNIT(*)
PLANE_ANGLE_UNIT()
SI_UNIT($,.RADIAN.)
);
#85793=(
NAMED_UNIT(*)
SI_UNIT($,.STERADIAN.)
SOLID_ANGLE_UNIT()
);
#85795=SHAPE_DEFINITION_REPRESENTATION(#85814,#85863);
#85814=PRODUCT_DEFINITION_SHAPE('',$,#85883);
#85863=SHAPE_REPRESENTATION('',(#10099),#85771);
#85881=PRODUCT_DEFINITION_CONTEXT('part definition',#85940,'design');
#85883=PRODUCT_DEFINITION('Clutch Release Fork Lever',
'Clutch Release Fork Lever',#85902,#85881);
#85902=PRODUCT_DEFINITION_FORMATION('',$,#85943);
#85940=APPLICATION_CONTEXT(
'Core Data for Automotive Mechanical Design Process');
#85941=PRODUCT_CONTEXT('part definition',#85940,'mechanical');
#85943=PRODUCT('Clutch Release Fork Lever','Clutch Release Fork Lever',
$,(#85941));
#85962=PRESENTATION_STYLE_ASSIGNMENT((#85980));
#85980=SURFACE_STYLE_USAGE(.BOTH.,#85998);
#85998=SURFACE_SIDE_STYLE('',(#86016));
#86016=SURFACE_STYLE_FILL_AREA(#86034);
#86034=FILL_AREA_STYLE('Opaque(112,115,119)',(#86052));
#86052=FILL_AREA_STYLE_COLOUR('Opaque(112,115,119)',#86070);
#86070=COLOUR_RGB('Opaque(112,115,119)', 0.66274510, 0.83137255, 0.94901961);
ENDSEC;
END-ISO-10303-21;
